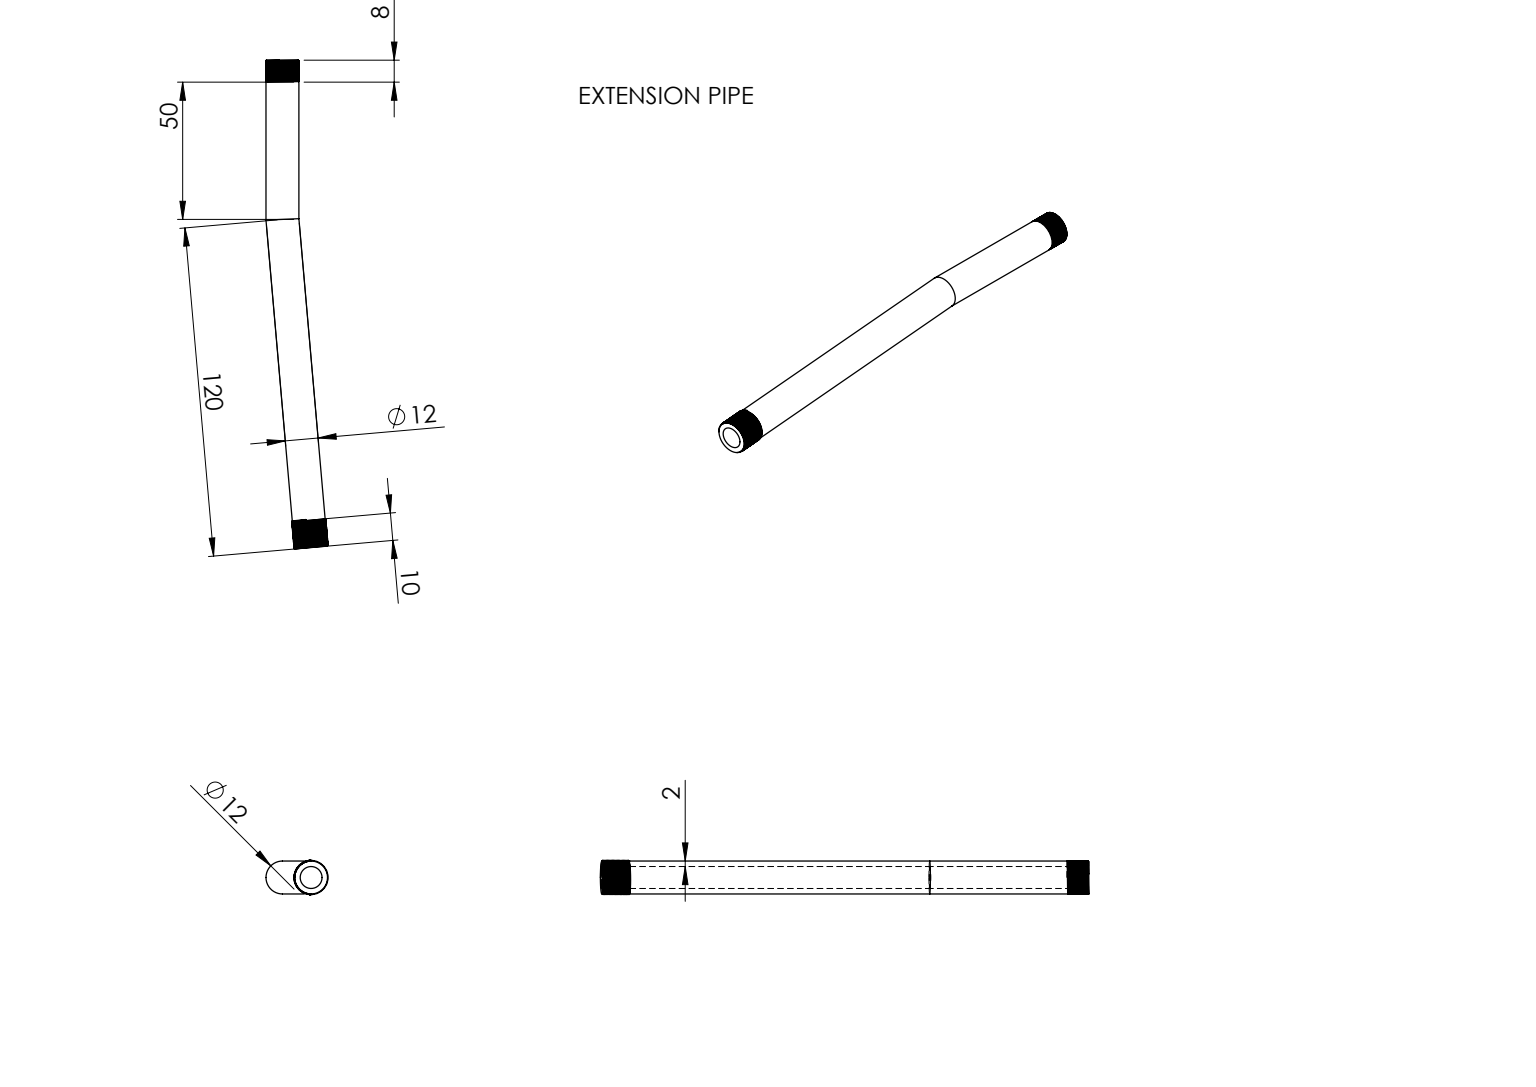
ISO-10303-21;
HEADER;
FILE_DESCRIPTION (('STEP AP214'),
    '1' );
FILE_NAME ('extension pipe.step',
    '2026-10-31T03:36:27',
    ( '' ),
    ( '' ),
    'SwSTEP 2.0',
    'SolidWorks 2026',
    '' );
FILE_SCHEMA (( 'AUTOMOTIVE_DESIGN' ));
ENDSEC;

DATA;
#1=CARTESIAN_POINT ( 'NONE',  ( 20.99999999999999645, 6.928203230275506996, -4.556249998770971033 ) ) ;
#4=CARTESIAN_POINT ( 'NONE',  ( 28.29077060037018043, 5.407089921784856479, 169.1523531505532674 ) ) ;
#11=CARTESIAN_POINT ( 'NONE',  ( 31.25278368747686741, 6.928203230275514990, 167.1898537967678351 ) ) ;
#19=CARTESIAN_POINT ( 'NONE',  ( 15.24356964375000167, -3.323476615752272600, -8.765624999385490668 ) ) ;
#24=CARTESIAN_POINT ( 'NONE',  ( 24.95044711734591658, -3.604726614523244610, 166.7907448923220954 ) ) ;
#32=CARTESIAN_POINT ( 'NONE',  ( 37.56819361912707222, 7.646167579472015790E-16, 167.7383919071516516 ) ) ;
#33=EDGE_LOOP ( 'NONE', ( #36990, #5292, #11130, #31770 ) ) ;
#35=CARTESIAN_POINT ( 'NONE',  ( 23.99999999999999645, 5.196152422706631135, -0.5437499987709648597 ) ) ;
#41=ORIENTED_EDGE ( 'NONE', *, *, #17124, .T. ) ;
#45=CARTESIAN_POINT ( 'NONE',  ( 31.45868912971818432, 0.000000000000000000, 169.5433637710095809 ) ) ;
#46=CARTESIAN_POINT ( 'NONE',  ( 37.19073179189800271, 7.347880794884117764E-16, 166.2186317273649934 ) ) ;
#58=CARTESIAN_POINT ( 'NONE',  ( 24.36378002397578868, 0.000000000000000000, 160.0851093307920223 ) ) ;
#59=CARTESIAN_POINT ( 'NONE',  ( 26.75643035624999655, 3.323476615752271712, -1.340624999385481075 ) ) ;
#64=ORIENTED_EDGE ( 'NONE', *, *, #31239, .F. ) ;
#66=CARTESIAN_POINT ( 'NONE',  ( 18.00000000000000355, -5.196152422706632912, -7.518749998770946519 ) ) ;
#67=CARTESIAN_POINT ( 'NONE',  ( 23.87821517812499650, 4.985214923628404904, -6.140624999385474680 ) ) ;
#75=CARTESIAN_POINT ( 'NONE',  ( 33.73804336749152810, 5.196152422706631135, 161.1753621882693892 ) ) ;
#80=CARTESIAN_POINT ( 'NONE',  ( 23.87821517812499650, 4.985214923628404904, -5.353124999385477700 ) ) ;
#88=EDGE_CURVE ( 'NONE', #32501, #27950, #21194, .T. ) ;
#91=CARTESIAN_POINT ( 'NONE',  ( 36.93903810116746911, 3.604726614523243278, 160.5471114303018680 ) ) ;
#103=ORIENTED_EDGE ( 'NONE', *, *, #10401, .F. ) ;
#104=CARTESIAN_POINT ( 'NONE',  ( 15.00000000000000000, 3.464101615137752166, -5.437500000000009770 ) ) ;
#106=DIRECTION ( 'NONE',  ( 0.9961946980917462113, 0.000000000000000000, -0.08715574274765118534 ) ) ;
#109=CARTESIAN_POINT ( 'NONE',  ( 31.18169728485186454, -7.209453229046475009, 166.3773324967488918 ) ) ;
#111=DIRECTION ( 'NONE',  ( 1.000000000000000000, 0.000000000000000000, 0.000000000000000000 ) ) ;
#114=ORIENTED_EDGE ( 'NONE', *, *, #15759, .T. ) ;
#119=CARTESIAN_POINT ( 'NONE',  ( 21.00000000000000000, 6.646953231504538984, -7.003124999385472726 ) ) ;
#122=CARTESIAN_POINT ( 'NONE',  ( 31.03707322417642800, -6.928203230275514990, 164.7242719189907803 ) ) ;
#123=CARTESIAN_POINT ( 'NONE',  ( 34.15965927292618431, 5.196152422706637353, 165.9944540390638679 ) ) ;
#126=CARTESIAN_POINT ( 'NONE',  ( 31.34102887711597774, 6.928203230275506996, 168.1985009298100522 ) ) ;
#131=DIRECTION ( 'NONE',  ( 0.9961946980917462113, 0.000000000000000000, -0.08715574274765118534 ) ) ;
#134=( BOUNDED_CURVE ( )  B_SPLINE_CURVE ( 2, ( #28363, #34243, #8285, #7031, #33171, #27292, #31580 ),
 .UNSPECIFIED., .F., .F. ) 
 B_SPLINE_CURVE_WITH_KNOTS ( ( 3, 2, 2, 3 ),
 ( 0.2826086956521732252, 0.2898550724637675158, 0.2971014492753617509, 0.3043478260869560414 ),
 .UNSPECIFIED. ) 
 CURVE ( )  GEOMETRIC_REPRESENTATION_ITEM ( )  RATIONAL_B_SPLINE_CURVE ( ( 1.000000000000012212, 0.8660254037844263841, 1.000000000000000000, 0.8660254037844387076, 1.000000000000000000, 0.8660254037844479225, 0.9999999999999907851 ) ) 
 REPRESENTATION_ITEM ( '' )  );
#139=CARTESIAN_POINT ( 'NONE',  ( 26.40304527788004663, 2.021082040740327379, -8.000000000000000000 ) ) ;
#140=CARTESIAN_POINT ( 'NONE',  ( 37.59924285248093412, -3.604726614523238837, 168.0932862683468443 ) ) ;
#141=CARTESIAN_POINT ( 'NONE',  ( 15.00000000000000178, -3.464101615137757051, -1.256249998770949228 ) ) ;
#150=CARTESIAN_POINT ( 'NONE',  ( 36.93740393099094632, -3.604726614523235284, 160.5284327797126025 ) ) ;
#151=CARTESIAN_POINT ( 'NONE',  ( 15.24356964374999990, 3.323476615752268604, -7.378124999385474503 ) ) ;
#153=CARTESIAN_POINT ( 'NONE',  ( 24.98313052087628350, 3.604726614523240613, 167.1643179041065252 ) ) ;
#154=CARTESIAN_POINT ( 'NONE',  ( 34.06814574304114984, -5.196152422706635576, 164.9484496060674985 ) ) ;
#161=EDGE_LOOP ( 'NONE', ( #20979, #30282, #30052, #34984, #7724, #7445, #15889, #35352 ) ) ;
#167=AXIS2_PLACEMENT_3D ( 'NONE', #4303, #33308, #24772 ) ;
#168=CARTESIAN_POINT ( 'NONE',  ( 26.75643035624999655, 3.323476615752271712, -3.140624999385464022 ) ) ;
#182=CARTESIAN_POINT ( 'NONE',  ( 21.00000000000016342, 4.000000000000002665, 50.00000000000000000 ) ) ;
#188=CARTESIAN_POINT ( 'NONE',  ( 30.87038786627866216, 6.928203230275506996, 162.8190495601146495 ) ) ;
#191=FACE_OUTER_BOUND ( 'NONE', #37346, .T. ) ;
#193=CARTESIAN_POINT ( 'NONE',  ( 15.24356964375000167, -3.323476615752272600, -1.453124999385472016 ) ) ;
#209=CARTESIAN_POINT ( 'NONE',  ( 19.00081571707366379, 5.492723647597353320, -10.23957781181608517 ) ) ;
#215=CARTESIAN_POINT ( 'NONE',  ( 25.06483902970220967, 0.000000000000000000, 168.0982504335675287 ) ) ;
#230=AXIS2_PLACEMENT_3D ( 'NONE', #7909, #4677, #5414 ) ;
#236=LINE ( 'NONE', #19612, #23826 ) ;
#242=CARTESIAN_POINT ( 'NONE',  ( 24.81477950914817754, 0.000000000000000000, 162.4454087870936121 ) ) ;
#243=ORIENTED_EDGE ( 'NONE', *, *, #7163, .F. ) ;
#249=CARTESIAN_POINT ( 'NONE',  ( 26.75643035624999655, 3.323476615752271712, -2.240624999385472549 ) ) ;
#252=ORIENTED_EDGE ( 'NONE', *, *, #5826, .F. ) ;
#255=CARTESIAN_POINT ( 'NONE',  ( 15.24356964374999990, 3.323476615752268604, -4.678124999385468108 ) ) ;
#260=EDGE_CURVE ( 'NONE', #23273, #19908, #35667, .T. ) ;
#264=CARTESIAN_POINT ( 'NONE',  ( 27.81970530529572372, -5.196152422706632912, 162.3707280659671994 ) ) ;
#268=CARTESIAN_POINT ( 'NONE',  ( 26.75643035624999655, 7.049594010296217766E-16, -4.978124999385491023 ) ) ;
#269=CARTESIAN_POINT ( 'NONE',  ( 24.00000000000000000, -5.196152422706629359, -1.650000000000012568 ) ) ;
#276=CARTESIAN_POINT ( 'NONE',  ( 33.95006120609467359, 5.407089921784862696, 162.2014130487530110 ) ) ;
#280=CARTESIAN_POINT ( 'NONE',  ( 24.71019261795870037, -3.464101615138094559, 161.2499751506078383 ) ) ;
#288=ORIENTED_EDGE ( 'NONE', *, *, #7515, .F. ) ;
#289=CARTESIAN_POINT ( 'NONE',  ( 15.00000000000000000, 3.464101615137752166, -3.637499999999994849 ) ) ;
#290=CARTESIAN_POINT ( 'NONE',  ( 34.18580599575048495, -5.196152422706635576, 166.2933124484913492 ) ) ;
#293=CARTESIAN_POINT ( 'NONE',  ( 34.37331128181295270, -5.407089921784855591, 167.0391835513610488 ) ) ;
#298=ORIENTED_EDGE ( 'NONE', *, *, #35567, .F. ) ;
#300=CARTESIAN_POINT ( 'NONE',  ( 24.61867908796596183, 0.000000000000000000, 160.2039707163872038 ) ) ;
#303=CARTESIAN_POINT ( 'NONE',  ( 15.24356964374999990, 3.323476615752268604, -6.028124999385455318 ) ) ;
#308=DIRECTION ( 'NONE',  ( 0.000000000000000000, 0.000000000000000000, 1.000000000000000000 ) ) ;
#309=CARTESIAN_POINT ( 'NONE',  ( 28.35571312319377313, 5.196152422706630247, 168.4973254592314618 ) ) ;
#314=( BOUNDED_CURVE ( )  B_SPLINE_CURVE ( 2, ( #13110, #21469, #7242, #4198, #30360, #25227, #30737 ),
 .UNSPECIFIED., .F., .F. ) 
 B_SPLINE_CURVE_WITH_KNOTS ( ( 3, 2, 2, 3 ),
 ( 0.5000000000000013323, 0.5072463768115947902, 0.5144927536231880261, 0.5217391304347814840 ),
 .UNSPECIFIED. ) 
 CURVE ( )  GEOMETRIC_REPRESENTATION_ITEM ( )  RATIONAL_B_SPLINE_CURVE ( ( 0.9999999999999753530, 0.8660254037844633546, 1.000000000000000000, 0.8660254037844387076, 1.000000000000000000, 0.8660254037844592467, 0.9999999999999794609 ) ) 
 REPRESENTATION_ITEM ( '' )  );
#323=CARTESIAN_POINT ( 'NONE',  ( 21.00000000000016342, -4.000000000000002665, 50.00000000000000000 ) ) ;
#324=CARTESIAN_POINT ( 'NONE',  ( 37.56655944895057075, 3.604726614523243278, 167.7197132565624713 ) ) ;
#325=CARTESIAN_POINT ( 'NONE',  ( 21.00000000000000000, 6.928203230275506996, -1.406249998770969123 ) ) ;
#330=FACE_OUTER_BOUND ( 'NONE', #17009, .T. ) ;
#335=EDGE_LOOP ( 'NONE', ( #19344, #12527, #16125, #26950 ) ) ;
#336=CARTESIAN_POINT ( 'NONE',  ( 24.36378002397578868, 0.000000000000000000, 160.0851093307920223 ) ) ;
#338=CARTESIAN_POINT ( 'NONE',  ( 26.75643035624999655, -3.323476615752267715, -8.053124999385453009 ) ) ;
#340=CARTESIAN_POINT ( 'NONE',  ( 37.21031035046954116, 7.646167579472024665E-16, 163.6477674281124450 ) ) ;
#341=CARTESIAN_POINT ( 'NONE',  ( 25.01414827068343172, -3.464101615137761048, 164.7242041589784947 ) ) ;
#348=ORIENTED_EDGE ( 'NONE', *, *, #4481, .T. ) ;
#352=EDGE_CURVE ( 'NONE', #13050, #23173, #13433, .T. ) ;
#354=CARTESIAN_POINT ( 'NONE',  ( 18.12178482187500350, -4.985214923628407568, -4.678124999385496530 ) ) ;
#377=ORIENTED_EDGE ( 'NONE', *, *, #18191, .T. ) ;
#378=CARTESIAN_POINT ( 'NONE',  ( 37.64336544724692146, -3.604726614523235284, 168.5976098342557918 ) ) ;
#380=CARTESIAN_POINT ( 'NONE',  ( 26.75643035624999655, 7.049594010296217766E-16, -1.265624999385456251 ) ) ;
#392=CARTESIAN_POINT ( 'NONE',  ( 18.12178482187499640, 4.985214923628404904, -8.428124999385472549 ) ) ;
#399=CARTESIAN_POINT ( 'NONE',  ( 28.05054758442196672, 5.407089921784862696, 166.4065915139379115 ) ) ;
#402=DIRECTION ( 'NONE',  ( 0.9961946980917462113, 0.000000000000000000, -0.08715574274765118534 ) ) ;
#407=VERTEX_POINT ( 'NONE', #11887 ) ;
#416=ORIENTED_EDGE ( 'NONE', *, *, #28626, .T. ) ;
#424=CARTESIAN_POINT ( 'NONE',  ( 25.44883753774445978, 3.464101615137752610, 169.6927252169354290 ) ) ;
#435=CARTESIAN_POINT ( 'NONE',  ( 30.67183618977810156, -7.209453229046475009, 160.5495935129122245 ) ) ;
#436=CARTESIAN_POINT ( 'NONE',  ( 26.75643035624999655, 7.049594010296217766E-16, -3.178124999385495641 ) ) ;
#441=CARTESIAN_POINT ( 'NONE',  ( 26.75643035624999655, -3.323476615752267271, -6.253124999385469174 ) ) ;
#448=CARTESIAN_POINT ( 'NONE',  ( 24.82458453031440726, 0.000000000000000000, 162.5574806918533000 ) ) ;
#452=CARTESIAN_POINT ( 'NONE',  ( 23.87821517812499650, 4.985214923628404904, -6.703124999385495997 ) ) ;
#460=CARTESIAN_POINT ( 'NONE',  ( 20.99999999999999645, 6.928203230275506996, -5.906249998770958243 ) ) ;
#461=CARTESIAN_POINT ( 'NONE',  ( 33.74088742350031822, -5.407089921784861808, 159.8105457733328478 ) ) ;
#470=CARTESIAN_POINT ( 'NONE',  ( 37.03711979530484655, 3.464101615138000856, 164.4628385719782955 ) ) ;
#474=CARTESIAN_POINT ( 'NONE',  ( 18.00000000000000000, 5.196152422706630247, -8.174999999999988276 ) ) ;
#476=CYLINDRICAL_SURFACE ( 'NONE', #30001, 5.999999999999994671 ) ;
#479=CARTESIAN_POINT ( 'NONE',  ( 28.14696362483655889, -5.407089921784859143, 167.5086318987019069 ) ) ;
#484=AXIS2_PLACEMENT_3D ( 'NONE', #11652, #17544, #9193 ) ;
#486=DIRECTION ( 'NONE',  ( 0.000000000000000000, 0.000000000000000000, 1.000000000000000000 ) ) ;
#487=CARTESIAN_POINT ( 'NONE',  ( 26.99999999999999645, 7.347880794884117764E-16, -3.318749998770964549 ) ) ;
#489=CARTESIAN_POINT ( 'NONE',  ( 23.87821517812500005, -4.985214923628404016, -6.290624999385458160 ) ) ;
#492=CARTESIAN_POINT ( 'NONE',  ( 36.99463137071579411, 7.347880794884117764E-16, 163.9771936566585566 ) ) ;
#496=CARTESIAN_POINT ( 'NONE',  ( 25.41615413421409642, -3.464101615137757051, 169.3191522051509992 ) ) ;
#508=CARTESIAN_POINT ( 'NONE',  ( 37.44889919624123564, 3.604726614523243278, 166.3748504141385922 ) ) ;
#509=CARTESIAN_POINT ( 'NONE',  ( 15.00000000000000000, 3.464101615137752166, -2.231249998770934884 ) ) ;
#517=CARTESIAN_POINT ( 'NONE',  ( 24.78536444607796341, 0.000000000000000000, 162.1091930777120069 ) ) ;
#518=ORIENTED_EDGE ( 'NONE', *, *, #17390, .F. ) ;
#519=CARTESIAN_POINT ( 'NONE',  ( 30.61300606342343755, 7.209453229046475009, 159.8771620917002565 ) ) ;
#520=CARTESIAN_POINT ( 'NONE',  ( 26.75643035624999655, 7.049594010296217766E-16, -9.815624999385457627 ) ) ;
#522=CARTESIAN_POINT ( 'NONE',  ( 37.33123894353190764, 3.604726614523243278, 165.0299875717147131 ) ) ;
#523=CARTESIAN_POINT ( 'NONE',  ( 30.89980292934887629, 6.928203230275514990, 163.1552652694962546 ) ) ;
#534=EDGE_CURVE ( 'NONE', #28874, #27232, #3235, .T. ) ;
#535=CARTESIAN_POINT ( 'NONE',  ( 18.12178482187499640, 4.985214923628404904, -4.828124999385480010 ) ) ;
#544=CARTESIAN_POINT ( 'NONE',  ( 31.20375858228842603, -6.928203230275506996, 166.6294942803155550 ) ) ;
#550=CARTESIAN_POINT ( 'NONE',  ( 30.88754665307854097, 7.209453229046475009, 163.0151753906892793 ) ) ;
#554=CARTESIAN_POINT ( 'NONE',  ( 15.00000000000000000, 0.000000000000000000, 0.000000000000000000 ) ) ;
#562=CARTESIAN_POINT ( 'NONE',  ( 37.52570519453759346, -3.604726614523235284, 167.2527469918319412 ) ) ;
#565=CARTESIAN_POINT ( 'NONE',  ( 26.99999999999999645, 7.347880794884117764E-16, -4.668749998770954868 ) ) ;
#574=CARTESIAN_POINT ( 'NONE',  ( 21.00000000000000000, 6.646953231504538984, -1.603124999385459937 ) ) ;
#582=CARTESIAN_POINT ( 'NONE',  ( 27.85444716323975101, 5.407089921784862696, 164.1651534432314747 ) ) ;
#585=CARTESIAN_POINT ( 'NONE',  ( 15.00000000000001954, 11.99999999999999822, 50.26196565745151190 ) ) ;
#588=CARTESIAN_POINT ( 'NONE',  ( 31.04687824534265417, -6.928203230275506996, 164.8363438237504113 ) ) ;
#589=CARTESIAN_POINT ( 'NONE',  ( 27.99008328789078703, -5.407089921784859143, 165.7154814421367348 ) ) ;
#590=VERTEX_POINT ( 'NONE', #13390 ) ;
#594=EDGE_CURVE ( 'NONE', #25471, #14391, #18768, .T. ) ;
#596=LINE ( 'NONE', #9710, #21812 ) ;
#608=CARTESIAN_POINT ( 'NONE',  ( 20.99999999999999645, 0.000000000000000000, -8.000000000000000000 ) ) ;
#611=CARTESIAN_POINT ( 'NONE',  ( 26.99999999999999645, 7.347880794884117764E-16, -4.668749998770954868 ) ) ;
#617=CARTESIAN_POINT ( 'NONE',  ( 29.49486714975617474, 6.148716665048038266, 159.5363409456820136 ) ) ;
#619=CARTESIAN_POINT ( 'NONE',  ( 26.75643035624999655, -3.323476615752267715, -2.315624999385466509 ) ) ;
#623=VECTOR ( 'NONE', #32641, 1000.000000000000000 ) ;
#624=ORIENTED_EDGE ( 'NONE', *, *, #36236, .T. ) ;
#625=CARTESIAN_POINT ( 'NONE',  ( 26.75643035624999655, -3.323476615752267271, -4.003124999385458516 ) ) ;
#626=CARTESIAN_POINT ( 'NONE',  ( 24.65463083184878101, 3.464101615137419543, 160.6149010293500510 ) ) ;
#629=EDGE_CURVE ( 'NONE', #9403, #23945, #16100, .T. ) ;
#633=CARTESIAN_POINT ( 'NONE',  ( 36.68087069682425039, 7.347880794884117764E-16, 160.3908927435282692 ) ) ;
#638=CARTESIAN_POINT ( 'NONE',  ( 15.24356964374999990, 0.000000000000000000, -6.553124999385484983 ) ) ;
#646=CARTESIAN_POINT ( 'NONE',  ( 36.81810950810510974, 7.646167579472024665E-16, 159.1648912866995715 ) ) ;
#658=CARTESIAN_POINT ( 'NONE',  ( 18.00000000000000355, -5.196152422706632912, -8.025000000000003908 ) ) ;
#662=CARTESIAN_POINT ( 'NONE',  ( 37.41458162253433528, 3.604726614523238837, 165.9825987517649253 ) ) ;
#664=EDGE_CURVE ( 'NONE', #25295, #10376, #15092, .T. ) ;
#671=CARTESIAN_POINT ( 'NONE',  ( 15.00000000000063771, -3.464101615138124757, -3.506249998770952558 ) ) ;
#673=CARTESIAN_POINT ( 'NONE',  ( 21.00000000000000000, 6.646953231504538984, -5.203124999385457805 ) ) ;
#678=CARTESIAN_POINT ( 'NONE',  ( 28.18902776508177510, 5.196152422706636465, 166.5921030979066586 ) ) ;
#681=FACE_OUTER_BOUND ( 'NONE', #22092, .T. ) ;
#682=CARTESIAN_POINT ( 'NONE',  ( 28.43415329166666083, 5.196152422706630247, 169.3939006875140194 ) ) ;
#687=CARTESIAN_POINT ( 'NONE',  ( 20.99999999999999645, -6.646953231504538984, -0.5906249993854775227 ) ) ;
#694=CARTESIAN_POINT ( 'NONE',  ( 37.06326651802246630, 7.347880794884125653E-16, 164.7616969801814548 ) ) ;
#695=CARTESIAN_POINT ( 'NONE',  ( 28.06362094583411704, -5.407089921784865361, 166.5560207186516664 ) ) ;
#703=CARTESIAN_POINT ( 'NONE',  ( 36.95867962683190910, 3.464101615138031054, 163.5662633436957663 ) ) ;
#706=CARTESIAN_POINT ( 'NONE',  ( 27.54558899987776144, 5.407089921784856479, 160.6348884818688418 ) ) ;
#708=CARTESIAN_POINT ( 'NONE',  ( 21.00000000000000000, 6.928203230275506996, -0.5624999999999866773 ) ) ;
#710=CARTESIAN_POINT ( 'NONE',  ( 30.98069435314010178, -7.209453229046482114, 164.0798584742748290 ) ) ;
#711=CARTESIAN_POINT ( 'NONE',  ( 31.03707322417642800, -6.928203230275514990, 164.7242719189907518 ) ) ;
#712=CARTESIAN_POINT ( 'NONE',  ( 25.17756528844239483, 0.000000000000000000, 166.5920692191248804 ) ) ;
#721=CARTESIAN_POINT ( 'NONE',  ( 26.75643035624999655, 7.049594010296217766E-16, -4.528124999385485516 ) ) ;
#733=( BOUNDED_CURVE ( )  B_SPLINE_CURVE ( 2, ( #32456, #15221, #12753, #23751, #29425, #29803, #21299 ),
 .UNSPECIFIED., .F., .F. ) 
 B_SPLINE_CURVE_WITH_KNOTS ( ( 3, 2, 2, 3 ),
 ( 0.6956521739130425708, 0.7028985507246365838, 0.7101449275362307079, 0.7173913043478246099 ),
 .UNSPECIFIED. ) 
 CURVE ( )  GEOMETRIC_REPRESENTATION_ITEM ( )  RATIONAL_B_SPLINE_CURVE ( ( 1.000000000000016431, 0.8660254037844222763, 1.000000000000000000, 0.8660254037844387076, 1.000000000000000000, 0.8660254037844653530, 0.9999999999999733546 ) ) 
 REPRESENTATION_ITEM ( '' )  );
#738=CARTESIAN_POINT ( 'NONE',  ( 30.90715669519676467, -7.209453229046475009, 163.2393191977598974 ) ) ;
#750=ORIENTED_EDGE ( 'NONE', *, *, #22577, .F. ) ;
#751=EDGE_CURVE ( 'NONE', #37490, #27706, #21564, .T. ) ;
#752=CARTESIAN_POINT ( 'NONE',  ( 28.14696362483655889, -5.407089921784859143, 167.5086318987019069 ) ) ;
#753=CARTESIAN_POINT ( 'NONE',  ( 21.00000000000000000, -6.646953231504538984, -3.628124999385489158 ) ) ;
#755=CARTESIAN_POINT ( 'NONE',  ( 15.02283181144952628, 7.347880794884122694E-16, 50.52293445648592751 ) ) ;
#757=CARTESIAN_POINT ( 'NONE',  ( 20.99999999999999645, -6.928203230275506996, -7.481249998770959309 ) ) ;
#766=CARTESIAN_POINT ( 'NONE',  ( 23.87821517812500005, -4.985214923628404016, -2.240624999385460114 ) ) ;
#768=CARTESIAN_POINT ( 'NONE',  ( 15.00000000000000178, -3.464101615137757051, -6.206249998770966059 ) ) ;
#769=DIRECTION ( 'NONE',  ( 0.000000000000000000, 0.000000000000000000, 1.000000000000000000 ) ) ;
#772=VECTOR ( 'NONE', #3527, 1000.000000000000000 ) ;
#773=ORIENTED_EDGE ( 'NONE', *, *, #629, .F. ) ;
#775=CARTESIAN_POINT ( 'NONE',  ( 24.70858993122118363, 3.604726614523240613, 164.0263046051175024 ) ) ;
#782=CARTESIAN_POINT ( 'NONE',  ( 25.03378979634835488, -3.604726614523240613, 167.7433560723723076 ) ) ;
#795=( BOUNDED_CURVE ( )  B_SPLINE_CURVE ( 2, ( #34956, #23784, #32113, #6149, #3492, #15063, #12212 ),
 .UNSPECIFIED., .F., .F. ) 
 B_SPLINE_CURVE_WITH_KNOTS ( ( 3, 2, 2, 3 ),
 ( 0.02173913043478289606, 0.02898550724637719705, 0.03623188405797149458, 0.04347826086956579211 ),
 .UNSPECIFIED. ) 
 CURVE ( )  GEOMETRIC_REPRESENTATION_ITEM ( )  RATIONAL_B_SPLINE_CURVE ( ( 0.9999999999999946709, 0.8660254037844440367, 1.000000000000000000, 0.8660254037844387076, 1.000000000000000000, 0.8660254037844280495, 1.000000000000010658 ) ) 
 REPRESENTATION_ITEM ( '' )  );
#802=CARTESIAN_POINT ( 'NONE',  ( 21.00000000000000355, 0.000000000000000000, 50.00000000000001421 ) ) ;
#804=CARTESIAN_POINT ( 'NONE',  ( 26.99999999999999289, 0.000000000000000000, 49.73803434254939759 ) ) ;
#805=VERTEX_POINT ( 'NONE', #21931 ) ;
#810=CARTESIAN_POINT ( 'NONE',  ( 21.00000000000000000, 6.646953231504538984, -5.765624999385476457 ) ) ;
#816=CARTESIAN_POINT ( 'NONE',  ( 18.12178482187500350, -4.985214923628407568, -5.915624999385471483 ) ) ;
#826=CARTESIAN_POINT ( 'NONE',  ( 30.69389748721465949, -6.928203230275506996, 160.8017552964788592 ) ) ;
#830=CARTESIAN_POINT ( 'NONE',  ( 26.75643035624999655, 3.323476615752271268, -6.290624999385498128 ) ) ;
#834=LINE ( 'NONE', #16009, #19275 ) ;
#838=CARTESIAN_POINT ( 'NONE',  ( 33.81932759197320593, -5.407089921784861808, 160.7071210016154055 ) ) ;
#845=CARTESIAN_POINT ( 'NONE',  ( 25.05990503573306682, 0.000000000000000000, 165.2472063767010013 ) ) ;
#849=ORIENTED_EDGE ( 'NONE', *, *, #1576, .T. ) ;
#850=CARTESIAN_POINT ( 'NONE',  ( 26.99999999999999645, 3.464101615137755275, -7.387499999999980638 ) ) ;
#855=CARTESIAN_POINT ( 'NONE',  ( 31.16208724273364084, 7.209453229046475009, 166.1531886896782737 ) ) ;
#860=ORIENTED_EDGE ( 'NONE', *, *, #32619, .T. ) ;
#865=CARTESIAN_POINT ( 'NONE',  ( 15.24356964374999990, 3.323476615752268604, -6.478124999385451055 ) ) ;
#870=( BOUNDED_CURVE ( )  B_SPLINE_CURVE ( 2, ( #20831, #29529, #6222, #18875, #33264, #1604, #17986 ),
 .UNSPECIFIED., .F., .F. ) 
 B_SPLINE_CURVE_WITH_KNOTS ( ( 3, 2, 2, 3 ),
 ( 0.6304347826086960094, 0.6376811594202902445, 0.6449275362318845906, 0.6521739130434789367 ),
 .UNSPECIFIED. ) 
 CURVE ( )  GEOMETRIC_REPRESENTATION_ITEM ( )  RATIONAL_B_SPLINE_CURVE ( ( 0.9999999999999938938, 0.8660254037844448138, 1.000000000000000000, 0.8660254037844387076, 1.000000000000000000, 0.8660254037844263841, 1.000000000000012212 ) ) 
 REPRESENTATION_ITEM ( '' )  );
#873=CARTESIAN_POINT ( 'NONE',  ( 31.36063891923419789, -6.928203230275506996, 168.4226447368806987 ) ) ;
#886=CARTESIAN_POINT ( 'NONE',  ( 28.14206111430700474, -5.407089921784865361, 167.4525959469342524 ) ) ;
#899=CARTESIAN_POINT ( 'NONE',  ( 33.71964321120555752, 5.407089921784857367, 159.5677233156729642 ) ) ;
#900=CARTESIAN_POINT ( 'NONE',  ( 26.99999999999999645, 3.464101615137755275, -0.6375000000000126121 ) ) ;
#902=CARTESIAN_POINT ( 'NONE',  ( 24.90795869275643426, 0.000000000000000000, 166.3050999770023850 ) ) ;
#903=UNCERTAINTY_MEASURE_WITH_UNIT (LENGTH_MEASURE( 1.000000000000000082E-05 ), #4566, 'distance_accuracy_value', 'NONE');
#904=CARTESIAN_POINT ( 'NONE',  ( 36.98482634954957859, 7.347880794884125653E-16, 163.8651217518988688 ) ) ;
#905=DIRECTION ( 'NONE',  ( 1.000000000000000000, 0.000000000000000000, 0.000000000000000000 ) ) ;
#908=EDGE_CURVE ( 'NONE', #17354, #5563, #28159, .T. ) ;
#911=ORIENTED_EDGE ( 'NONE', *, *, #11960, .F. ) ;
#917=CARTESIAN_POINT ( 'NONE',  ( 21.00000000000000000, 6.646953231504538984, -3.515624999385498217 ) ) ;
#927=FACE_BOUND ( 'NONE', #31912, .T. ) ;
#930=CARTESIAN_POINT ( 'NONE',  ( 37.29692136982500728, 3.604726614523238837, 164.6377359093410746 ) ) ;
#934=PLANE ( 'NONE',  #1221 ) ;
#941=VERTEX_POINT ( 'NONE', #5036 ) ;
#942=CARTESIAN_POINT ( 'NONE',  ( 31.22091736908830839, -7.209453229046475009, 166.8256201108902133 ) ) ;
#943=CARTESIAN_POINT ( 'NONE',  ( 23.87821517812500005, -4.985214923628404016, -2.690624999385465621 ) ) ;
#951=ORIENTED_EDGE ( 'NONE', *, *, #25354, .F. ) ;
#952=VERTEX_POINT ( 'NONE', #16800 ) ;
#955=CARTESIAN_POINT ( 'NONE',  ( 26.75643035624999655, 3.323476615752271712, -2.128124999385482052 ) ) ;
#957=CARTESIAN_POINT ( 'NONE',  ( 26.99999999999999645, 7.347880794884117764E-16, -7.818749998770941012 ) ) ;
#961=ORIENTED_EDGE ( 'NONE', *, *, #8896, .T. ) ;
#964=CARTESIAN_POINT ( 'NONE',  ( 24.75434669616370087, -3.604726614523244610, 164.5493068216156871 ) ) ;
#971=CARTESIAN_POINT ( 'NONE',  ( 31.20130732697009535, 7.209453229046475009, 166.6014763038195383 ) ) ;
#972=VERTEX_POINT ( 'NONE', #11471 ) ;
#977=DIRECTION ( 'NONE',  ( 0.000000000000000000, 0.000000000000000000, 1.000000000000000000 ) ) ;
#986=CARTESIAN_POINT ( 'NONE',  ( 23.99999999999999645, 5.196152422706631135, -1.500000000000001332 ) ) ;
#992=CARTESIAN_POINT ( 'NONE',  ( 25.05663669537974414, 3.464101615137583856, 165.2098490755226123 ) ) ;
#998=CARTESIAN_POINT ( 'NONE',  ( 15.24356964375000167, -3.323476615752272600, -4.715624999385497063 ) ) ;
#1002=CARTESIAN_POINT ( 'NONE',  ( 20.99999999999999645, -6.646953231504538984, -6.778124999385457983 ) ) ;
#1004=VECTOR ( 'NONE', #14540, 1000.000000000000000 ) ;
#1006=EDGE_CURVE ( 'NONE', #5916, #35535, #23839, .T. ) ;
#1009=CARTESIAN_POINT ( 'NONE',  ( 33.60730975337005333, -5.196152422706629359, 159.6810701411317552 ) ) ;
#1014=CARTESIAN_POINT ( 'NONE',  ( 20.99999999999999645, -6.646953231504538984, -7.340624999385477523 ) ) ;
#1015=CARTESIAN_POINT ( 'NONE',  ( 26.99999999999999645, 7.347880794884117764E-16, -2.475000000000004974 ) ) ;
#1019=CARTESIAN_POINT ( 'NONE',  ( 25.48152094116770883, 0.000000000000000000, 170.0662982274954800 ) ) ;
#1024=CARTESIAN_POINT ( 'NONE',  ( 36.85732959234155004, 7.646167579472024665E-16, 159.6131789008408646 ) ) ;
#1032=CARTESIAN_POINT ( 'NONE',  ( 24.99999999999999289, 0.000000000000000000, -8.000000000000000000 ) ) ;
#1038=CARTESIAN_POINT ( 'NONE',  ( 26.99999999999999645, 7.347880794884117764E-16, -6.074999999999997513 ) ) ;
#1042=CARTESIAN_POINT ( 'NONE',  ( 27.82012958953286130, 5.407089921784856479, 163.7729017808578362 ) ) ;
#1043=CARTESIAN_POINT ( 'NONE',  ( 28.42434827050043467, 5.196152422706636465, 169.2818287827543600 ) ) ;
#1051=CARTESIAN_POINT ( 'NONE',  ( 26.75643035624999655, -3.323476615752267715, -7.603124999385488358 ) ) ;
#1058=CARTESIAN_POINT ( 'NONE',  ( 31.24297866652486633, -6.928203230275506996, 167.0777818944568480 ) ) ;
#1070=EDGE_CURVE ( 'NONE', #30479, #30148, #16319, .T. ) ;
#1072=( BOUNDED_CURVE ( )  B_SPLINE_CURVE ( 2, ( #10156, #21731, #27592, #6752, #33281, #24192, #32900 ),
 .UNSPECIFIED., .F., .F. ) 
 B_SPLINE_CURVE_WITH_KNOTS ( ( 3, 2, 2, 3 ),
 ( 0.7173913043478248319, 0.7246376811594191780, 0.7318840579710134131, 0.7391304347826076482 ),
 .UNSPECIFIED. ) 
 CURVE ( )  GEOMETRIC_REPRESENTATION_ITEM ( )  RATIONAL_B_SPLINE_CURVE ( ( 1.000000000000022649, 0.8660254037844161701, 1.000000000000000000, 0.8660254037844387076, 1.000000000000000000, 0.8660254037844571373, 0.9999999999999815703 ) ) 
 REPRESENTATION_ITEM ( '' )  );
#1076=CARTESIAN_POINT ( 'NONE',  ( 37.44236251553515871, -3.604726614523238837, 166.3001358117817006 ) ) ;
#1085=CARTESIAN_POINT ( 'NONE',  ( 15.00000000000000355, 7.347880794884112834E-16, -8.000000000000000000 ) ) ;
#1089=CARTESIAN_POINT ( 'NONE',  ( 24.39973176785919051, 3.604726614523236616, 160.4960396437548695 ) ) ;
#1090=CARTESIAN_POINT ( 'NONE',  ( 21.00000000000000000, -6.646953231504538984, -9.478124999385466154 ) ) ;
#1091=CARTESIAN_POINT ( 'NONE',  ( 25.40961745350799461, 3.464101615137737067, 169.2444376027941360 ) ) ;
#1092=CARTESIAN_POINT ( 'NONE',  ( 24.79356678040014117, -3.604726614523244610, 164.9975944357569517 ) ) ;
#1093=CARTESIAN_POINT ( 'NONE',  ( 36.86389775648721212, -3.464101615137755275, 162.4829016082965438 ) ) ;
#1105=CARTESIAN_POINT ( 'NONE',  ( 15.24356964374999990, 0.000000000000000000, -6.553124999385484983 ) ) ;
#1116=LINE ( 'NONE', #12682, #17619 ) ;
#1120=CARTESIAN_POINT ( 'NONE',  ( 31.08364707426076023, 7.209453229046475009, 165.2566134613956876 ) ) ;
#1130=ORIENTED_EDGE ( 'NONE', *, *, #27910, .F. ) ;
#1131=CARTESIAN_POINT ( 'NONE',  ( 34.37331128181295270, -5.407089921784855591, 167.0391835513610488 ) ) ;
#1132=CARTESIAN_POINT ( 'NONE',  ( 26.75643035624999655, -3.323476615752267715, -3.103124999385467486 ) ) ;
#1133=CARTESIAN_POINT ( 'NONE',  ( 26.78555467025737258, 0.1019468494213565390, -8.000000000000003553 ) ) ;
#1143=CARTESIAN_POINT ( 'NONE',  ( 21.00000000000000000, -6.646953231504538984, -2.728124999385465266 ) ) ;
#1145=EDGE_CURVE ( 'NONE', #13208, #28137, #27709, .T. ) ;
#1146=CARTESIAN_POINT ( 'NONE',  ( 15.00000000000000178, -3.464101615137757051, -8.456249998770944742 ) ) ;
#1153=CARTESIAN_POINT ( 'NONE',  ( 24.74781001545762393, 3.604726614523240613, 164.4745922192587670 ) ) ;
#1158=DIRECTION ( 'NONE',  ( 0.000000000000000000, 0.000000000000000000, 1.000000000000000000 ) ) ;
#1161=CARTESIAN_POINT ( 'NONE',  ( 37.41131328218130392, 7.646167579472015790E-16, 165.9452414505865079 ) ) ;
#1163=CARTESIAN_POINT ( 'NONE',  ( 31.31161381383153142, -6.928203230275514990, 167.8622852179797462 ) ) ;
#1170=VERTEX_POINT ( 'NONE', #12026 ) ;
#1171=( LENGTH_UNIT ( ) NAMED_UNIT ( * ) SI_UNIT ( .MILLI., .METRE. ) );
#1175=CARTESIAN_POINT ( 'NONE',  ( 15.00000000000000000, 0.000000000000000000, -1.349999999999990097 ) ) ;
#1178=CARTESIAN_POINT ( 'NONE',  ( 15.60291623300155095, 2.331604889245508350, -7.999999999999992895 ) ) ;
#1186=CARTESIAN_POINT ( 'NONE',  ( 15.24356964375000167, -3.323476615752272600, -3.815624999385473615 ) ) ;
#1189=CARTESIAN_POINT ( 'NONE',  ( 36.99136303036318196, -3.464101615137506140, 163.9398363554800540 ) ) ;
#1196=CARTESIAN_POINT ( 'NONE',  ( 27.61053152270135058, 5.196152422706630247, 159.9798607905470362 ) ) ;
#1200=CARTESIAN_POINT ( 'NONE',  ( 23.87821517812500005, -4.985214923628404016, -5.953124999385495109 ) ) ;
#1214=CARTESIAN_POINT ( 'NONE',  ( 26.97716818855048260, 0.000000000000000000, 49.47706554351410801 ) ) ;
#1221=AXIS2_PLACEMENT_3D ( 'NONE', #29172, #18014, #26333 ) ;
#1223=CARTESIAN_POINT ( 'NONE',  ( 26.99999999999999289, 0.000000000000000000, -8.000000000000000000 ) ) ;
#1226=CARTESIAN_POINT ( 'NONE',  ( 31.04442699002431993, 7.209453229046475009, 164.8083258472544230 ) ) ;
#1229=VERTEX_POINT ( 'NONE', #1019 ) ;
#1234=DIRECTION ( 'NONE',  ( 0.000000000000000000, 0.000000000000000000, 1.000000000000000000 ) ) ;
#1236=CARTESIAN_POINT ( 'NONE',  ( 25.22171936664797798, 0.000000000000000000, 169.8914008901326724 ) ) ;
#1237=CARTESIAN_POINT ( 'NONE',  ( 21.00000000000000000, 6.646953231504538984, -9.253124999385450522 ) ) ;
#1238=VECTOR ( 'NONE', #13008, 1000.000000000000000 ) ;
#1246=CARTESIAN_POINT ( 'NONE',  ( 31.30180879287953388, 6.928203230275506996, 167.7502133156687876 ) ) ;
#1252=CARTESIAN_POINT ( 'NONE',  ( 15.24356964374999990, 0.000000000000000000, -0.2531249993854844949 ) ) ;
#1260=CARTESIAN_POINT ( 'NONE',  ( 28.02440086159767674, -5.407089921784865361, 166.1077331045103733 ) ) ;
#1269=CARTESIAN_POINT ( 'NONE',  ( 18.00000000000000355, -5.196152422706632912, -7.968749998770952025 ) ) ;
#1275=CARTESIAN_POINT ( 'NONE',  ( 21.00000000000000000, 6.928203230275506996, -0.1124999999999909128 ) ) ;
#1277=CARTESIAN_POINT ( 'NONE',  ( 30.88264414254899393, 7.209453229046482114, 162.9591394389215964 ) ) ;
#1278=CARTESIAN_POINT ( 'NONE',  ( 24.77882776526477571, -3.464101615137761048, 162.0344784741307933 ) ) ;
#1283=ORIENTED_EDGE ( 'NONE', *, *, #15614, .T. ) ;
#1285=ORIENTED_EDGE ( 'NONE', *, *, #5231, .T. ) ;
#1290=CARTESIAN_POINT ( 'NONE',  ( 15.24356964374999990, 0.000000000000000000, -5.653124999385472194 ) ) ;
#1304=EDGE_CURVE ( 'NONE', #17372, #23833, #795, .T. ) ;
#1306=CARTESIAN_POINT ( 'NONE',  ( 37.13677269252619340, 7.646167579472015790E-16, 162.8072281515975135 ) ) ;
#1309=CARTESIAN_POINT ( 'NONE',  ( 14.99999999999945111, -3.464101615137439083, -0.8625000000000012657 ) ) ;
#1311=CARTESIAN_POINT ( 'NONE',  ( 18.00000000000000355, -5.196152422706632912, -5.718749998770950249 ) ) ;
#1313=CARTESIAN_POINT ( 'NONE',  ( 18.00000000000000355, -5.196152422706632912, -4.368749998770960374 ) ) ;
#1319=CARTESIAN_POINT ( 'NONE',  ( 28.21233043189729273, 5.407089921784856479, 168.2557779222707097 ) ) ;
#1320=CARTESIAN_POINT ( 'NONE',  ( 18.12178482187500350, -4.985214923628407568, -3.665624999385469707 ) ) ;
#1324=CARTESIAN_POINT ( 'NONE',  ( 34.27731952563551232, 5.196152422706637353, 167.3393168814877185 ) ) ;
#1335=CARTESIAN_POINT ( 'NONE',  ( 18.12178482187499640, 4.985214923628404904, -0.6656249993854668201 ) ) ;
#1337=CARTESIAN_POINT ( 'NONE',  ( 26.75643035624999655, 7.049594010296217766E-16, -0.4781249993854874702 ) ) ;
#1343=CARTESIAN_POINT ( 'NONE',  ( 24.86547026816695904, 3.604726614523240613, 165.8194550616826461 ) ) ;
#1350=CARTESIAN_POINT ( 'NONE',  ( 25.02725311564228505, 3.604726614523236616, 167.6686414700154444 ) ) ;
#1355=( BOUNDED_CURVE ( )  B_SPLINE_CURVE ( 2, ( #10748, #29951, #25522, #19488, #18598, #33873, #4171 ),
 .UNSPECIFIED., .F., .F. ) 
 B_SPLINE_CURVE_WITH_KNOTS ( ( 3, 2, 2, 3 ),
 ( 0.4782608695652167397, 0.4855072463768107527, 0.4927536231884048767, 0.4999999999999988898 ),
 .UNSPECIFIED. ) 
 CURVE ( )  GEOMETRIC_REPRESENTATION_ITEM ( )  RATIONAL_B_SPLINE_CURVE ( ( 1.000000000000012212, 0.8660254037844263841, 1.000000000000000000, 0.8660254037844387076, 1.000000000000000000, 0.8660254037844592467, 0.9999999999999794609 ) ) 
 REPRESENTATION_ITEM ( '' )  );
#1357=EDGE_CURVE ( 'NONE', #13931, #17802, #834, .T. ) ;
#1359=ADVANCED_FACE ( 'NONE', ( #15816 ), #4428, .T. ) ;
#1368=CARTESIAN_POINT ( 'NONE',  ( 15.00000000000000000, 0.000000000000000000, -2.250000000000001776 ) ) ;
#1370=DIRECTION ( 'NONE',  ( 0.9961946980917462113, 0.000000000000000000, -0.08715574274765118534 ) ) ;
#1372=DIRECTION ( 'NONE',  ( 1.000000000000000000, 0.000000000000000000, 0.000000000000000000 ) ) ;
#1379=CARTESIAN_POINT ( 'NONE',  ( 26.75643035624999655, 3.323476615752271712, -5.390624999385475569 ) ) ;
#1381=ORIENTED_EDGE ( 'NONE', *, *, #20383, .F. ) ;
#1382=CARTESIAN_POINT ( 'NONE',  ( 20.99999999999999645, 6.646953231504538984, -7.003124999385472726 ) ) ;
#1407=CARTESIAN_POINT ( 'NONE',  ( 34.31653960987195973, 5.196152422706637353, 167.7876044956290116 ) ) ;
#1412=ORIENTED_EDGE ( 'NONE', *, *, #35882, .T. ) ;
#1416=CARTESIAN_POINT ( 'NONE',  ( 37.29365302947196881, 7.646167579472015790E-16, 164.6003786081626572 ) ) ;
#1417=CARTESIAN_POINT ( 'NONE',  ( 31.40966402442264283, 6.928203230275514990, 168.9830042533329504 ) ) ;
#1419=ORIENTED_EDGE ( 'NONE', *, *, #11897, .T. ) ;
#1423=CARTESIAN_POINT ( 'NONE',  ( 24.58599568454329543, 3.464101615138089674, 159.8303977058270959 ) ) ;
#1424=CARTESIAN_POINT ( 'NONE',  ( 26.99999999999999289, 0.000000000000000000, -8.000000000000000000 ) ) ;
#1427=CYLINDRICAL_SURFACE ( 'NONE', #12358, 5.999999999999994671 ) ;
#1428=CARTESIAN_POINT ( 'NONE',  ( 23.87821517812500005, -4.985214923628404016, -8.540624999385460825 ) ) ;
#1436=CARTESIAN_POINT ( 'NONE',  ( 25.21351703232580022, 3.464101615137752166, 167.0029995320877276 ) ) ;
#1449=CARTESIAN_POINT ( 'NONE',  ( 27.82830044041545747, -5.407089921784865361, 163.8662950338039650 ) ) ;
#1462=DIRECTION ( 'NONE',  ( 0.08715574274765150453, 0.000000000000000000, 0.9961946980917461003 ) ) ;
#1464=VERTEX_POINT ( 'NONE', #21326 ) ;
#1467=CARTESIAN_POINT ( 'NONE',  ( 21.00000000000000000, -6.928203230275506996, -2.137499999999987743 ) ) ;
#1469=CARTESIAN_POINT ( 'NONE',  ( 33.98928129033111389, 5.407089921784862696, 162.6497006628943041 ) ) ;
#1470=CARTESIAN_POINT ( 'NONE',  ( 36.82794601260381029, 7.347880794884125653E-16, 162.0719712953337250 ) ) ;
#1478=DIRECTION ( 'NONE',  ( 0.9961946980917462113, 0.000000000000000000, -0.08715574274765118534 ) ) ;
#1480=CARTESIAN_POINT ( 'NONE',  ( 23.87821517812499650, 4.985214923628404904, -7.153124999385473970 ) ) ;
#1493=CARTESIAN_POINT ( 'NONE',  ( 30.82871652672388052, -7.209453229046475009, 162.3427439694773398 ) ) ;
#1503=ORIENTED_EDGE ( 'NONE', *, *, #11731, .F. ) ;
#1504=CARTESIAN_POINT ( 'NONE',  ( 24.87690945940258302, -3.604726614523240613, 165.9502056158071355 ) ) ;
#1505=CARTESIAN_POINT ( 'NONE',  ( 18.12178482187500350, -4.985214923628407568, -4.565624999385481608 ) ) ;
#1506=EDGE_CURVE ( 'NONE', #23173, #20504, #20187, .T. ) ;
#1508=AXIS2_PLACEMENT_3D ( 'NONE', #13039, #30663, #33125 ) ;
#1514=ORIENTED_EDGE ( 'NONE', *, *, #4696, .F. ) ;
#1518=CARTESIAN_POINT ( 'NONE',  ( 21.00000000000000000, -6.646953231504538984, -3.628124999385489158 ) ) ;
#1521=CARTESIAN_POINT ( 'NONE',  ( 26.99999999999999645, 7.347880794884117764E-16, -9.168749998770959309 ) ) ;
#1528=CARTESIAN_POINT ( 'NONE',  ( 36.97172150469783958, -3.604726614523238837, 160.9206844420862694 ) ) ;
#1531=SURFACE_SIDE_STYLE ('',( #14174 ) ) ;
#1538=VECTOR ( 'NONE', #3418, 1000.000000000000000 ) ;
#1539=( BOUNDED_CURVE ( )  B_SPLINE_CURVE ( 2, ( #31113, #8365, #19564, #1, #19936, #11568, #23141 ),
 .UNSPECIFIED., .F., .F. ) 
 B_SPLINE_CURVE_WITH_KNOTS ( ( 3, 2, 2, 3 ),
 ( 0.3913043478260868069, 0.3985507246376810975, 0.4057971014492754436, 0.4130434782608697342 ),
 .UNSPECIFIED. ) 
 CURVE ( )  GEOMETRIC_REPRESENTATION_ITEM ( )  RATIONAL_B_SPLINE_CURVE ( ( 1.000000000000003109, 0.8660254037844357100, 1.000000000000000000, 0.8660254037844387076, 1.000000000000000000, 0.8660254037844355990, 1.000000000000003109 ) ) 
 REPRESENTATION_ITEM ( '' )  );
#1544=CARTESIAN_POINT ( 'NONE',  ( 27.00000000000003908, -3.464101615137728185, -2.456249998770948295 ) ) ;
#1555=LINE ( 'NONE', #16722, #15004 ) ;
#1556=FACE_OUTER_BOUND ( 'NONE', #35166, .T. ) ;
#1558=ORIENTED_EDGE ( 'NONE', *, *, #594, .T. ) ;
#1563=CARTESIAN_POINT ( 'NONE',  ( 18.12178482187499640, 4.985214923628404904, -5.278124999385486404 ) ) ;
#1566=EDGE_CURVE ( 'NONE', #3429, #35216, #33057, .T. ) ;
#1569=CARTESIAN_POINT ( 'NONE',  ( 23.87821517812499650, 4.985214923628404904, -7.040624999385459049 ) ) ;
#1573=( BOUNDED_CURVE ( )  B_SPLINE_CURVE ( 2, ( #20156, #25464, #8226, #17130, #28666, #34364, #31705 ),
 .UNSPECIFIED., .F., .F. ) 
 B_SPLINE_CURVE_WITH_KNOTS ( ( 3, 2, 2, 3 ),
 ( 0.6086956521739121939, 0.6159420289855062070, 0.6231884057971003310, 0.6304347826086944551 ),
 .UNSPECIFIED. ) 
 CURVE ( )  GEOMETRIC_REPRESENTATION_ITEM ( )  RATIONAL_B_SPLINE_CURVE ( ( 1.000000000000016431, 0.8660254037844222763, 1.000000000000000000, 0.8660254037844387076, 1.000000000000000000, 0.8660254037844612451, 0.9999999999999774625 ) ) 
 REPRESENTATION_ITEM ( '' )  );
#1574=AXIS2_PLACEMENT_3D ( 'NONE', #26100, #8857, #131 ) ;
#1576=EDGE_CURVE ( 'NONE', #14024, #22269, #24528, .T. ) ;
#1581=CARTESIAN_POINT ( 'NONE',  ( 27.81970530529572372, -5.196152422706632912, 162.3707280659671994 ) ) ;
#1584=CARTESIAN_POINT ( 'NONE',  ( 24.00000000000000000, -5.196152422706629359, -7.950000000000012612 ) ) ;
#1591=ORIENTED_EDGE ( 'NONE', *, *, #30400, .T. ) ;
#1602=EDGE_LOOP ( 'NONE', ( #5890, #19433, #27846, #21433 ) ) ;
#1603=DIRECTION ( 'NONE',  ( 0.000000000000000000, 0.000000000000000000, 1.000000000000000000 ) ) ;
#1604=CARTESIAN_POINT ( 'NONE',  ( 14.99999999999968203, -3.464101615137573198, -7.106249998770961973 ) ) ;
#1607=CARTESIAN_POINT ( 'NONE',  ( 24.75598086634022010, 0.000000000000000000, 164.5679854722048958 ) ) ;
#1610=VERTEX_POINT ( 'NONE', #12971 ) ;
#1612=ORIENTED_EDGE ( 'NONE', *, *, #18908, .T. ) ;
#1614=CARTESIAN_POINT ( 'NONE',  ( 21.00000000000000000, -6.928203230275506996, -5.231249998770948650 ) ) ;
#1615=CARTESIAN_POINT ( 'NONE',  ( 15.24356964374999990, 0.000000000000000000, -1.040624999385481031 ) ) ;
#1618=CARTESIAN_POINT ( 'NONE',  ( 26.75643035624999655, 3.323476615752271712, -9.328124999385446259 ) ) ;
#1626=CARTESIAN_POINT ( 'NONE',  ( 25.18083362879543685, -3.464101615137757051, 166.6294265203033262 ) ) ;
#1632=CARTESIAN_POINT ( 'NONE',  ( 20.99999999999999645, 6.646953231504538984, -1.715624999385482852 ) ) ;
#1636=AXIS2_PLACEMENT_3D ( 'NONE', #17636, #21747, #29554 ) ;
#1638=CARTESIAN_POINT ( 'NONE',  ( 28.25112623189659544, -5.196152422706632912, 167.3018918215213660 ) ) ;
#1642=CARTESIAN_POINT ( 'NONE',  ( 37.32470226282583781, -3.604726614523238837, 164.9552729693578215 ) ) ;
#1647=CARTESIAN_POINT ( 'NONE',  ( 15.00000000000034461, -3.464101615137956003, -3.562499999999996447 ) ) ;
#1651=CARTESIAN_POINT ( 'NONE',  ( 16.07192114941521766, -3.422577806627481234, -8.000000000000001776 ) ) ;
#1657=CARTESIAN_POINT ( 'NONE',  ( 18.00000000000000000, 5.196152422706630247, -3.225000000000005862 ) ) ;
#1658=CARTESIAN_POINT ( 'NONE',  ( 24.71512661192725702, -3.604726614523244610, 164.1010192074743941 ) ) ;
#1659=CARTESIAN_POINT ( 'NONE',  ( 33.68901826208886519, 5.196152422706637353, 160.6150026693684367 ) ) ;
#1670=CARTESIAN_POINT ( 'NONE',  ( 21.00000000000000000, 6.646953231504538984, -7.565624999385492266 ) ) ;
#1673=CARTESIAN_POINT ( 'NONE',  ( 31.44888410865908668, 6.928203230275514990, 169.4312918674742434 ) ) ;
#1681=DIRECTION ( 'NONE',  ( -0.000000000000000000, -0.000000000000000000, -1.000000000000000000 ) ) ;
#1682=CARTESIAN_POINT ( 'NONE',  ( 33.83730346391489263, 5.407089921784857367, 160.9125861580968149 ) ) ;
#1691=CARTESIAN_POINT ( 'NONE',  ( 34.15106413780644345, 5.407089921784857367, 164.4988870712271023 ) ) ;
#1693=CARTESIAN_POINT ( 'NONE',  ( 15.24356964374999990, 0.000000000000000000, -4.640624999385472904 ) ) ;
#1698=CARTESIAN_POINT ( 'NONE',  ( 15.00000000000000355, 7.347880794884112834E-16, -8.000000000000000000 ) ) ;
#1702=ORIENTED_EDGE ( 'NONE', *, *, #27762, .F. ) ;
#1706=CARTESIAN_POINT ( 'NONE',  ( 21.00000000000000000, 6.646953231504538984, -4.753124999385462068 ) ) ;
#1709=CARTESIAN_POINT ( 'NONE',  ( 21.00000000000000000, 6.928203230275506996, -9.506249998770956111 ) ) ;
#1713=ORIENTED_EDGE ( 'NONE', *, *, #10791, .T. ) ;
#1717=CARTESIAN_POINT ( 'NONE',  ( 30.82381401619432637, -7.209453229046482114, 162.2867080177096852 ) ) ;
#1718=ADVANCED_FACE ( 'NONE', ( #28616 ), #14601, .T. ) ;
#1728=DIRECTION ( 'NONE',  ( 0.08715574274765150453, 0.000000000000000000, 0.9961946980917461003 ) ) ;
#1736=CARTESIAN_POINT ( 'NONE',  ( 15.02283181144952628, 7.347880794884122694E-16, 50.52293445648592751 ) ) ;
#1747=CARTESIAN_POINT ( 'NONE',  ( 15.00000000000000178, -3.464101615137757051, -6.712500000000003020 ) ) ;
#1751=EDGE_CURVE ( 'NONE', #24079, #15328, #5891, .T. ) ;
#1754=CARTESIAN_POINT ( 'NONE',  ( 21.00000000000000000, 6.646953231504538984, -7.565624999385492266 ) ) ;
#1757=CARTESIAN_POINT ( 'NONE',  ( 23.87821517812499650, 4.985214923628404904, -7.490624999385464555 ) ) ;
#1760=CARTESIAN_POINT ( 'NONE',  ( 37.64499961742345135, 3.604726614523243278, 168.6162884848450005 ) ) ;
#1763=ADVANCED_FACE ( 'NONE', ( #26334 ), #19416, .T. ) ;
#1764=CARTESIAN_POINT ( 'NONE',  ( 27.00000000000052580, -3.464101615137444412, -7.462499999999999467 ) ) ;
#1768=CYLINDRICAL_SURFACE ( 'NONE', #5822, 5.999999999999994671 ) ;
#1777=CYLINDRICAL_SURFACE ( 'NONE', #7695, 5.999999999999994671 ) ;
#1778=ORIENTED_EDGE ( 'NONE', *, *, #29074, .T. ) ;
#1794=CARTESIAN_POINT ( 'NONE',  ( 34.05955060792140188, -5.407089921784855591, 163.4528826382307614 ) ) ;
#1795=DIRECTION ( 'NONE',  ( 0.000000000000000000, 0.000000000000000000, 1.000000000000000000 ) ) ;
#1799=ORIENTED_EDGE ( 'NONE', *, *, #664, .T. ) ;
#1800=ORIENTED_EDGE ( 'NONE', *, *, #8770, .F. ) ;
#1801=CARTESIAN_POINT ( 'NONE',  ( 26.99999999999999645, 7.347880794884117764E-16, -6.018749998770944742 ) ) ;
#1804=DIRECTION ( 'NONE',  ( 0.9961946980917462113, 0.000000000000000000, -0.08715574274765118534 ) ) ;
#1805=CARTESIAN_POINT ( 'NONE',  ( 15.24356964375000167, -3.323476615752272600, -9.103124999385496352 ) ) ;
#1812=CARTESIAN_POINT ( 'NONE',  ( 25.25600545691528254, 0.000000000000000000, 167.4886444474074381 ) ) ;
#1816=CARTESIAN_POINT ( 'NONE',  ( 26.75643035624999655, -3.323476615752267271, -0.9656249993854794100 ) ) ;
#1824=CARTESIAN_POINT ( 'NONE',  ( 34.09102412561951212, 5.196152422706631135, 165.2099507155409412 ) ) ;
#1825=CARTESIAN_POINT ( 'NONE',  ( 34.06772145880400160, 5.407089921784862696, 163.5462758911768617 ) ) ;
#1832=CARTESIAN_POINT ( 'NONE',  ( 37.07307153918868181, 7.347880794884117764E-16, 164.8737688849411143 ) ) ;
#1834=CARTESIAN_POINT ( 'NONE',  ( 30.72331255028488428, -6.928203230275514990, 161.1379710058604644 ) ) ;
#1836=CARTESIAN_POINT ( 'NONE',  ( 27.00000000000052580, -3.464101615137444412, -7.856249998770953979 ) ) ;
#1842=CARTESIAN_POINT ( 'NONE',  ( 18.00000000000000355, -5.196152422706632912, -2.175000000000010481 ) ) ;
#1843=CARTESIAN_POINT ( 'NONE',  ( 27.74986027194257332, -5.407089921784865361, 162.9697198055213789 ) ) ;
#1844=CARTESIAN_POINT ( 'NONE',  ( 30.84097280299421229, -6.928203230275514990, 162.4828338482843151 ) ) ;
#1855=CARTESIAN_POINT ( 'NONE',  ( 23.87821517812500005, -4.985214923628404016, -9.553124999385486760 ) ) ;
#1858=DIRECTION ( 'NONE',  ( 0.08715574274765150453, 0.000000000000000000, 0.9961946980917461003 ) ) ;
#1868=CARTESIAN_POINT ( 'NONE',  ( 33.87652354815133293, 5.407089921784857367, 161.3608737722381079 ) ) ;
#1869=CARTESIAN_POINT ( 'NONE',  ( 37.15151170766156952, 7.347880794884117764E-16, 165.7703441132237003 ) ) ;
#1871=CARTESIAN_POINT ( 'NONE',  ( 36.59262550718515428, 7.347880794884125653E-16, 159.3822456104860237 ) ) ;
#1876=CYLINDRICAL_SURFACE ( 'NONE', #25136, 5.999999999999994671 ) ;
#1878=AXIS2_PLACEMENT_3D ( 'NONE', #9654, #26702, #23684 ) ;
#1880=CARTESIAN_POINT ( 'NONE',  ( 37.17272443640960233, -3.604726614523235284, 163.2181584645603323 ) ) ;
#1881=CARTESIAN_POINT ( 'NONE',  ( 23.87821517812499650, 4.985214923628404904, -5.240624999385462779 ) ) ;
#1884=CARTESIAN_POINT ( 'NONE',  ( 37.33453876732453125, -3.464101615137755275, 167.8623529779920034 ) ) ;
#1887=CARTESIAN_POINT ( 'NONE',  ( 29.49323130461320730, 6.148716367659644355, 159.5176625013623095 ) ) ;
#1891=ORIENTED_EDGE ( 'NONE', *, *, #7343, .F. ) ;
#1894=CARTESIAN_POINT ( 'NONE',  ( 15.24356964374999990, 3.323476615752268604, -2.878124999385485161 ) ) ;
#1897=CARTESIAN_POINT ( 'NONE',  ( 24.00000000000000000, -5.196152422706629359, -10.14374999877096251 ) ) ;
#1898=EDGE_CURVE ( 'NONE', #29577, #4196, #33243, .T. ) ;
#1918=ORIENTED_EDGE ( 'NONE', *, *, #4718, .F. ) ;
#1929=CARTESIAN_POINT ( 'NONE',  ( 34.14658591151403755, -5.196152422706635576, 165.8450248343500562 ) ) ;
#1931=VECTOR ( 'NONE', #2756, 1000.000000000000000 ) ;
#1936=CARTESIAN_POINT ( 'NONE',  ( 26.75643035624999655, -3.323476615752267715, -7.715624999385478411 ) ) ;
#1941=CARTESIAN_POINT ( 'NONE',  ( 34.52528910822917396, -5.407089921784861808, 168.7762980561585380 ) ) ;
#1949=CARTESIAN_POINT ( 'NONE',  ( 20.99999999999999645, 6.928203230275506996, -6.862499999999990941 ) ) ;
#1950=CARTESIAN_POINT ( 'NONE',  ( 15.00000000000000000, 0.000000000000000000, -3.093749998770961795 ) ) ;
#1954=( BOUNDED_CURVE ( )  B_SPLINE_CURVE ( 2, ( #28163, #8083, #30649, #25506, #1824, #24944, #13393 ),
 .UNSPECIFIED., .F., .F. ) 
 B_SPLINE_CURVE_WITH_KNOTS ( ( 3, 2, 2, 3 ),
 ( 0.3478260869565212854, 0.3550724637681154094, 0.3623188405797094780, 0.3695652173913035465 ),
 .UNSPECIFIED. ) 
 CURVE ( )  GEOMETRIC_REPRESENTATION_ITEM ( )  RATIONAL_B_SPLINE_CURVE ( ( 1.000000000000008216, 0.8660254037844304920, 1.000000000000000000, 0.8660254037844387076, 1.000000000000000000, 0.8660254037844530295, 0.9999999999999856781 ) ) 
 REPRESENTATION_ITEM ( '' )  );
#1960=ORIENTED_EDGE ( 'NONE', *, *, #2267, .F. ) ;
#1967=CARTESIAN_POINT ( 'NONE',  ( 37.07307153918868181, 7.347880794884117764E-16, 164.8737688849411143 ) ) ;
#1977=CARTESIAN_POINT ( 'NONE',  ( 37.01584409946383403, -3.604726614523235284, 161.4250080079952170 ) ) ;
#1978=CARTESIAN_POINT ( 'NONE',  ( 24.93570810221097034, -3.464101615138005741, 163.8276289306958233 ) ) ;
#1983=ORIENTED_EDGE ( 'NONE', *, *, #32619, .F. ) ;
#1985=CARTESIAN_POINT ( 'NONE',  ( 23.99999999999999645, 5.196152422706631135, -4.143749998770957177 ) ) ;
#1988=CYLINDRICAL_SURFACE ( 'NONE', #26802, 6.000000000000001776 ) ;
#1996=CARTESIAN_POINT ( 'NONE',  ( 24.93897644267070035, 3.464101615137752166, 163.8649862330987048 ) ) ;
#2001=CARTESIAN_POINT ( 'NONE',  ( 20.99999999999999645, -6.646953231504538984, -2.840624999385488181 ) ) ;
#2010=CARTESIAN_POINT ( 'NONE',  ( 24.86547026816695904, 3.604726614523240613, 165.8194550616826461 ) ) ;
#2025=CARTESIAN_POINT ( 'NONE',  ( 15.00000000000000000, 3.464101615137752166, -2.287500000000007638 ) ) ;
#2028=CARTESIAN_POINT ( 'NONE',  ( 33.87162103762178589, 5.407089921784862696, 161.3048378204704534 ) ) ;
#2030=CARTESIAN_POINT ( 'NONE',  ( 33.83282523762249383, -5.196152422706635576, 162.2587239212197971 ) ) ;
#2038=CARTESIAN_POINT ( 'NONE',  ( 26.99999999999999645, 7.347880794884117764E-16, -1.124999999999987121 ) ) ;
#2040=CARTESIAN_POINT ( 'NONE',  ( 21.00000000000000000, 6.646953231504538984, -9.815624999385470062 ) ) ;
#2056=CARTESIAN_POINT ( 'NONE',  ( 24.55988044515800439, 0.000000000000000000, 162.3265474014984591 ) ) ;
#2059=CARTESIAN_POINT ( 'NONE',  ( 36.86389775648778055, -3.464101615137418211, 162.4829016082964870 ) ) ;
#2060=CARTESIAN_POINT ( 'NONE',  ( 27.72819177541068214, 5.196152422706630247, 161.3247236329709153 ) ) ;
#2062=DIRECTION ( 'NONE',  ( 0.9961946980917462113, 0.000000000000000000, -0.08715574274765118534 ) ) ;
#2068=CARTESIAN_POINT ( 'NONE',  ( 31.04442699002431993, 7.209453229046475009, 164.8083258472544230 ) ) ;
#2069=CARTESIAN_POINT ( 'NONE',  ( 15.24356964375000167, -3.323476615752272600, -4.603124999385474148 ) ) ;
#2071=CARTESIAN_POINT ( 'NONE',  ( 34.52528910822917396, -5.407089921784861808, 168.7762980561585380 ) ) ;
#2073=CARTESIAN_POINT ( 'NONE',  ( 28.43742163191258499, -5.196152422706638241, 169.4312579874681148 ) ) ;
#2079=VERTEX_POINT ( 'NONE', #21052 ) ;
#2080=ORIENTED_EDGE ( 'NONE', *, *, #22684, .F. ) ;
#2084=AXIS2_PLACEMENT_3D ( 'NONE', #26295, #17974, #2991 ) ;
#2085=CARTESIAN_POINT ( 'NONE',  ( 18.12178482187499640, 4.985214923628404904, -3.365624999385474769 ) ) ;
#2088=CARTESIAN_POINT ( 'NONE',  ( 26.75643035624999655, -3.323476615752267715, -1.865624999385470772 ) ) ;
#2093=( BOUNDED_CURVE ( )  B_SPLINE_CURVE ( 2, ( #2964, #14532, #17944, #15093, #20983, #26642, #12807 ),
 .UNSPECIFIED., .F., .F. ) 
 B_SPLINE_CURVE_WITH_KNOTS ( ( 3, 2, 2, 3 ),
 ( 0.7608695652173899093, 0.7681159420289841444, 0.7753623188405783795, 0.7826086956521727256 ),
 .UNSPECIFIED. ) 
 CURVE ( )  GEOMETRIC_REPRESENTATION_ITEM ( )  RATIONAL_B_SPLINE_CURVE ( ( 1.000000000000026645, 0.8660254037844120623, 1.000000000000000000, 0.8660254037844387076, 1.000000000000000000, 0.8660254037844612451, 0.9999999999999774625 ) ) 
 REPRESENTATION_ITEM ( '' )  );
#2101=CARTESIAN_POINT ( 'NONE',  ( 21.00000000000000355, 0.000000000000000000, 50.00000000000001421 ) ) ;
#2107=VERTEX_POINT ( 'NONE', #23887 ) ;
#2108=CYLINDRICAL_SURFACE ( 'NONE', #17316, 5.999999999999994671 ) ;
#2114=CARTESIAN_POINT ( 'NONE',  ( 26.99999999999999645, 7.347880794884117764E-16, -1.518749998770940746 ) ) ;
#2117=CARTESIAN_POINT ( 'NONE',  ( 24.00000000000000000, -5.196152422706629359, -8.399999999999991473 ) ) ;
#2123=CARTESIAN_POINT ( 'NONE',  ( 26.75643035624999655, 3.323476615752271712, -7.190624999385489602 ) ) ;
#2151=CARTESIAN_POINT ( 'NONE',  ( 24.99999999999999289, 0.000000000000000000, -8.000000000000000000 ) ) ;
#2162=CARTESIAN_POINT ( 'NONE',  ( 33.86345018673919327, -5.407089921784855591, 161.2114445675243530 ) ) ;
#2163=CARTESIAN_POINT ( 'NONE',  ( 21.00000000000000000, 6.646953231504538984, -0.8156249993854914893 ) ) ;
#2169=CARTESIAN_POINT ( 'NONE',  ( 21.00000000000000000, -6.928203230275506996, -5.681249998770944387 ) ) ;
#2170=CARTESIAN_POINT ( 'NONE',  ( 20.99999999999999645, 6.646953231504538984, -3.403124999385474858 ) ) ;
#2172=CARTESIAN_POINT ( 'NONE',  ( 15.00000000000021316, 3.464101615137874735, -4.537499999999988987 ) ) ;
#2179=CARTESIAN_POINT ( 'NONE',  ( 37.03385145495223441, 7.347880794884117764E-16, 164.4254812707998497 ) ) ;
#2184=CARTESIAN_POINT ( 'NONE',  ( 18.12178482187499640, 4.985214923628404904, -2.578124999385478233 ) ) ;
#2190=CARTESIAN_POINT ( 'NONE',  ( 26.99999999999983658, -3.464101615137843648, -6.562499999999986677 ) ) ;
#2193=CARTESIAN_POINT ( 'NONE',  ( 17.00000000000000000, 4.898587196589406912E-16, 50.17464377163448574 ) ) ;
#2194=CARTESIAN_POINT ( 'NONE',  ( 37.24953043470598146, 7.646167579472024665E-16, 164.0960550422537096 ) ) ;
#2196=VECTOR ( 'NONE', #32723, 1000.000000000000114 ) ;
#2210=CARTESIAN_POINT ( 'NONE',  ( 26.99999999999999645, 7.347880794884117764E-16, -3.374999999999989342 ) ) ;
#2211=CARTESIAN_POINT ( 'NONE',  ( 25.96202780814182631, -3.113882786269718483, -8.000000000000003553 ) ) ;
#2212=CARTESIAN_POINT ( 'NONE',  ( 36.97825818540390941, 3.604726614523243278, 160.9953990444431611 ) ) ;
#2214=CARTESIAN_POINT ( 'NONE',  ( 34.50404489593442747, 5.407089921784857367, 168.5334755984986828 ) ) ;
#2219=ORIENTED_EDGE ( 'NONE', *, *, #1145, .T. ) ;
#2224=CARTESIAN_POINT ( 'NONE',  ( 26.75643035624999655, 3.323476615752271712, -9.440624999385470062 ) ) ;
#2236=EDGE_CURVE ( 'NONE', #14024, #33229, #26477, .T. ) ;
#2240=CARTESIAN_POINT ( 'NONE',  ( 33.98111043944852128, -5.407089921784855591, 162.5563074099482037 ) ) ;
#2243=CYLINDRICAL_SURFACE ( 'NONE', #18562, 5.999999999999994671 ) ;
#2251=CARTESIAN_POINT ( 'NONE',  ( 34.11184405356999605, 5.407089921784857367, 164.0505994570858093 ) ) ;
#2252=CARTESIAN_POINT ( 'NONE',  ( 21.00000000000000000, 6.646953231504538984, -4.303124999385465443 ) ) ;
#2255=CARTESIAN_POINT ( 'NONE',  ( 28.20742792136773858, 5.407089921784862696, 168.1997419705030552 ) ) ;
#2256=CARTESIAN_POINT ( 'NONE',  ( 34.19887935716262461, 5.196152422706637353, 166.4427416532051609 ) ) ;
#2266=LINE ( 'NONE', #16314, #18341 ) ;
#2267=EDGE_CURVE ( 'NONE', #1610, #12755, #4683, .T. ) ;
#2268=CARTESIAN_POINT ( 'NONE',  ( 23.87821517812499650, 4.985214923628404904, -4.340624999385478411 ) ) ;
#2271=CARTESIAN_POINT ( 'NONE',  ( 18.12178482187500350, -4.985214923628407568, -0.6281249993854709501 ) ) ;
#2279=CARTESIAN_POINT ( 'NONE',  ( 26.97716818855048260, 0.000000000000000000, 49.47706554351410801 ) ) ;
#2289=( BOUNDED_CURVE ( )  B_SPLINE_CURVE ( 2, ( #27246, #1836, #16257, #30474, #1269, #21760, #1651 ),
 .UNSPECIFIED., .F., .F. ) 
 B_SPLINE_CURVE_WITH_KNOTS ( ( 3, 2, 2, 3 ),
 ( 0.7173913043478249429, 0.7246376811594196221, 0.7318840579710143013, 0.7349428514613199903 ),
 .UNSPECIFIED. ) 
 CURVE ( )  GEOMETRIC_REPRESENTATION_ITEM ( )  RATIONAL_B_SPLINE_CURVE ( ( 1.000000000000020428, 0.8660254037844181685, 1.000000000000000000, 0.8660254037844387076, 1.000000000000000000, 0.9434475140576754626, 0.9346381638529801528 ) ) 
 REPRESENTATION_ITEM ( '' )  );
#2299=CARTESIAN_POINT ( 'NONE',  ( 23.99999999999999645, 5.196152422706631135, -2.849999999999991651 ) ) ;
#2302=CARTESIAN_POINT ( 'NONE',  ( 25.01087993033039325, 0.000000000000000000, 164.6868468578000488 ) ) ;
#2305=CARTESIAN_POINT ( 'NONE',  ( 26.99999999999999645, 3.464101615137755275, -8.287500000000004974 ) ) ;
#2312=CARTESIAN_POINT ( 'NONE',  ( 21.00000000000000000, 6.646953231504538984, -7.115624999385463667 ) ) ;
#2316=ORIENTED_EDGE ( 'NONE', *, *, #22130, .T. ) ;
#2321=CARTESIAN_POINT ( 'NONE',  ( 28.20742792136773858, 5.407089921784862696, 168.1997419705030552 ) ) ;
#2323=CARTESIAN_POINT ( 'NONE',  ( 37.38683221308021842, 7.347880794884117764E-16, 168.4600697980714017 ) ) ;
#2343=CARTESIAN_POINT ( 'NONE',  ( 25.29522554115172639, 0.000000000000000000, 167.9369320615487311 ) ) ;
#2354=CARTESIAN_POINT ( 'NONE',  ( 37.01911243981686539, 7.646167579472015790E-16, 161.4623653091736628 ) ) ;
#2359=ORIENTED_EDGE ( 'NONE', *, *, #5005, .F. ) ;
#2360=CARTESIAN_POINT ( 'NONE',  ( 15.00000000000000000, 3.464101615137752166, -5.831249998770964282 ) ) ;
#2361=CARTESIAN_POINT ( 'NONE',  ( 26.75643035624999655, -3.323476615752267271, -3.103124999385467042 ) ) ;
#2370=CARTESIAN_POINT ( 'NONE',  ( 24.98473320761322114, -3.464101615137757051, 164.3879884495968611 ) ) ;
#2374=CARTESIAN_POINT ( 'NONE',  ( 26.75643035624999655, 3.323476615752271268, -1.340624999385481075 ) ) ;
#2381=EDGE_CURVE ( 'NONE', #34425, #11807, #4459, .T. ) ;
#2383=CARTESIAN_POINT ( 'NONE',  ( 25.44230085693126497, 0.000000000000000000, 169.6180106133541869 ) ) ;
#2384=CARTESIAN_POINT ( 'NONE',  ( 30.88264414254898682, 7.209453229046482114, 162.9591394389216532 ) ) ;
#2398=CARTESIAN_POINT ( 'NONE',  ( 15.00000000000000000, 0.000000000000000000, -4.049999999999998046 ) ) ;
#2399=CARTESIAN_POINT ( 'NONE',  ( 25.55176585154777769, -3.713212129012403828, -8.000000000000000000 ) ) ;
#2401=CARTESIAN_POINT ( 'NONE',  ( 33.61057809361597748, 5.196152422706637353, 159.7184274410858507 ) ) ;
#2404=ADVANCED_FACE ( 'NONE', ( #11971 ), #31579, .F. ) ;
#2411=CARTESIAN_POINT ( 'NONE',  ( 23.87821517812499650, 4.985214923628404904, -8.053124999385484983 ) ) ;
#2415=CARTESIAN_POINT ( 'NONE',  ( 28.46356835473687852, 5.196152422706636465, 169.7301163968956530 ) ) ;
#2416=CARTESIAN_POINT ( 'NONE',  ( 30.78459393195788607, -7.209453229046482114, 161.8384204035683922 ) ) ;
#2426=CARTESIAN_POINT ( 'NONE',  ( 37.56002276824448671, -3.604726614523238837, 167.6449986542055797 ) ) ;
#2429=CARTESIAN_POINT ( 'NONE',  ( 26.99999999999999645, 7.347880794884117764E-16, -6.468749998770951137 ) ) ;
#2437=CARTESIAN_POINT ( 'NONE',  ( 27.59788244552635206, -5.407089921784859143, 161.2326053007238897 ) ) ;
#2438=CARTESIAN_POINT ( 'NONE',  ( 15.24356964374999990, 3.323476615752268604, -8.728124999385462601 ) ) ;
#2441=CARTESIAN_POINT ( 'NONE',  ( 34.44684893975629336, -5.407089921784861808, 167.8797228278759803 ) ) ;
#2442=CARTESIAN_POINT ( 'NONE',  ( 37.10248660225891371, 7.347880794884125653E-16, 165.2099845943227479 ) ) ;
#2456=CARTESIAN_POINT ( 'NONE',  ( 15.24356964375000167, -3.323476615752272600, -1.115624999385467442 ) ) ;
#2470=VECTOR ( 'NONE', #10254, 1000.000000000000000 ) ;
#2474=ADVANCED_FACE ( 'NONE', ( #32117 ), #1777, .T. ) ;
#2480=CARTESIAN_POINT ( 'NONE',  ( 25.32464060422194052, 0.000000000000000000, 168.2731477709303363 ) ) ;
#2493=CARTESIAN_POINT ( 'NONE',  ( 23.87821517812499650, 4.985214923628404904, -8.053124999385484983 ) ) ;
#2499=CARTESIAN_POINT ( 'NONE',  ( 37.37045902776835504, 3.604726614523243278, 165.4782751858559777 ) ) ;
#2503=CARTESIAN_POINT ( 'NONE',  ( 15.00000000000000000, 0.000000000000000000, -7.649999999999989697 ) ) ;
#2506=( BOUNDED_SURFACE ( )  B_SPLINE_SURFACE ( 1, 2, ( 
 ( #13707, #36433, #4971, #33972, #19780, #1760, #25259, #19222, #1941, #13512, #36621, #10475, #30586, #11037, #30953, #4789, #10663, #33417, #22052, #4602, #16181, #22243, #33606, #7645, #28282, #36808, #27731, #16552, #24697, #16922, #10850, #8013, #10292, #19588, #31137, #36993, #5155, #16735, #2321, #31315, #13892, #25439, #28463, #13143, #36249, #29013, #11965, #34898, #215, #31867, #5522, #20327, #37357, #34707, #8940, #26178, #8754, #26364, #11410, #3057, #17106, #28832, #11780, #34343, #14627, #20516, #20697, #3246, #17480, #23346, #17292, #32054, #25623, #22979, #5900, #2867, #14820, #6084, #11590, #17669, #14440, #25995, #29205, #24, #34528, #6282, #399, #23536, #35081, #2499, #28646, #9131, #32242, #17857, #14073, #37180, #23166, #11221, #8388, #22793, #19957, #31499, #2684, #14259, #25809, #8568, #20135, #31681, #5711, #1343, #18046, #6850, #35458, #32622, #29778, #6660, #15194, #23726, #27313, #9695, #9508, #21084, #12149, #29588, #20889, #35264, #3808, #26741, #23917, #7051, #18425, #32430, #26934, #3433, #33191, #12343, #18234, #26553, #35837, #12724, #15764, #27128, #15384, #964, #12915, #1153, #582, #21271, #30161, #29969, #3998, #24478, #24293, #9879, #32809, #6475, #15572, #775, #24104, #21459, #32999, #35649, #36024, #12540, #18619, #3625, #4190, #10064, #9319, #21639, #7234, #29399, #15001, #34260, #19876, #33567, #5438, #4374, #27689, #37092, #8122, #20054, #31418, #28380, #22896, #19693, #5263, #13989, #31233, #1717, #23077, #17020, #28745, #28559, #18808, #33380, #2600, #2785, #14172, #25726, #25540, #2416, #37279, #24656, #11326, #16840, #11140, #7418, #17206, #34444, #30350, #1528, #5622, #22717, #8304, #21827, #34623, #16138, #24843, #8483, #14359, #25913, #13287, #31599, #37458, #11508, #15953, #36207, #36394, #27506, #13101, #10251, #10440, #18989, #30546, #4563, #22013, #32526, #6001, #35179, #11691, #34997, #17954, #2971, #20799, #15101, #26843, #9415, #23636, #9225, #23444, #32341, #31779, #17581, #26462, #9040, #20991, #6379, #17764, #12252, #20612, #32152, #3345, #6192, #29114, #12445, #29497, #18143, #3536 ),
 ( #26651, #14541, #682, #29305, #14913, #23264, #6569, #23822, #20236, #28936, #29685, #496, #12062, #34808, #24013, #3158, #14728, #35364, #3719, #15291, #26277, #873, #8667, #5814, #17396, #26096, #309, #126, #8853, #20427, #31971, #11875, #35742, #27404, #18899, #7510, #24197, #13012, #4099, #1246, #35930, #12816, #21365, #29875, #33468, #15859, #15670, #27221, #18330, #9788, #27035, #3908, #9972, #32904, #30064, #13198, #24566, #1058, #33099, #9603, #1812, #18526, #24385, #32716, #4469, #30451, #21918, #33286, #21552, #7142, #19084, #7324, #6756, #1436, #36299, #36120, #10160, #30635, #16048, #27595, #21735, #12632, #15480, #1626, #18716, #24750, #6958, #4652, #30255, #10346, #4282, #27785, #16234, #13380, #35559, #21177, #8256, #19276, #25307, #36859, #19829, #2738, #24933, #10904, #22478, #36487, #13761, #16606, #7696, #5026, #31368, #25493, #5391, #28148, #2179, #22107, #28701, #25681, #4840, #31551, #16971, #33656, #25122, #28333, #30816, #34025, #8070, #31006, #16419, #11279, #19646, #10717, #11093, #31188, #5211, #33844, #34211, #2556, #22291, #28513, #16788, #7883, #8436, #2370, #13944, #27966, #19457, #37045, #20005, #22667, #14125, #37231, #22849, #34398, #5575, #10531, #17161, #1996, #13569, #36679, #20188, #20562, #8619, #17531, #14491, #34765, #32293, #5765, #11462, #11827, #3295, #29065, #25863, #32476, #2922, #6333, #17715, #14867, #29449, #6523, #3484, #3109, #18097, #34946, #8992, #9368, #14676, #31737, #23775, #31921, #264, #17345, #448, #26226, #28888, #17905, #14310, #26603, #35313, #32104, #26048, #29637, #23216, #12202, #37412, #23031, #34578, #23398, #75, #6137, #9179, #11640, #8807, #29254, #26413, #20379, #12015, #5952, #23586, #35128, #20748, #15054, #633, #20943, #32853, #826, #7458, #4419, #21129, #10295, #21684, #12393, #3860, #7096, #35508, #4046, #15618, #9744, #23965, #27547, #6903, #26983, #27358, #35879, #18475, #12583, #12961, #18849, #1009, #33236, #9921, #24149, #24700, #27172, #1196, #6709, #35692, #24339, #36252, #21316, #30016, #21505, #7275, #30396, #24519, #3673, #21867, #19037, #33420 ) ),
 .UNSPECIFIED., .F., .F., .F. ) 
 B_SPLINE_SURFACE_WITH_KNOTS ( ( 2, 2 ),
 ( 3, 2, 2, 2, 2, 2, 2, 2, 2, 2, 2, 2, 2, 2, 2, 2, 2, 2, 2, 2, 2, 2, 2, 2, 2, 2, 2, 2, 2, 2, 2, 2, 2, 2, 2, 2, 2, 2, 2, 2, 2, 2, 2, 2, 2, 2, 2, 2, 2, 2, 2, 2, 2, 2, 2, 2, 2, 2, 2, 2, 2, 2, 2, 2, 2, 2, 2, 2, 2, 2, 2, 2, 2, 2, 2, 2, 2, 2, 2, 2, 2, 2, 2, 2, 2, 2, 2, 2, 2, 2, 2, 2, 2, 2, 2, 2, 2, 2, 2, 2, 2, 2, 2, 2, 2, 2, 2, 2, 2, 2, 2, 2, 2, 2, 2, 2, 2, 2, 2, 2, 2, 2, 2, 2, 2, 2, 2, 2, 2, 2, 2, 2, 2, 2, 3 ),
 ( 0.000000000000000000, 1.000000000000000000 ),
 ( 0.000000000000000000, 0.007246376811594202987, 0.01449275362318840597, 0.02173913043478260809, 0.02898550724637681195, 0.03623188405797101580, 0.04347826086956521618, 0.05072463768115942351, 0.05797101449275362389, 0.06521739130434782428, 0.07246376811594203160, 0.07971014492753622505, 0.08695652173913043237, 0.09420289855072463969, 0.1014492753623188470, 0.1086956521739130405, 0.1159420289855072478, 0.1231884057971014551, 0.1304347826086956486, 0.1376811594202898559, 0.1449275362318840632, 0.1521739130434782705, 0.1594202898550724501, 0.1666666666666666574, 0.1739130434782608647, 0.1811594202898550721, 0.1884057971014492794, 0.1956521739130434867, 0.2028985507246376940, 0.2101449275362318736, 0.2173913043478260809, 0.2246376811594202882, 0.2318840579710144956, 0.2391304347826087029, 0.2463768115942029102, 0.2536231884057971175, 0.2608695652173912971, 0.2681159420289855322, 0.2753623188405797118, 0.2826086956521738913, 0.2898550724637681264, 0.2971014492753623060, 0.3043478260869565410, 0.3115942028985507206, 0.3188405797101449002, 0.3260869565217391353, 0.3333333333333333148, 0.3405797101449275499, 0.3478260869565217295, 0.3550724637681159646, 0.3623188405797101441, 0.3695652173913043237, 0.3768115942028985588, 0.3840579710144927383, 0.3913043478260869734, 0.3985507246376811530, 0.4057971014492753881, 0.4130434782608695676, 0.4202898550724637472, 0.4275362318840579823, 0.4347826086956521618, 0.4420289855072463969, 0.4492753623188405765, 0.4565217391304347561, 0.4637681159420289911, 0.4710144927536231707, 0.4782608695652174058, 0.4855072463768115854, 0.4927536231884058204, 0.5000000000000000000, 0.5072463768115942351, 0.5144927536231883591, 0.5217391304347825942, 0.5289855072463768293, 0.5362318840579710644, 0.5434782608695651884, 0.5507246376811594235, 0.5579710144927536586, 0.5652173913043477826, 0.5724637681159420177, 0.5797101449275362528, 0.5869565217391304879, 0.5942028985507246119, 0.6014492753623188470, 0.6086956521739130821, 0.6159420289855072062, 0.6231884057971014412, 0.6304347826086956763, 0.6376811594202898004, 0.6449275362318840354, 0.6521739130434782705, 0.6594202898550725056, 0.6666666666666666297, 0.6739130434782608647, 0.6811594202898550998, 0.6884057971014492239, 0.6956521739130434590, 0.7028985507246376940, 0.7101449275362319291, 0.7173913043478260532, 0.7246376811594202882, 0.7318840579710145233, 0.7391304347826086474, 0.7463768115942028825, 0.7536231884057971175, 0.7608695652173913526, 0.7681159420289854767, 0.7753623188405797118, 0.7826086956521739468, 0.7898550724637680709, 0.7971014492753623060, 0.8043478260869565410, 0.8115942028985507761, 0.8188405797101449002, 0.8260869565217391353, 0.8333333333333333703, 0.8405797101449274944, 0.8478260869565217295, 0.8550724637681159646, 0.8623188405797101996, 0.8695652173913043237, 0.8768115942028985588, 0.8840579710144927938, 0.8913043478260869179, 0.8985507246376811530, 0.9057971014492753881, 0.9130434782608695121, 0.9202898550724637472, 0.9275362318840579823, 0.9347826086956522174, 0.9420289855072463414, 0.9492753623188405765, 0.9565217391304348116, 0.9637681159420289356, 0.9662082944262200268 ),
 .UNSPECIFIED. ) 
 GEOMETRIC_REPRESENTATION_ITEM ( )  RATIONAL_B_SPLINE_SURFACE ( (
 ( 1.000000000000000000, 0.8660254037844387076, 1.000000000000000000, 0.8660254037844387076, 1.000000000000000000, 0.8660254037844387076, 1.000000000000000000, 0.8660254037844387076, 1.000000000000000000, 0.8660254037844387076, 1.000000000000000000, 0.8660254037844387076, 1.000000000000000000, 0.8660254037844387076, 1.000000000000000000, 0.8660254037844387076, 1.000000000000000000, 0.8660254037844387076, 1.000000000000000000, 0.8660254037844387076, 1.000000000000000000, 0.8660254037844387076, 1.000000000000000000, 0.8660254037844387076, 1.000000000000000000, 0.8660254037844387076, 1.000000000000000000, 0.8660254037844387076, 1.000000000000000000, 0.8660254037844387076, 1.000000000000000000, 0.8660254037844387076, 1.000000000000000000, 0.8660254037844387076, 1.000000000000000000, 0.8660254037844387076, 1.000000000000000000, 0.8660254037844387076, 1.000000000000000000, 0.8660254037844387076, 1.000000000000000000, 0.8660254037844387076, 1.000000000000000000, 0.8660254037844387076, 1.000000000000000000, 0.8660254037844387076, 1.000000000000000000, 0.8660254037844387076, 1.000000000000000000, 0.8660254037844387076, 1.000000000000000000, 0.8660254037844387076, 1.000000000000000000, 0.8660254037844387076, 1.000000000000000000, 0.8660254037844387076, 1.000000000000000000, 0.8660254037844387076, 1.000000000000000000, 0.8660254037844387076, 1.000000000000000000, 0.8660254037844387076, 1.000000000000000000, 0.8660254037844387076, 1.000000000000000000, 0.8660254037844387076, 1.000000000000000000, 0.8660254037844387076, 1.000000000000000000, 0.8660254037844387076, 1.000000000000000000, 0.8660254037844387076, 1.000000000000000000, 0.8660254037844387076, 1.000000000000000000, 0.8660254037844387076, 1.000000000000000000, 0.8660254037844387076, 1.000000000000000000, 0.8660254037844387076, 1.000000000000000000, 0.8660254037844387076, 1.000000000000000000, 0.8660254037844387076, 1.000000000000000000, 0.8660254037844387076, 1.000000000000000000, 0.8660254037844387076, 1.000000000000000000, 0.8660254037844387076, 1.000000000000000000, 0.8660254037844387076, 1.000000000000000000, 0.8660254037844387076, 1.000000000000000000, 0.8660254037844387076, 1.000000000000000000, 0.8660254037844387076, 1.000000000000000000, 0.8660254037844387076, 1.000000000000000000, 0.8660254037844387076, 1.000000000000000000, 0.8660254037844387076, 1.000000000000000000, 0.8660254037844387076, 1.000000000000000000, 0.8660254037844387076, 1.000000000000000000, 0.8660254037844387076, 1.000000000000000000, 0.8660254037844387076, 1.000000000000000000, 0.8660254037844387076, 1.000000000000000000, 0.8660254037844387076, 1.000000000000000000, 0.8660254037844387076, 1.000000000000000000, 0.8660254037844387076, 1.000000000000000000, 0.8660254037844387076, 1.000000000000000000, 0.8660254037844387076, 1.000000000000000000, 0.8660254037844387076, 1.000000000000000000, 0.8660254037844387076, 1.000000000000000000, 0.8660254037844387076, 1.000000000000000000, 0.8660254037844387076, 1.000000000000000000, 0.8660254037844387076, 1.000000000000000000, 0.8660254037844387076, 1.000000000000000000, 0.8660254037844387076, 1.000000000000000000, 0.8660254037844387076, 1.000000000000000000, 0.8660254037844387076, 1.000000000000000000, 0.8660254037844387076, 1.000000000000000000, 0.8660254037844387076, 1.000000000000000000, 0.8660254037844387076, 1.000000000000000000, 0.8660254037844387076, 1.000000000000000000, 0.8660254037844387076, 1.000000000000000000, 0.8660254037844387076, 1.000000000000000000, 0.8660254037844387076, 1.000000000000000000, 0.8660254037844387076, 1.000000000000000000, 0.8660254037844387076, 1.000000000000000000, 0.8660254037844387076, 1.000000000000000000, 0.8660254037844387076, 1.000000000000000000, 0.8660254037844387076, 1.000000000000000000, 0.8660254037844387076, 1.000000000000000000, 0.8660254037844387076, 1.000000000000000000, 0.8660254037844387076, 1.000000000000000000, 0.8660254037844387076, 1.000000000000000000, 0.8660254037844387076, 1.000000000000000000, 0.8660254037844387076, 1.000000000000000000, 0.8660254037844387076, 1.000000000000000000, 0.8660254037844387076, 1.000000000000000000, 0.8660254037844387076, 1.000000000000000000, 0.8660254037844387076, 1.000000000000000000, 0.8660254037844387076, 1.000000000000000000, 0.8660254037844387076, 1.000000000000000000, 0.8660254037844387076, 1.000000000000000000, 0.8660254037844387076, 1.000000000000000000, 0.8660254037844387076, 1.000000000000000000, 0.8660254037844387076, 1.000000000000000000, 0.8660254037844387076, 1.000000000000000000, 0.8660254037844387076, 1.000000000000000000, 0.8660254037844387076, 1.000000000000000000, 0.8660254037844387076, 1.000000000000000000, 0.8660254037844387076, 1.000000000000000000, 0.8660254037844387076, 1.000000000000000000, 0.8660254037844387076, 1.000000000000000000, 0.8660254037844387076, 1.000000000000000000, 0.8660254037844387076, 1.000000000000000000, 0.8660254037844387076, 1.000000000000000000, 0.8660254037844387076, 1.000000000000000000, 0.8660254037844387076, 1.000000000000000000, 0.8660254037844387076, 1.000000000000000000, 0.8660254037844387076, 1.000000000000000000, 0.8660254037844387076, 1.000000000000000000, 0.8660254037844387076, 1.000000000000000000, 0.8660254037844387076, 1.000000000000000000, 0.8660254037844387076, 1.000000000000000000, 0.8660254037844387076, 1.000000000000000000, 0.8660254037844387076, 1.000000000000000000, 0.8660254037844387076, 1.000000000000000000, 0.8660254037844387076, 1.000000000000000000, 0.8660254037844387076, 1.000000000000000000, 0.8660254037844387076, 1.000000000000000000, 0.8660254037844387076, 1.000000000000000000, 0.8660254037844387076, 1.000000000000000000, 0.8660254037844387076, 1.000000000000000000, 0.8660254037844387076, 1.000000000000000000, 0.8660254037844387076, 1.000000000000000000, 0.8660254037844387076, 1.000000000000000000, 0.8660254037844387076, 1.000000000000000000, 0.8660254037844387076, 1.000000000000000000, 0.8660254037844387076, 1.000000000000000000, 0.8660254037844387076, 1.000000000000000000, 0.9548847740583508159, 0.9401541683247176540),
 ( 1.000000000000000000, 0.8660254037844387076, 1.000000000000000000, 0.8660254037844387076, 1.000000000000000000, 0.8660254037844387076, 1.000000000000000000, 0.8660254037844387076, 1.000000000000000000, 0.8660254037844387076, 1.000000000000000000, 0.8660254037844387076, 1.000000000000000000, 0.8660254037844387076, 1.000000000000000000, 0.8660254037844387076, 1.000000000000000000, 0.8660254037844387076, 1.000000000000000000, 0.8660254037844387076, 1.000000000000000000, 0.8660254037844387076, 1.000000000000000000, 0.8660254037844387076, 1.000000000000000000, 0.8660254037844387076, 1.000000000000000000, 0.8660254037844387076, 1.000000000000000000, 0.8660254037844387076, 1.000000000000000000, 0.8660254037844387076, 1.000000000000000000, 0.8660254037844387076, 1.000000000000000000, 0.8660254037844387076, 1.000000000000000000, 0.8660254037844387076, 1.000000000000000000, 0.8660254037844387076, 1.000000000000000000, 0.8660254037844387076, 1.000000000000000000, 0.8660254037844387076, 1.000000000000000000, 0.8660254037844387076, 1.000000000000000000, 0.8660254037844387076, 1.000000000000000000, 0.8660254037844387076, 1.000000000000000000, 0.8660254037844387076, 1.000000000000000000, 0.8660254037844387076, 1.000000000000000000, 0.8660254037844387076, 1.000000000000000000, 0.8660254037844387076, 1.000000000000000000, 0.8660254037844387076, 1.000000000000000000, 0.8660254037844387076, 1.000000000000000000, 0.8660254037844387076, 1.000000000000000000, 0.8660254037844387076, 1.000000000000000000, 0.8660254037844387076, 1.000000000000000000, 0.8660254037844387076, 1.000000000000000000, 0.8660254037844387076, 1.000000000000000000, 0.8660254037844387076, 1.000000000000000000, 0.8660254037844387076, 1.000000000000000000, 0.8660254037844387076, 1.000000000000000000, 0.8660254037844387076, 1.000000000000000000, 0.8660254037844387076, 1.000000000000000000, 0.8660254037844387076, 1.000000000000000000, 0.8660254037844387076, 1.000000000000000000, 0.8660254037844387076, 1.000000000000000000, 0.8660254037844387076, 1.000000000000000000, 0.8660254037844387076, 1.000000000000000000, 0.8660254037844387076, 1.000000000000000000, 0.8660254037844387076, 1.000000000000000000, 0.8660254037844387076, 1.000000000000000000, 0.8660254037844387076, 1.000000000000000000, 0.8660254037844387076, 1.000000000000000000, 0.8660254037844387076, 1.000000000000000000, 0.8660254037844387076, 1.000000000000000000, 0.8660254037844387076, 1.000000000000000000, 0.8660254037844387076, 1.000000000000000000, 0.8660254037844387076, 1.000000000000000000, 0.8660254037844387076, 1.000000000000000000, 0.8660254037844387076, 1.000000000000000000, 0.8660254037844387076, 1.000000000000000000, 0.8660254037844387076, 1.000000000000000000, 0.8660254037844387076, 1.000000000000000000, 0.8660254037844387076, 1.000000000000000000, 0.8660254037844387076, 1.000000000000000000, 0.8660254037844387076, 1.000000000000000000, 0.8660254037844387076, 1.000000000000000000, 0.8660254037844387076, 1.000000000000000000, 0.8660254037844387076, 1.000000000000000000, 0.8660254037844387076, 1.000000000000000000, 0.8660254037844387076, 1.000000000000000000, 0.8660254037844387076, 1.000000000000000000, 0.8660254037844387076, 1.000000000000000000, 0.8660254037844387076, 1.000000000000000000, 0.8660254037844387076, 1.000000000000000000, 0.8660254037844387076, 1.000000000000000000, 0.8660254037844387076, 1.000000000000000000, 0.8660254037844387076, 1.000000000000000000, 0.8660254037844387076, 1.000000000000000000, 0.8660254037844387076, 1.000000000000000000, 0.8660254037844387076, 1.000000000000000000, 0.8660254037844387076, 1.000000000000000000, 0.8660254037844387076, 1.000000000000000000, 0.8660254037844387076, 1.000000000000000000, 0.8660254037844387076, 1.000000000000000000, 0.8660254037844387076, 1.000000000000000000, 0.8660254037844387076, 1.000000000000000000, 0.8660254037844387076, 1.000000000000000000, 0.8660254037844387076, 1.000000000000000000, 0.8660254037844387076, 1.000000000000000000, 0.8660254037844387076, 1.000000000000000000, 0.8660254037844387076, 1.000000000000000000, 0.8660254037844387076, 1.000000000000000000, 0.8660254037844387076, 1.000000000000000000, 0.8660254037844387076, 1.000000000000000000, 0.8660254037844387076, 1.000000000000000000, 0.8660254037844387076, 1.000000000000000000, 0.8660254037844387076, 1.000000000000000000, 0.8660254037844387076, 1.000000000000000000, 0.8660254037844387076, 1.000000000000000000, 0.8660254037844387076, 1.000000000000000000, 0.8660254037844387076, 1.000000000000000000, 0.8660254037844387076, 1.000000000000000000, 0.8660254037844387076, 1.000000000000000000, 0.8660254037844387076, 1.000000000000000000, 0.8660254037844387076, 1.000000000000000000, 0.8660254037844387076, 1.000000000000000000, 0.8660254037844387076, 1.000000000000000000, 0.8660254037844387076, 1.000000000000000000, 0.8660254037844387076, 1.000000000000000000, 0.8660254037844387076, 1.000000000000000000, 0.8660254037844387076, 1.000000000000000000, 0.8660254037844387076, 1.000000000000000000, 0.8660254037844387076, 1.000000000000000000, 0.8660254037844387076, 1.000000000000000000, 0.8660254037844387076, 1.000000000000000000, 0.8660254037844387076, 1.000000000000000000, 0.8660254037844387076, 1.000000000000000000, 0.8660254037844387076, 1.000000000000000000, 0.8660254037844387076, 1.000000000000000000, 0.8660254037844387076, 1.000000000000000000, 0.8660254037844387076, 1.000000000000000000, 0.8660254037844387076, 1.000000000000000000, 0.8660254037844387076, 1.000000000000000000, 0.8660254037844387076, 1.000000000000000000, 0.8660254037844387076, 1.000000000000000000, 0.8660254037844387076, 1.000000000000000000, 0.8660254037844387076, 1.000000000000000000, 0.8660254037844387076, 1.000000000000000000, 0.8660254037844387076, 1.000000000000000000, 0.8660254037844387076, 1.000000000000000000, 0.8660254037844387076, 1.000000000000000000, 0.8660254037844387076, 1.000000000000000000, 0.8660254037844387076, 1.000000000000000000, 0.8660254037844387076, 1.000000000000000000, 0.9548847740583508159, 0.9401541683247176540) ) ) 
 REPRESENTATION_ITEM ( '' )  SURFACE ( )  );
#2512=CARTESIAN_POINT ( 'NONE',  ( 20.99999999999999645, 0.000000000000000000, -8.000000000000000000 ) ) ;
#2519=ADVANCED_FACE ( 'NONE', ( #4986 ), #21698, .T. ) ;
#2527=DIRECTION ( 'NONE',  ( 0.000000000000000000, 0.000000000000000000, 1.000000000000000000 ) ) ;
#2528=CARTESIAN_POINT ( 'NONE',  ( 24.65789917220240213, 0.000000000000000000, 160.6522583305284968 ) ) ;
#2541=CARTESIAN_POINT ( 'NONE',  ( 30.75027635825099281, -7.209453229046475009, 161.4461687411947821 ) ) ;
#2547=CARTESIAN_POINT ( 'NONE',  ( 24.00000000000000000, -5.196152422706629359, -7.443749998770954335 ) ) ;
#2548=CARTESIAN_POINT ( 'NONE',  ( 20.99999999999999645, -6.646953231504538984, -2.728124999385465266 ) ) ;
#2556=CARTESIAN_POINT ( 'NONE',  ( 36.95867962683237806, 3.464101615137755275, 163.5662633436956810 ) ) ;
#2560=CARTESIAN_POINT ( 'NONE',  ( 26.75643035624999655, 3.323476615752271268, -3.590624999385492178 ) ) ;
#2565=CARTESIAN_POINT ( 'NONE',  ( 36.91619120224290640, 7.347880794884117764E-16, 163.0806184283759706 ) ) ;
#2569=CARTESIAN_POINT ( 'NONE',  ( 33.91084112185822619, 5.407089921784862696, 161.7531254346117464 ) ) ;
#2583=CARTESIAN_POINT ( 'NONE',  ( 15.00000000000000000, 0.000000000000000000, -5.399999999999987921 ) ) ;
#2585=CARTESIAN_POINT ( 'NONE',  ( 27.47531968228746990, -5.407089921784865361, 159.8317065065323845 ) ) ;
#2587=CARTESIAN_POINT ( 'NONE',  ( 37.64990212795299840, 3.604726614523238837, 168.6723244366126551 ) ) ;
#2594=CARTESIAN_POINT ( 'NONE',  ( 18.00000000000000000, 5.196152422706630247, -4.968749998770949361 ) ) ;
#2596=CARTESIAN_POINT ( 'NONE',  ( 18.12178482187499640, 4.985214923628404904, -7.978124999385494576 ) ) ;
#2600=CARTESIAN_POINT ( 'NONE',  ( 33.91084112185822619, 5.407089921784862696, 161.7531254346117464 ) ) ;
#2608=CARTESIAN_POINT ( 'NONE',  ( 25.33444562538816669, 0.000000000000000000, 168.3852196756899957 ) ) ;
#2610=CARTESIAN_POINT ( 'NONE',  ( 34.48606902399273366, -5.407089921784861808, 168.3280104420172449 ) ) ;
#2620=CARTESIAN_POINT ( 'NONE',  ( 27.74168942105997360, 5.407089921784856479, 162.8763265525752786 ) ) ;
#2621=CARTESIAN_POINT ( 'NONE',  ( 26.75643035624999655, 7.049594010296217766E-16, -6.665624999385472371 ) ) ;
#2623=CARTESIAN_POINT ( 'NONE',  ( 25.02561894546576582, 0.000000000000000000, 167.6499628194262357 ) ) ;
#2624=CARTESIAN_POINT ( 'NONE',  ( 31.19395356112219986, -6.928203230275514990, 166.5174223755558955 ) ) ;
#2636=EDGE_CURVE ( 'NONE', #407, #26185, #30970, .T. ) ;
#2637=CARTESIAN_POINT ( 'NONE',  ( 21.00000000000000000, -6.646953231504538984, -2.840624999385488181 ) ) ;
#2644=CARTESIAN_POINT ( 'NONE',  ( 26.99999999999999645, 7.347880794884117764E-16, -2.925000000000010925 ) ) ;
#2649=CARTESIAN_POINT ( 'NONE',  ( 20.99999999999999645, 0.000000000000000000, -8.000000000000000000 ) ) ;
#2655=CARTESIAN_POINT ( 'NONE',  ( 14.99999999999989697, -3.464101615137695767, -2.606249998770969523 ) ) ;
#2658=CARTESIAN_POINT ( 'NONE',  ( 25.01527935017339033, 0.000000000000000000, 50.00000000000000000 ) ) ;
#2660=CARTESIAN_POINT ( 'NONE',  ( 37.60414536301047406, -3.604726614523235284, 168.1493222201144988 ) ) ;
#2678=CARTESIAN_POINT ( 'NONE',  ( 26.75643035624999655, -3.323476615752267715, -9.515624999385494220 ) ) ;
#2680=VERTEX_POINT ( 'NONE', #35055 ) ;
#2684=CARTESIAN_POINT ( 'NONE',  ( 37.32797060317886917, 7.646167579472024665E-16, 164.9926302705362957 ) ) ;
#2691=CARTESIAN_POINT ( 'NONE',  ( 25.22335353682449721, 3.604726614523236616, 169.9100795407218811 ) ) ;
#2692=ORIENTED_EDGE ( 'NONE', *, *, #1304, .T. ) ;
#2694=CARTESIAN_POINT ( 'NONE',  ( 25.32464060422194052, 0.000000000000000000, 168.2731477709303363 ) ) ;
#2718=CARTESIAN_POINT ( 'NONE',  ( 24.48470861703815515, -3.604726614523240613, 161.4673294743943188 ) ) ;
#2720=CARTESIAN_POINT ( 'NONE',  ( 15.24356964375000167, -3.323476615752272600, -1.115624999385467442 ) ) ;
#2725=ORIENTED_EDGE ( 'NONE', *, *, #34443, .F. ) ;
#2726=ORIENTED_EDGE ( 'NONE', *, *, #14588, .T. ) ;
#2727=CARTESIAN_POINT ( 'NONE',  ( 26.99999999999999645, -3.464101615137751278, -6.506249998770941900 ) ) ;
#2728=CARTESIAN_POINT ( 'NONE',  ( 15.24356964374999990, 3.323476615752268604, -2.428124999385457006 ) ) ;
#2730=CARTESIAN_POINT ( 'NONE',  ( 19.00081571707366379, 5.492723647597353320, -10.12707781181608979 ) ) ;
#2733=( BOUNDED_CURVE ( )  B_SPLINE_CURVE ( 3, ( #31686, #26557, #585, #12155 ),
 .UNSPECIFIED., .F., .F. ) 
 B_SPLINE_CURVE_WITH_KNOTS ( ( 4, 4 ),
 ( 3.141592653589793116, 6.283185307179586232 ),
 .UNSPECIFIED. ) 
 CURVE ( )  GEOMETRIC_REPRESENTATION_ITEM ( )  RATIONAL_B_SPLINE_CURVE ( ( 1.000000000000000000, 0.3333333333333333703, 0.3333333333333333703, 1.000000000000000000 ) ) 
 REPRESENTATION_ITEM ( '' )  );
#2736=ADVANCED_FACE ( 'NONE', ( #14977 ), #32026, .F. ) ;
#2738=CARTESIAN_POINT ( 'NONE',  ( 37.07633987954171317, 3.464101615137755275, 164.9111261861195601 ) ) ;
#2742=CARTESIAN_POINT ( 'NONE',  ( 23.87821517812500005, -4.985214923628404016, -3.703124999385493332 ) ) ;
#2753=CARTESIAN_POINT ( 'NONE',  ( 37.09591843811324452, 3.604726614523243278, 162.3402618868670118 ) ) ;
#2756=DIRECTION ( 'NONE',  ( 0.000000000000000000, 0.000000000000000000, 1.000000000000000000 ) ) ;
#2765=CARTESIAN_POINT ( 'NONE',  ( 26.99999999999999645, 7.347880794884117764E-16, -4.275000000000001243 ) ) ;
#2766=DIRECTION ( 'NONE',  ( 0.000000000000000000, 0.000000000000000000, 1.000000000000000000 ) ) ;
#2767=CARTESIAN_POINT ( 'NONE',  ( 36.89654967657799745, 7.646167579472024665E-16, 160.0614665149821576 ) ) ;
#2769=CARTESIAN_POINT ( 'NONE',  ( 24.61867908796596183, 0.000000000000000000, 160.2039707163872038 ) ) ;
#2772=FACE_OUTER_BOUND ( 'NONE', #7674, .T. ) ;
#2774=ORIENTED_EDGE ( 'NONE', *, *, #260, .F. ) ;
#2776=CARTESIAN_POINT ( 'NONE',  ( 30.95863305570354029, -6.928203230275514990, 163.8276966907082226 ) ) ;
#2778=CARTESIAN_POINT ( 'NONE',  ( 27.00000000000036593, 3.464101615137540779, -5.081249998770964282 ) ) ;
#2785=CARTESIAN_POINT ( 'NONE',  ( 37.01747826964035681, 3.604726614523243278, 161.4436866585844541 ) ) ;
#2793=VECTOR ( 'NONE', #22023, 1000.000000000000000 ) ;
#2798=CARTESIAN_POINT ( 'NONE',  ( 36.82301201863464968, 7.646167579472015790E-16, 159.2209272384671976 ) ) ;
#2799=CARTESIAN_POINT ( 'NONE',  ( 24.00000000000000000, -5.196152422706629359, -2.043749998770966414 ) ) ;
#2801=CARTESIAN_POINT ( 'NONE',  ( 24.62194742831963623, -3.464101615138128754, 160.2413280175655643 ) ) ;
#2806=LINE ( 'NONE', #8687, #33009 ) ;
#2809=CARTESIAN_POINT ( 'NONE',  ( 36.98316069593345645, 3.604726614523238837, 161.0514349962108156 ) ) ;
#2810=CARTESIAN_POINT ( 'NONE',  ( 18.12178482187499640, 4.985214923628404904, -6.965624999385466865 ) ) ;
#2812=CARTESIAN_POINT ( 'NONE',  ( 25.02235060511272735, 3.604726614523240613, 167.6126055182477614 ) ) ;
#2813=CARTESIAN_POINT ( 'NONE',  ( 28.14980768084533125, 5.196152422706636465, 166.1438154837653656 ) ) ;
#2823=CARTESIAN_POINT ( 'NONE',  ( 15.00000000000000000, 0.000000000000000000, -2.700000000000008171 ) ) ;
#2825=CARTESIAN_POINT ( 'NONE',  ( 26.75643035624999655, 3.323476615752271712, -1.790624999385476812 ) ) ;
#2839=AXIS2_PLACEMENT_3D ( 'NONE', #27460, #15532, #7009 ) ;
#2841=CARTESIAN_POINT ( 'NONE',  ( 24.00000000000000000, -5.196152422706629359, -0.2999999999999947153 ) ) ;
#2846=CARTESIAN_POINT ( 'NONE',  ( 34.46482481169798717, 5.407089921784857367, 168.0851879843573897 ) ) ;
#2848=CARTESIAN_POINT ( 'NONE',  ( 26.75643035624999655, 3.323476615752271712, -1.228124999385458160 ) ) ;
#2850=CARTESIAN_POINT ( 'NONE',  ( 20.99999999999999645, 0.000000000000000000, -8.000000000000000000 ) ) ;
#2852=CARTESIAN_POINT ( 'NONE',  ( 15.00000000000039613, 3.464101615137982204, -3.131249998770963217 ) ) ;
#2853=CARTESIAN_POINT ( 'NONE',  ( 25.28215217963232675, 3.464101615137679779, 167.7875028556106258 ) ) ;
#2855=CARTESIAN_POINT ( 'NONE',  ( 25.16776026727616511, 0.000000000000000000, 166.4799973143651926 ) ) ;
#2861=CARTESIAN_POINT ( 'NONE',  ( 26.75643035624999655, 7.049594010296217766E-16, -9.478124999385496352 ) ) ;
#2864=ORIENTED_EDGE ( 'NONE', *, *, #24228, .T. ) ;
#2867=CARTESIAN_POINT ( 'NONE',  ( 31.19640481644053409, 7.209453229046482114, 166.5454403520519122 ) ) ;
#2874=CARTESIAN_POINT ( 'NONE',  ( 31.43662783238875136, 7.209453229046475009, 169.2912019886672681 ) ) ;
#2877=CARTESIAN_POINT ( 'NONE',  ( 15.00000000000000000, 0.000000000000000000, -0.3937499987709536242 ) ) ;
#2887=ADVANCED_FACE ( 'NONE', ( #13726 ), #36826, .T. ) ;
#2889=DIRECTION ( 'NONE',  ( 1.000000000000000000, 0.000000000000000000, 0.000000000000000000 ) ) ;
#2896=VECTOR ( 'NONE', #4173, 1000.000000000000000 ) ;
#2899=CARTESIAN_POINT ( 'NONE',  ( 37.11555996377781952, 3.464101615137954671, 165.3594138002608531 ) ) ;
#2901=EDGE_LOOP ( 'NONE', ( #23388, #29483, #13738, #17865, #4823, #28867 ) ) ;
#2905=CARTESIAN_POINT ( 'NONE',  ( 27.55866236128991176, -5.407089921784859143, 160.7843176865825967 ) ) ;
#2906=CARTESIAN_POINT ( 'NONE',  ( 26.75643035624999655, -3.323476615752267715, -3.215624999385490401 ) ) ;
#2912=CARTESIAN_POINT ( 'NONE',  ( 26.99999999999999645, 3.464101615137755275, -7.331249998770939413 ) ) ;
#2913=CARTESIAN_POINT ( 'NONE',  ( 23.87821517812499650, 4.985214923628404904, -3.440624999385466509 ) ) ;
#2914=CARTESIAN_POINT ( 'NONE',  ( 27.00000000000015632, 3.464101615137663348, -6.487500000000022915 ) ) ;
#2922=CARTESIAN_POINT ( 'NONE',  ( 36.83775103377001869, 7.347880794884117764E-16, 162.1840432000934129 ) ) ;
#2927=CARTESIAN_POINT ( 'NONE',  ( 18.12178482187499640, 4.985214923628404904, -5.278124999385486404 ) ) ;
#2928=CARTESIAN_POINT ( 'NONE',  ( 15.00000000000027711, 3.464101615137910706, -0.4874999999999961586 ) ) ;
#2936=CARTESIAN_POINT ( 'NONE',  ( 27.61912665782109499, 5.407089921784862696, 161.4754277583837734 ) ) ;
#2939=EDGE_CURVE ( 'NONE', #15590, #31540, #34457, .T. ) ;
#2941=CARTESIAN_POINT ( 'NONE',  ( 26.99999999999999645, 7.347880794884117764E-16, -4.275000000000001243 ) ) ;
#2943=CARTESIAN_POINT ( 'NONE',  ( 25.40308077269482112, 0.000000000000000000, 169.1697229992128939 ) ) ;
#2950=CARTESIAN_POINT ( 'NONE',  ( 15.00000000000000178, -3.464101615137757051, -4.462499999999992362 ) ) ;
#2952=CARTESIAN_POINT ( 'NONE',  ( 33.89492370443730351, 5.196152422706631135, 162.9685126448345329 ) ) ;
#2954=CARTESIAN_POINT ( 'NONE',  ( 34.53019161875872101, -5.407089921784855591, 168.8323340079261925 ) ) ;
#2964=CARTESIAN_POINT ( 'NONE',  ( 36.74950584413092258, 7.347880794884125653E-16, 161.1753960670511674 ) ) ;
#2965=CARTESIAN_POINT ( 'NONE',  ( 15.24356964374999990, 0.000000000000000000, -6.440624999385469174 ) ) ;
#2968=CARTESIAN_POINT ( 'NONE',  ( 25.20698035151260896, 0.000000000000000000, 166.9282849285064856 ) ) ;
#2970=LINE ( 'NONE', #28558, #1004 ) ;
#2971=CARTESIAN_POINT ( 'NONE',  ( 30.64732363713033081, 7.209453229046482114, 160.2694137540738950 ) ) ;
#2979=EDGE_CURVE ( 'NONE', #31631, #35079, #36888, .T. ) ;
#2984=CARTESIAN_POINT ( 'NONE',  ( 26.60793733450167053, 1.299049382686714882, -8.000000000000000000 ) ) ;
#2985=CARTESIAN_POINT ( 'NONE',  ( 27.51944227705346790, -5.407089921784859143, 160.3360300724413321 ) ) ;
#2986=CARTESIAN_POINT ( 'NONE',  ( 26.99999999999999645, 7.347880794884117764E-16, -1.968749998770946696 ) ) ;
#2991=DIRECTION ( 'NONE',  ( 1.000000000000000000, 0.000000000000000000, 0.000000000000000000 ) ) ;
#2994=CARTESIAN_POINT ( 'NONE',  ( 30.66448242393021673, 6.928203230275514990, 160.4655395846485533 ) ) ;
#2995=ORIENTED_EDGE ( 'NONE', *, *, #23969, .F. ) ;
#2996=CARTESIAN_POINT ( 'NONE',  ( 30.73066631613276556, 7.209453229046475009, 161.2220249341241356 ) ) ;
#2997=CARTESIAN_POINT ( 'NONE',  ( 15.24356964374999990, 0.000000000000000000, -7.790624999385459049 ) ) ;
#2999=CARTESIAN_POINT ( 'NONE',  ( 34.42070221693199272, 5.407089921784862696, 167.5808644184484706 ) ) ;
#3000=CARTESIAN_POINT ( 'NONE',  ( 31.25278368747686741, 6.928203230275514990, 167.1898537967678351 ) ) ;
#3001=CARTESIAN_POINT ( 'NONE',  ( 26.97716818855048260, 0.000000000000000000, 49.47706554351410801 ) ) ;
#3012=CARTESIAN_POINT ( 'NONE',  ( 15.24356964374999990, 0.000000000000000000, -4.303124999385482319 ) ) ;
#3014=VECTOR ( 'NONE', #30318, 1000.000000000000000 ) ;
#3020=CARTESIAN_POINT ( 'NONE',  ( 36.98482634954957859, 7.347880794884125653E-16, 163.8651217518988688 ) ) ;
#3032=CARTESIAN_POINT ( 'NONE',  ( 36.84101937412247452, 3.464101615138092782, 162.2214005012719156 ) ) ;
#3038=CARTESIAN_POINT ( 'NONE',  ( 18.12178482187499640, 4.985214923628404904, -1.115624999385472771 ) ) ;
#3042=CARTESIAN_POINT ( 'NONE',  ( 30.96843807686977001, -6.928203230275506996, 163.9397685954678536 ) ) ;
#3043=LINE ( 'NONE', #5509, #7882 ) ;
#3052=CARTESIAN_POINT ( 'NONE',  ( 21.00000000000000000, -6.646953231504538984, -10.04062499938548392 ) ) ;
#3057=CARTESIAN_POINT ( 'NONE',  ( 25.02888728581879718, -3.604726614523244610, 167.6873201206046815 ) ) ;
#3065=CARTESIAN_POINT ( 'NONE',  ( 34.41253136604939300, -5.407089921784855591, 167.4874711655023418 ) ) ;
#3068=CARTESIAN_POINT ( 'NONE',  ( 15.00000000000000000, 0.000000000000000000, -1.293749998770965526 ) ) ;
#3085=CARTESIAN_POINT ( 'NONE',  ( 36.78545758801501364, -3.464101615137356927, 161.5863263800139293 ) ) ;
#3087=ORIENTED_EDGE ( 'NONE', *, *, #21957, .T. ) ;
#3094=CARTESIAN_POINT ( 'NONE',  ( 23.87821517812500005, -4.985214923628404016, -1.903124999385497063 ) ) ;
#3098=ORIENTED_EDGE ( 'NONE', *, *, #260, .T. ) ;
#3100=CARTESIAN_POINT ( 'NONE',  ( 23.87821517812500005, -4.985214923628404016, -4.490624999385461891 ) ) ;
#3109=CARTESIAN_POINT ( 'NONE',  ( 24.86053627419781265, 3.464101615137752166, 162.9684110048161187 ) ) ;
#3114=CARTESIAN_POINT ( 'NONE',  ( 20.99999999999999645, 6.646953231504538984, -4.415624999385457272 ) ) ;
#3122=CYLINDRICAL_SURFACE ( 'NONE', #484, 5.999999999999994671 ) ;
#3123=CARTESIAN_POINT ( 'NONE',  ( 24.63668644345436931, -3.604726614523244610, 163.2044439791918080 ) ) ;
#3137=CARTESIAN_POINT ( 'NONE',  ( 15.00000000000000178, -3.464101615137757051, -5.812500000000012434 ) ) ;
#3139=DIRECTION ( 'NONE',  ( 0.08715574274765150453, 0.000000000000000000, 0.9961946980917461003 ) ) ;
#3142=CARTESIAN_POINT ( 'NONE',  ( 37.49302179100721588, 3.604726614523238837, 166.8791739800475113 ) ) ;
#3146=VERTEX_POINT ( 'NONE', #36552 ) ;
#3148=LINE ( 'NONE', #28737, #19432 ) ;
#3150=CARTESIAN_POINT ( 'NONE',  ( 24.78536444607796341, 0.000000000000000000, 162.1091930777120069 ) ) ;
#3151=CARTESIAN_POINT ( 'NONE',  ( 21.00000000000000000, -6.646953231504538984, -5.878124999385467397 ) ) ;
#3155=CARTESIAN_POINT ( 'NONE',  ( 31.17434351900397971, 6.928203230275514990, 166.2932785684852490 ) ) ;
#3158=CARTESIAN_POINT ( 'NONE',  ( 31.38024896135242159, 6.928203230275506996, 168.6467885439513452 ) ) ;
#3169=CARTESIAN_POINT ( 'NONE',  ( 34.53836246964132073, 5.407089921784862696, 168.9257272608723213 ) ) ;
#3170=CARTESIAN_POINT ( 'NONE',  ( 15.00000000000000000, 3.464101615137752166, -2.681249998770962151 ) ) ;
#3175=FACE_OUTER_BOUND ( 'NONE', #34338, .T. ) ;
#3178=CYLINDRICAL_SURFACE ( 'NONE', #35316, 5.999999999999994671 ) ;
#3180=CARTESIAN_POINT ( 'NONE',  ( 24.59910052939444824, 0.000000000000000000, 162.7748350156397521 ) ) ;
#3181=CARTESIAN_POINT ( 'NONE',  ( 26.75643035624999655, -3.323476615752267715, -8.503124999385478944 ) ) ;
#3183=CARTESIAN_POINT ( 'NONE',  ( 31.00030439525832193, 7.209453229046482114, 164.3040022813454755 ) ) ;
#3184=CARTESIAN_POINT ( 'NONE',  ( 37.02404643378602600, 7.347880794884125653E-16, 164.3134093660401618 ) ) ;
#3196=CARTESIAN_POINT ( 'NONE',  ( 23.87821517812499650, 4.985214923628404904, -5.353124999385477700 ) ) ;
#3207=DIRECTION ( 'NONE',  ( 0.000000000000000000, 0.000000000000000000, 1.000000000000000000 ) ) ;
#3214=CARTESIAN_POINT ( 'NONE',  ( 25.41288579386105440, 0.000000000000000000, 169.2817949039725818 ) ) ;
#3226=CARTESIAN_POINT ( 'NONE',  ( 18.12178482187500350, -4.985214923628407568, -0.9656249993854615354 ) ) ;
#3230=CARTESIAN_POINT ( 'NONE',  ( 24.98473320761364036, -3.464101615138001744, 164.3879884495968042 ) ) ;
#3235=( BOUNDED_CURVE ( )  B_SPLINE_CURVE ( 2, ( #35009, #3357, #21004, #24208, #27048, #9052, #24025 ),
 .UNSPECIFIED., .F., .F. ) 
 B_SPLINE_CURVE_WITH_KNOTS ( ( 3, 2, 2, 3 ),
 ( 0.5869565217391301548, 0.5942028985507243899, 0.6014492753623187360, 0.6086956521739130821 ),
 .UNSPECIFIED. ) 
 CURVE ( )  GEOMETRIC_REPRESENTATION_ITEM ( )  RATIONAL_B_SPLINE_CURVE ( ( 1.000000000000006217, 0.8660254037844326014, 1.000000000000000000, 0.8660254037844387076, 1.000000000000000000, 0.8660254037844387076, 1.000000000000000000 ) ) 
 REPRESENTATION_ITEM ( '' )  );
#3239=CARTESIAN_POINT ( 'NONE',  ( 15.24356964375000167, -3.323476615752272600, -8.315624999385494931 ) ) ;
#3246=CARTESIAN_POINT ( 'NONE',  ( 37.44236251553515871, -3.604726614523238837, 166.3001358117817006 ) ) ;
#3252=CARTESIAN_POINT ( 'NONE',  ( 37.03385145495223441, 7.347880794884117764E-16, 164.4254812707998497 ) ) ;
#3253=CARTESIAN_POINT ( 'NONE',  ( 34.53019161875872101, -5.407089921784855591, 168.8323340079261925 ) ) ;
#3270=CARTESIAN_POINT ( 'NONE',  ( 26.99999999999981171, 3.464101615137862300, -4.181249998770934617 ) ) ;
#3274=CARTESIAN_POINT ( 'NONE',  ( 15.02283181144952628, 7.347880794884122694E-16, 50.52293445648592751 ) ) ;
#3282=CARTESIAN_POINT ( 'NONE',  ( 23.87821517812499650, 4.985214923628404904, -1.303124999385479876 ) ) ;
#3287=CARTESIAN_POINT ( 'NONE',  ( 23.87821517812500005, -4.985214923628404016, -4.040624999385455496 ) ) ;
#3295=CARTESIAN_POINT ( 'NONE',  ( 27.88507211235645400, 5.196152422706630247, 163.1178740895360306 ) ) ;
#3300=CARTESIAN_POINT ( 'NONE',  ( 18.12178482187499640, 4.985214923628404904, -3.478124999385490135 ) ) ;
#3308=CARTESIAN_POINT ( 'NONE',  ( 14.99999999999946709, 3.464101615137446188, -5.831249998770957177 ) ) ;
#3313=CARTESIAN_POINT ( 'NONE',  ( 15.00000000000000000, 0.000000000000000000, -1.293749998770965526 ) ) ;
#3323=CARTESIAN_POINT ( 'NONE',  ( 18.00000000000000355, -5.196152422706632912, -6.674999999999986500 ) ) ;
#3324=FACE_OUTER_BOUND ( 'NONE', #20908, .T. ) ;
#3325=DIRECTION ( 'NONE',  ( 1.000000000000000000, 0.000000000000000000, 0.000000000000000000 ) ) ;
#3327=CARTESIAN_POINT ( 'NONE',  ( 28.01623001071507701, 5.407089921784856479, 166.0143398515642730 ) ) ;
#3332=ORIENTED_EDGE ( 'NONE', *, *, #6641, .T. ) ;
#3333=CARTESIAN_POINT ( 'NONE',  ( 29.54925929127992745, 5.908847637349538218, 159.6727443940304738 ) ) ;
#3336=CARTESIAN_POINT ( 'NONE',  ( 18.12178482187499640, 4.985214923628404904, -6.515624999385460470 ) ) ;
#3345=CARTESIAN_POINT ( 'NONE',  ( 27.47531968228746990, -5.407089921784865361, 159.8317065065323845 ) ) ;
#3357=CARTESIAN_POINT ( 'NONE',  ( 27.00000000000015632, -3.464101615137659351, -6.112499999999985612 ) ) ;
#3359=CARTESIAN_POINT ( 'NONE',  ( 25.02561894546576582, 0.000000000000000000, 167.6499628194262357 ) ) ;
#3360=CARTESIAN_POINT ( 'NONE',  ( 15.00000000000000000, 3.464101615137752166, -3.131249998770958332 ) ) ;
#3367=CARTESIAN_POINT ( 'NONE',  ( 26.97716818855048260, 0.000000000000000000, 49.47706554351410801 ) ) ;
#3368=ORIENTED_EDGE ( 'NONE', *, *, #25804, .F. ) ;
#3371=CARTESIAN_POINT ( 'NONE',  ( 18.00000000000000355, -5.196152422706632912, -0.3749999999999864553 ) ) ;
#3374=CARTESIAN_POINT ( 'NONE',  ( 37.32797060317886917, 7.646167579472024665E-16, 164.9926302705362957 ) ) ;
#3375=CARTESIAN_POINT ( 'NONE',  ( 25.05336835491987557, -3.464101615137761048, 165.1724917731197593 ) ) ;
#3382=ORIENTED_EDGE ( 'NONE', *, *, #2381, .T. ) ;
#3385=CARTESIAN_POINT ( 'NONE',  ( 30.94882803475154986, 6.928203230275506996, 163.7156247883972071 ) ) ;
#3388=CARTESIAN_POINT ( 'NONE',  ( 26.75643035624999655, -3.323476615752267715, -4.565624999385477167 ) ) ;
#3402=FACE_OUTER_BOUND ( 'NONE', #33356, .T. ) ;
#3403=CARTESIAN_POINT ( 'NONE',  ( 24.73633934067528983, 0.000000000000000000, 161.5488335588110544 ) ) ;
#3413=CARTESIAN_POINT ( 'NONE',  ( 24.91612954363902688, -3.604726614523240613, 166.3984932299484569 ) ) ;
#3414=CARTESIAN_POINT ( 'NONE',  ( 26.75643035624999655, 3.323476615752271712, -1.678124999385453897 ) ) ;
#3415=ADVANCED_FACE ( 'NONE', ( #7387 ), #7759, .T. ) ;
#3416=CARTESIAN_POINT ( 'NONE',  ( 20.99999999999999645, 0.000000000000000000, -8.000000000000000000 ) ) ;
#3418=DIRECTION ( 'NONE',  ( 0.08715574274765150453, 0.000000000000000000, 0.9961946980917461003 ) ) ;
#3426=CARTESIAN_POINT ( 'NONE',  ( 15.24356964374999990, 0.000000000000000000, -1.040624999385481031 ) ) ;
#3429=VERTEX_POINT ( 'NONE', #25189 ) ;
#3433=CARTESIAN_POINT ( 'NONE',  ( 24.78703009969406779, 3.604726614523240613, 164.9228798334000601 ) ) ;
#3440=CARTESIAN_POINT ( 'NONE',  ( 34.21643094486717729, -5.407089921784855591, 165.2460330947959051 ) ) ;
#3463=DIRECTION ( 'NONE',  ( 0.08715574274765150453, 0.000000000000000000, 0.9961946980917461003 ) ) ;
#3471=CARTESIAN_POINT ( 'NONE',  ( 24.40626844856526745, -3.604726614523240613, 160.5707542461117612 ) ) ;
#3472=CARTESIAN_POINT ( 'NONE',  ( 21.00000000000000000, 6.646953231504538984, -1.265624999385487115 ) ) ;
#3475=ORIENTED_EDGE ( 'NONE', *, *, #28590, .T. ) ;
#3477=CARTESIAN_POINT ( 'NONE',  ( 23.87821517812499650, 4.985214923628404904, -4.340624999385478411 ) ) ;
#3478=CARTESIAN_POINT ( 'NONE',  ( 27.63994658577156827, 5.196152422706636465, 160.3160764999286698 ) ) ;
#3482=FACE_OUTER_BOUND ( 'NONE', #24373, .T. ) ;
#3484=CARTESIAN_POINT ( 'NONE',  ( 24.86380461455084756, 0.000000000000000000, 163.0057683059945930 ) ) ;
#3488=CARTESIAN_POINT ( 'NONE',  ( 18.12178482187499640, 4.985214923628404904, -5.728124999385491911 ) ) ;
#3492=CARTESIAN_POINT ( 'NONE',  ( 18.00000000000000355, -5.196152422706632912, -0.7687499987709400795 ) ) ;
#3497=CARTESIAN_POINT ( 'NONE',  ( 33.75396078491245078, 5.407089921784862696, 159.9599749780466027 ) ) ;
#3503=CARTESIAN_POINT ( 'NONE',  ( 24.00000000000000000, -5.196152422706629359, -2.043749998770966414 ) ) ;
#3507=CARTESIAN_POINT ( 'NONE',  ( 37.03385145495223441, 7.347880794884117764E-16, 164.4254812707998497 ) ) ;
#3511=CARTESIAN_POINT ( 'NONE',  ( 15.00000000000000000, 3.464101615137752166, -7.687499999999988454 ) ) ;
#3513=CARTESIAN_POINT ( 'NONE',  ( 26.99999999999999645, 7.347880794884117764E-16, -3.374999999999989342 ) ) ;
#3516=CARTESIAN_POINT ( 'NONE',  ( 25.06647319987872535, 3.604726614523236616, 168.1169290841567090 ) ) ;
#3519=ADVANCED_FACE ( 'NONE', ( #8684 ), #14560, .T. ) ;
#3524=DIRECTION ( 'NONE',  ( 0.000000000000000000, 0.000000000000000000, 1.000000000000000000 ) ) ;
#3526=CARTESIAN_POINT ( 'NONE',  ( 24.00000000000000000, -5.196152422706629359, -3.393749998770956289 ) ) ;
#3527=DIRECTION ( 'NONE',  ( 0.08715574274765150453, 0.000000000000000000, 0.9961946980917461003 ) ) ;
#3528=CARTESIAN_POINT ( 'NONE',  ( 26.75643035624999655, 7.049594010296217766E-16, -6.665624999385472371 ) ) ;
#3533=AXIS2_PLACEMENT_3D ( 'NONE', #32188, #12284, #905 ) ;
#3535=CARTESIAN_POINT ( 'NONE',  ( 26.97716818855048260, 0.000000000000000000, 49.47706554351410801 ) ) ;
#3536=CARTESIAN_POINT ( 'NONE',  ( 29.48996426250578295, 6.148716598298411107, 159.4803050314378368 ) ) ;
#3539=ADVANCED_FACE ( 'NONE', ( #330 ), #8320, .T. ) ;
#3542=CARTESIAN_POINT ( 'NONE',  ( 24.81151116879471630, 3.464101615137512358, 162.4080514859152231 ) ) ;
#3550=CARTESIAN_POINT ( 'NONE',  ( 26.09447537722126498, 2.706287405489508746, -7.999999999999998224 ) ) ;
#3552=CARTESIAN_POINT ( 'NONE',  ( 25.06483902970220967, 0.000000000000000000, 168.0982504335675287 ) ) ;
#3561=CARTESIAN_POINT ( 'NONE',  ( 33.97336387291019122, 5.196152422706631135, 163.8650878731170906 ) ) ;
#3563=ORIENTED_EDGE ( 'NONE', *, *, #11960, .T. ) ;
#3564=CARTESIAN_POINT ( 'NONE',  ( 26.99999999999999645, 3.464101615137755275, -0.1875000000000169031 ) ) ;
#3566=CARTESIAN_POINT ( 'NONE',  ( 34.18538171151332961, 5.407089921784862696, 164.8911387336007408 ) ) ;
#3568=CARTESIAN_POINT ( 'NONE',  ( 24.97492818644699142, -3.464101615137761048, 164.2759165448372016 ) ) ;
#3579=CARTESIAN_POINT ( 'NONE',  ( 15.24356964374999990, 0.000000000000000000, -4.753124999385488714 ) ) ;
#3589=CARTESIAN_POINT ( 'NONE',  ( 26.99999999999999645, 7.347880794884117764E-16, -0.6187499987709565996 ) ) ;
#3594=CARTESIAN_POINT ( 'NONE',  ( 27.82012958953286130, 5.407089921784856479, 163.7729017808578362 ) ) ;
#3600=CARTESIAN_POINT ( 'NONE',  ( 15.00000000000000000, 0.000000000000000000, -4.443749998770951670 ) ) ;
#3604=ORIENTED_EDGE ( 'NONE', *, *, #6147, .F. ) ;
#3605=CARTESIAN_POINT ( 'NONE',  ( 34.30794447475221176, 5.407089921784857367, 166.2920375277922460 ) ) ;
#3606=CARTESIAN_POINT ( 'NONE',  ( 15.24356964374999990, 3.323476615752268604, -3.328124999385480898 ) ) ;
#3609=CARTESIAN_POINT ( 'NONE',  ( 20.99999999999999645, 6.928203230275506996, -3.712500000000020339 ) ) ;
#3611=CARTESIAN_POINT ( 'NONE',  ( 24.00000000000000000, -5.196152422706629359, -7.443749998770954335 ) ) ;
#3619=CARTESIAN_POINT ( 'NONE',  ( 26.75643035624999655, -3.323476615752267715, -2.203124999385475569 ) ) ;
#3621=CARTESIAN_POINT ( 'NONE',  ( 23.99999999999999645, 5.196152422706631135, -7.743749998770948828 ) ) ;
#3625=CARTESIAN_POINT ( 'NONE',  ( 30.90225418466721408, -7.209453229046482114, 163.1832832459922713 ) ) ;
#3633=CARTESIAN_POINT ( 'NONE',  ( 24.95208128752243226, 0.000000000000000000, 166.8094235429113041 ) ) ;
#3658=CARTESIAN_POINT ( 'NONE',  ( 24.39973176785919406, 3.604726614523236616, 160.4960396437548411 ) ) ;
#3659=CARTESIAN_POINT ( 'NONE',  ( 15.24356964374999990, 3.323476615752268604, -5.690624999385482496 ) ) ;
#3663=AXIS2_PLACEMENT_3D ( 'NONE', #29610, #21659, #33212 ) ;
#3665=CARTESIAN_POINT ( 'NONE',  ( 26.75643035624999655, -3.323476615752267271, -5.803124999385441463 ) ) ;
#3666=CARTESIAN_POINT ( 'NONE',  ( 36.59589384753738273, 3.464101615138219348, 159.4196029116645548 ) ) ;
#3673=CARTESIAN_POINT ( 'NONE',  ( 24.58599568454271278, 3.464101615137752166, 159.8303977058271244 ) ) ;
#3679=CARTESIAN_POINT ( 'NONE',  ( 18.12178482187499640, 4.985214923628404904, -6.628124999385476279 ) ) ;
#3699=CARTESIAN_POINT ( 'NONE',  ( 23.99999999999999645, 5.196152422706631135, -6.899999999999989697 ) ) ;
#3703=CARTESIAN_POINT ( 'NONE',  ( 24.95208128752243226, 0.000000000000000000, 166.8094235429113041 ) ) ;
#3704=PLANE ( 'NONE',  #32296 ) ;
#3706=EDGE_LOOP ( 'NONE', ( #7520, #19620, #27501, #25106 ) ) ;
#3712=CARTESIAN_POINT ( 'NONE',  ( 18.12178482187499640, 4.985214923628404904, -7.415624999385473259 ) ) ;
#3715=LINE ( 'NONE', #27030, #1238 ) ;
#3719=CARTESIAN_POINT ( 'NONE',  ( 37.34761212884377812, 7.347880794884117764E-16, 168.0117821839301087 ) ) ;
#3723=CARTESIAN_POINT ( 'NONE',  ( 23.87821517812499650, 4.985214923628404904, -0.4031249993854957303 ) ) ;
#3727=ORIENTED_EDGE ( 'NONE', *, *, #35816, .T. ) ;
#3730=CARTESIAN_POINT ( 'NONE',  ( 15.00000000000000000, 0.000000000000000000, -7.649999999999989697 ) ) ;
#3731=CARTESIAN_POINT ( 'NONE',  ( 31.42927406654086298, -6.928203230275514990, 169.2071480604035685 ) ) ;
#3732=CARTESIAN_POINT ( 'NONE',  ( 25.02888728581879718, -3.604726614523244610, 167.6873201206046815 ) ) ;
#3740=CARTESIAN_POINT ( 'NONE',  ( 30.98804811898798661, 6.928203230275506996, 164.1639124025385001 ) ) ;
#3744=CARTESIAN_POINT ( 'NONE',  ( 15.24356964374999990, 3.323476615752268604, -9.628124999385486049 ) ) ;
#3746=CARTESIAN_POINT ( 'NONE',  ( 37.28875051894242887, 7.646167579472024665E-16, 164.5443426563950027 ) ) ;
#3747=CARTESIAN_POINT ( 'NONE',  ( 27.96678062107526941, -5.196152422706638241, 164.0518066177726553 ) ) ;
#3748=CARTESIAN_POINT ( 'NONE',  ( 31.13512343476753585, 6.928203230275514990, 165.8449909543439560 ) ) ;
#3755=ORIENTED_EDGE ( 'NONE', *, *, #23969, .T. ) ;
#3759=CARTESIAN_POINT ( 'NONE',  ( 15.24356964374999990, 0.000000000000000000, -3.403124999385470417 ) ) ;
#3773=CYLINDRICAL_SURFACE ( 'NONE', #31872, 6.000000000000001776 ) ;
#3774=CARTESIAN_POINT ( 'NONE',  ( 37.21848120135211957, 3.604726614523238837, 163.7411606810585170 ) ) ;
#3780=CARTESIAN_POINT ( 'NONE',  ( 27.00000000000018474, -3.464101615137644696, -4.256249998770928578 ) ) ;
#3785=CARTESIAN_POINT ( 'NONE',  ( 25.06974154023176382, 0.000000000000000000, 168.1542863853351548 ) ) ;
#3786=CARTESIAN_POINT ( 'NONE',  ( 15.24356964374999990, 0.000000000000000000, -1.940624999385465177 ) ) ;
#3791=DIRECTION ( 'NONE',  ( 0.08715574274765150453, 0.000000000000000000, 0.9961946980917461003 ) ) ;
#3798=CARTESIAN_POINT ( 'NONE',  ( 23.87821517812499650, 4.985214923628404904, -2.090624999385476634 ) ) ;
#3800=CARTESIAN_POINT ( 'NONE',  ( 23.99999999999999645, 5.196152422706631135, -8.193749998770954335 ) ) ;
#3808=CARTESIAN_POINT ( 'NONE',  ( 37.24953043470598146, 7.646167579472024665E-16, 164.0960550422537096 ) ) ;
#3813=DIRECTION ( 'NONE',  ( 0.08715574274765150453, 0.000000000000000000, 0.9961946980917461003 ) ) ;
#3815=LINE ( 'NONE', #32062, #11502 ) ;
#3816=CARTESIAN_POINT ( 'NONE',  ( 31.22091736908830839, -7.209453229046475009, 166.8256201108902133 ) ) ;
#3817=VERTEX_POINT ( 'NONE', #32924 ) ;
#3835=DIRECTION ( 'NONE',  ( 0.000000000000000000, 0.000000000000000000, 1.000000000000000000 ) ) ;
#3836=CARTESIAN_POINT ( 'NONE',  ( 15.70715912503073142, 2.547338863122542651, -8.000000000000005329 ) ) ;
#3846=CARTESIAN_POINT ( 'NONE',  ( 23.87821517812499650, 4.985214923628404904, -4.003124999385487826 ) ) ;
#3849=AXIS2_PLACEMENT_3D ( 'NONE', #13163, #4809, #19425 ) ;
#3851=CARTESIAN_POINT ( 'NONE',  ( 26.75643035624999655, -3.323476615752267271, -7.153124999385460647 ) ) ;
#3854=EDGE_CURVE ( 'NONE', #31979, #9957, #26863, .T. ) ;
#3860=CARTESIAN_POINT ( 'NONE',  ( 33.65960319901864040, 5.196152422706631135, 160.2787869599868316 ) ) ;
#3865=CARTESIAN_POINT ( 'NONE',  ( 20.99999999999999645, -6.646953231504538984, -6.440624999385486937 ) ) ;
#3866=DIRECTION ( 'NONE',  ( 1.000000000000000000, 0.000000000000000000, 0.000000000000000000 ) ) ;
#3873=CARTESIAN_POINT ( 'NONE',  ( 36.89654967657799745, 7.646167579472024665E-16, 160.0614665149821576 ) ) ;
#3885=CARTESIAN_POINT ( 'NONE',  ( 15.00000000000000178, -3.464101615137757051, -7.162499999999998757 ) ) ;
#3892=CARTESIAN_POINT ( 'NONE',  ( 37.17599277676264080, 7.646167579472015790E-16, 163.2555157657388065 ) ) ;
#3901=CARTESIAN_POINT ( 'NONE',  ( 18.12178482187499640, 4.985214923628404904, -9.215624999385468641 ) ) ;
#3905=CARTESIAN_POINT ( 'NONE',  ( 24.86380461455084756, 0.000000000000000000, 163.0057683059945930 ) ) ;
#3908=CARTESIAN_POINT ( 'NONE',  ( 31.26258870864309003, 6.928203230275506996, 167.3019257015274945 ) ) ;
#3920=LINE ( 'NONE', #36312, #31394 ) ;
#3921=CARTESIAN_POINT ( 'NONE',  ( 34.38148213269554532, 5.407089921784862696, 167.1325768043071776 ) ) ;
#3934=CARTESIAN_POINT ( 'NONE',  ( 33.79808337967844523, 5.407089921784857367, 160.4642985439555218 ) ) ;
#3935=CARTESIAN_POINT ( 'NONE',  ( 21.00000000000000000, -6.646953231504538984, -9.028124999385470417 ) ) ;
#3937=CARTESIAN_POINT ( 'NONE',  ( 28.05054758442196672, 5.407089921784862696, 166.4065915139379115 ) ) ;
#3938=CARTESIAN_POINT ( 'NONE',  ( 24.92917142150447063, 3.464101615137757051, 163.7529143283390169 ) ) ;
#3949=CARTESIAN_POINT ( 'NONE',  ( 18.12178482187499640, 4.985214923628404904, -7.078124999385481786 ) ) ;
#3956=( BOUNDED_CURVE ( )  B_SPLINE_CURVE ( 2, ( #12177, #35290, #9346, #20917, #22226, #10278, #25242 ),
 .UNSPECIFIED., .F., .F. ) 
 B_SPLINE_CURVE_WITH_KNOTS ( ( 3, 2, 2, 3 ),
 ( 0.8478260869565228397, 0.8550724637681171858, 0.8623188405797115319, 0.8695652173913057670 ),
 .UNSPECIFIED. ) 
 CURVE ( )  GEOMETRIC_REPRESENTATION_ITEM ( )  RATIONAL_B_SPLINE_CURVE ( ( 0.9999999999999794609, 0.8660254037844592467, 1.000000000000000000, 0.8660254037844387076, 1.000000000000000000, 0.8660254037844120623, 1.000000000000026645 ) ) 
 REPRESENTATION_ITEM ( '' )  );
#3958=CYLINDRICAL_SURFACE ( 'NONE', #2839, 6.000000000000001776 ) ;
#3960=CARTESIAN_POINT ( 'NONE',  ( 15.00000000000063771, -3.464101615138124757, -3.112499999999997158 ) ) ;
#3964=CARTESIAN_POINT ( 'NONE',  ( 27.91164311941789933, -5.407089921784859143, 164.8189062138541772 ) ) ;
#3976=CARTESIAN_POINT ( 'NONE',  ( 25.10569328411516921, 3.604726614523236616, 168.5652166982980305 ) ) ;
#3977=CARTESIAN_POINT ( 'NONE',  ( 26.75643035624999655, 3.323476615752271712, -3.028124999385441107 ) ) ;
#3980=CARTESIAN_POINT ( 'NONE',  ( 26.99999999999999645, 7.347880794884117764E-16, -2.475000000000004974 ) ) ;
#3981=CARTESIAN_POINT ( 'NONE',  ( 18.00000000000000000, 5.196152422706630247, -3.168749998770953091 ) ) ;
#3986=ORIENTED_EDGE ( 'NONE', *, *, #19589, .F. ) ;
#3989=CARTESIAN_POINT ( 'NONE',  ( 26.75643035624999655, -3.323476615752267715, -2.653124999385471305 ) ) ;
#3991=CARTESIAN_POINT ( 'NONE',  ( 18.00000000000000355, -5.196152422706632912, -10.21874999877095469 ) ) ;
#3998=CARTESIAN_POINT ( 'NONE',  ( 37.17109026623309376, 7.646167579472024665E-16, 163.1994798139711520 ) ) ;
#4006=CARTESIAN_POINT ( 'NONE',  ( 28.18618370907300275, -5.407089921784859143, 167.9569195128432000 ) ) ;
#4011=( BOUNDED_CURVE ( )  B_SPLINE_CURVE ( 2, ( #22876, #17188, #290, #5603, #11856, #34977, #8835 ),
 .UNSPECIFIED., .F., .F. ) 
 B_SPLINE_CURVE_WITH_KNOTS ( ( 3, 2, 2, 3 ),
 ( 0.2826086956521731142, 0.2898550724637674603, 0.2971014492753617509, 0.3043478260869560970 ),
 .UNSPECIFIED. ) 
 CURVE ( )  GEOMETRIC_REPRESENTATION_ITEM ( )  RATIONAL_B_SPLINE_CURVE ( ( 1.000000000000014433, 0.8660254037844243857, 1.000000000000000000, 0.8660254037844387076, 1.000000000000000000, 0.8660254037844469233, 0.9999999999999917843 ) ) 
 REPRESENTATION_ITEM ( '' )  );
#4018=ORIENTED_EDGE ( 'NONE', *, *, #22396, .T. ) ;
#4028=DIRECTION ( 'NONE',  ( 0.08715574274765150453, 0.000000000000000000, 0.9961946980917461003 ) ) ;
#4035=CARTESIAN_POINT ( 'NONE',  ( 21.00000000000000000, -6.646953231504538984, -5.090624999385466865 ) ) ;
#4037=EDGE_CURVE ( 'NONE', #22329, #4445, #17973, .T. ) ;
#4039=CARTESIAN_POINT ( 'NONE',  ( 18.12178482187500350, -4.985214923628407568, -7.715624999385467753 ) ) ;
#4046=CARTESIAN_POINT ( 'NONE',  ( 36.63838227223477872, -3.464101615137751278, 159.9052478282085303 ) ) ;
#4050=CARTESIAN_POINT ( 'NONE',  ( 26.75643035624999655, 3.323476615752271268, -5.840624999385470417 ) ) ;
#4060=CARTESIAN_POINT ( 'NONE',  ( 38.16802127826974100, 7.686353184319911769, 158.6159210646234783 ) ) ;
#4061=ORIENTED_EDGE ( 'NONE', *, *, #8048, .T. ) ;
#4069=CARTESIAN_POINT ( 'NONE',  ( 23.34314575050770202, 3.999999999999897859, 49.79500130984166617 ) ) ;
#4075=CARTESIAN_POINT ( 'NONE',  ( 15.00000000000000000, 0.000000000000000000, -7.649999999999989697 ) ) ;
#4080=CARTESIAN_POINT ( 'NONE',  ( 27.95086320365434318, -5.407089921784859143, 165.2671938279954702 ) ) ;
#4089=CARTESIAN_POINT ( 'NONE',  ( 18.00000000000000355, -5.196152422706632912, -1.274999999999998357 ) ) ;
#4091=CARTESIAN_POINT ( 'NONE',  ( 18.12178482187500350, -4.985214923628407568, -9.065624999385457627 ) ) ;
#4098=DIRECTION ( 'NONE',  ( 0.08715574274765150453, 0.000000000000000000, 0.9961946980917461003 ) ) ;
#4099=CARTESIAN_POINT ( 'NONE',  ( 28.31649303895732928, 5.196152422706630247, 168.0490378450901687 ) ) ;
#4105=AXIS2_PLACEMENT_3D ( 'NONE', #32264, #25832, #37379 ) ;
#4113=CARTESIAN_POINT ( 'NONE',  ( 31.25523494279520165, -7.209453229046482114, 167.2178717732638233 ) ) ;
#4125=ORIENTED_EDGE ( 'NONE', *, *, #17246, .T. ) ;
#4126=CARTESIAN_POINT ( 'NONE',  ( 18.00000000000000355, -5.196152422706632912, -6.168749998770955756 ) ) ;
#4127=EDGE_LOOP ( 'NONE', ( #7309, #1381, #30410, #24410 ) ) ;
#4129=CARTESIAN_POINT ( 'NONE',  ( 24.00000000000000000, -5.196152422706629359, -0.7500000000000006661 ) ) ;
#4130=CARTESIAN_POINT ( 'NONE',  ( 37.18419511108445619, 3.464101615137973766, 166.1439171237837513 ) ) ;
#4131=CARTESIAN_POINT ( 'NONE',  ( 37.13513852234969193, 3.604726614523243278, 162.7885495010082764 ) ) ;
#4132=CARTESIAN_POINT ( 'NONE',  ( 27.83604700695378398, 5.196152422706636465, 162.5575145706350781 ) ) ;
#4142=CARTESIAN_POINT ( 'NONE',  ( 18.12178482187500350, -4.985214923628407568, -6.928124999385470772 ) ) ;
#4157=CARTESIAN_POINT ( 'NONE',  ( 24.68080903822037087, -3.604726614523240613, 163.7087675451007271 ) ) ;
#4168=CARTESIAN_POINT ( 'NONE',  ( 34.25565102910361759, -5.407089921784855591, 165.6943207089371981 ) ) ;
#4169=CARTESIAN_POINT ( 'NONE',  ( 26.75643035624999655, -3.323476615752267715, -3.553124999385494753 ) ) ;
#4171=CARTESIAN_POINT ( 'NONE',  ( 36.98482634954957859, 7.347880794884125653E-16, 163.8651217518988688 ) ) ;
#4172=CARTESIAN_POINT ( 'NONE',  ( 34.38190641693269356, -5.196152422706635576, 168.5347505191977859 ) ) ;
#4173=DIRECTION ( 'NONE',  ( 0.08715574274765150453, 0.000000000000000000, 0.9961946980917461003 ) ) ;
#4178=VERTEX_POINT ( 'NONE', #1832 ) ;
#4181=CARTESIAN_POINT ( 'NONE',  ( 15.24356964374999990, 3.323476615752268604, -1.528124999385498173 ) ) ;
#4184=CARTESIAN_POINT ( 'NONE',  ( 23.87821517812499650, 4.985214923628404904, -0.4031249993854957303 ) ) ;
#4190=CARTESIAN_POINT ( 'NONE',  ( 27.78908035617901717, -5.407089921784865361, 163.4180074196626720 ) ) ;
#4195=CARTESIAN_POINT ( 'NONE',  ( 37.37536153829788077, 3.604726614523238837, 165.5343111376236607 ) ) ;
#4196=VERTEX_POINT ( 'NONE', #4671 ) ;
#4198=CARTESIAN_POINT ( 'NONE',  ( 20.99999999999999645, -6.928203230275506996, -5.287499999999990763 ) ) ;
#4205=EDGE_LOOP ( 'NONE', ( #21903, #16404, #32468, #17665, #13665 ) ) ;
#4214=DIRECTION ( 'NONE',  ( 0.000000000000000000, 0.000000000000000000, 1.000000000000000000 ) ) ;
#4221=CARTESIAN_POINT ( 'NONE',  ( 18.12178482187499640, 4.985214923628404904, -3.478124999385490135 ) ) ;
#4224=ORIENTED_EDGE ( 'NONE', *, *, #14456, .F. ) ;
#4231=( BOUNDED_CURVE ( )  B_SPLINE_CURVE ( 2, ( #32123, #5784, #34231, #14145, #25882, #5409, #2941 ),
 .UNSPECIFIED., .F., .F. ) 
 B_SPLINE_CURVE_WITH_KNOTS ( ( 3, 2, 2, 3 ),
 ( 0.3913043478260868069, 0.3985507246376810975, 0.4057971014492754436, 0.4130434782608697342 ),
 .UNSPECIFIED. ) 
 CURVE ( )  GEOMETRIC_REPRESENTATION_ITEM ( )  RATIONAL_B_SPLINE_CURVE ( ( 1.000000000000003109, 0.8660254037844357100, 1.000000000000000000, 0.8660254037844387076, 1.000000000000000000, 0.8660254037844355990, 1.000000000000003109 ) ) 
 REPRESENTATION_ITEM ( '' )  );
#4236=DIRECTION ( 'NONE',  ( 1.000000000000000000, 0.000000000000000000, 0.000000000000000000 ) ) ;
#4237=DIRECTION ( 'NONE',  ( 0.9961946980917462113, 0.000000000000000000, -0.08715574274765118534 ) ) ;
#4247=VERTEX_POINT ( 'NONE', #16254 ) ;
#4251=CARTESIAN_POINT ( 'NONE',  ( 36.82467767225140420, -3.464101615137388013, 162.0346139941552508 ) ) ;
#4263=CARTESIAN_POINT ( 'NONE',  ( 34.21643094486717729, -5.407089921784855591, 165.2460330947959051 ) ) ;
#4266=EDGE_CURVE ( 'NONE', #32003, #30542, #13215, .T. ) ;
#4269=ORIENTED_EDGE ( 'NONE', *, *, #629, .T. ) ;
#4274=CARTESIAN_POINT ( 'NONE',  ( 23.99999999999999645, 5.196152422706631135, -6.000000000000005329 ) ) ;
#4275=CARTESIAN_POINT ( 'NONE',  ( 23.87821517812499650, 4.985214923628404904, -9.740624999385467220 ) ) ;
#4282=CARTESIAN_POINT ( 'NONE',  ( 37.11229162342512211, 7.347880794884117764E-16, 165.3220564990824073 ) ) ;
#4292=ADVANCED_FACE ( 'NONE', ( #4491 ), #4860, .T. ) ;
#4293=EDGE_LOOP ( 'NONE', ( #6512, #33594, #114, #10757 ) ) ;
#4296=CARTESIAN_POINT ( 'NONE',  ( 24.75107835581066240, 0.000000000000000000, 164.5119495204372413 ) ) ;
#4303=CARTESIAN_POINT ( 'NONE',  ( 21.00000000000000355, 0.000000000000000000, 50.00000000000001421 ) ) ;
#4311=CARTESIAN_POINT ( 'NONE',  ( 15.00000000000000000, 0.000000000000000000, -1.799999999999996048 ) ) ;
#4313=CARTESIAN_POINT ( 'NONE',  ( 24.75107835581066240, 0.000000000000000000, 164.5119495204372413 ) ) ;
#4314=CARTESIAN_POINT ( 'NONE',  ( 33.79360515338605353, -5.196152422706635576, 161.8104363070785041 ) ) ;
#4321=ORIENTED_EDGE ( 'NONE', *, *, #23832, .F. ) ;
#4323=FACE_OUTER_BOUND ( 'NONE', #36129, .T. ) ;
#4325=CARTESIAN_POINT ( 'NONE',  ( 21.00000000000000000, -6.646953231504538984, -6.440624999385486049 ) ) ;
#4338=CARTESIAN_POINT ( 'NONE',  ( 24.83768937516614272, -3.604726614523240613, 165.5019180016658993 ) ) ;
#4341=CARTESIAN_POINT ( 'NONE',  ( 18.00000000000000355, -5.196152422706632912, -3.918749998770953979 ) ) ;
#4342=CARTESIAN_POINT ( 'NONE',  ( 29.51299565928205482, 6.068759932216711839, 159.5818089612911024 ) ) ;
#4350=CARTESIAN_POINT ( 'NONE',  ( 37.25770128558855987, 3.604726614523238837, 164.1894482951998100 ) ) ;
#4351=CARTESIAN_POINT ( 'NONE',  ( 26.75643035624999655, -3.323476615752267715, -4.003124999385458516 ) ) ;
#4353=CARTESIAN_POINT ( 'NONE',  ( 25.36712902881142284, -3.464101615137761048, 168.7587926862500467 ) ) ;
#4359=VERTEX_POINT ( 'NONE', #10923 ) ;
#4364=EDGE_CURVE ( 'NONE', #22619, #29003, #35223, .T. ) ;
#4365=CARTESIAN_POINT ( 'NONE',  ( 18.12178482187499640, 4.985214923628404904, -2.915624999385468819 ) ) ;
#4368=CARTESIAN_POINT ( 'NONE',  ( 15.00000000000000000, 0.000000000000000000, -9.843749998770940479 ) ) ;
#4374=CARTESIAN_POINT ( 'NONE',  ( 30.86303410043077022, -7.209453229046482114, 162.7349956318509783 ) ) ;
#4375=EDGE_CURVE ( 'NONE', #7924, #6128, #11760, .T. ) ;
#4384=CYLINDRICAL_SURFACE ( 'NONE', #12489, 6.000000000000001776 ) ;
#4399=FACE_OUTER_BOUND ( 'NONE', #4127, .T. ) ;
#4400=DIRECTION ( 'NONE',  ( 0.000000000000000000, 0.000000000000000000, 1.000000000000000000 ) ) ;
#4402=ORIENTED_EDGE ( 'NONE', *, *, #2381, .F. ) ;
#4407=CARTESIAN_POINT ( 'NONE',  ( 23.87821517812499650, 4.985214923628404904, -5.353124999385477700 ) ) ;
#4411=CARTESIAN_POINT ( 'NONE',  ( 26.60793733450167053, 1.299049382686714882, -8.000000000000000000 ) ) ;
#4419=CARTESIAN_POINT ( 'NONE',  ( 24.71019261795811772, -3.464101615137757051, 161.2499751506078667 ) ) ;
#4428=CYLINDRICAL_SURFACE ( 'NONE', #11372, 6.000000000000001776 ) ;
#4445=VERTEX_POINT ( 'NONE', #28905 ) ;
#4449=CARTESIAN_POINT ( 'NONE',  ( 37.13350435217316203, -3.604726614523235284, 162.7698708504190677 ) ) ;
#4457=LINE ( 'NONE', #1424, #25577 ) ;
#4459=( BOUNDED_CURVE ( )  B_SPLINE_CURVE ( 2, ( #28654, #34716, #22985, #6092, #5528, #26372, #28840 ),
 .UNSPECIFIED., .F., .F. ) 
 B_SPLINE_CURVE_WITH_KNOTS ( ( 3, 2, 2, 3 ),
 ( 0.08695652173913032135, 0.09420289855072443153, 0.1014492753623185417, 0.1086956521739126380 ),
 .UNSPECIFIED. ) 
 CURVE ( )  GEOMETRIC_REPRESENTATION_ITEM ( )  RATIONAL_B_SPLINE_CURVE ( ( 1.000000000000001998, 0.8660254037844367092, 1.000000000000000000, 0.8660254037844387076, 1.000000000000000000, 0.8660254037844461461, 0.9999999999999925615 ) ) 
 REPRESENTATION_ITEM ( '' )  );
#4461=CARTESIAN_POINT ( 'NONE',  ( 15.00000000000000000, 0.000000000000000000, -4.500000000000003553 ) ) ;
#4462=CARTESIAN_POINT ( 'NONE',  ( 26.75643035624999655, -3.323476615752267715, -8.503124999385478944 ) ) ;
#4466=CARTESIAN_POINT ( 'NONE',  ( 27.84585202812001015, 5.196152422706630247, 162.6695864753947660 ) ) ;
#4468=CARTESIAN_POINT ( 'NONE',  ( 15.00000000000001954, -11.99999999999999822, 50.26196565745151190 ) ) ;
#4469=CARTESIAN_POINT ( 'NONE',  ( 34.20868437832884013, 5.196152422706631135, 166.5548135579648488 ) ) ;
#4474=CARTESIAN_POINT ( 'NONE',  ( 15.24356964374999990, 0.000000000000000000, -1.153124999385496396 ) ) ;
#4479=CARTESIAN_POINT ( 'NONE',  ( 31.24297866652485922, -6.928203230275506996, 167.0777818944568480 ) ) ;
#4480=CARTESIAN_POINT ( 'NONE',  ( 21.00000000000000355, 0.000000000000000000, 50.00000000000001421 ) ) ;
#4481=EDGE_CURVE ( 'NONE', #19092, #11864, #4231, .T. ) ;
#4484=CARTESIAN_POINT ( 'NONE',  ( 31.00030439525832193, 7.209453229046482114, 164.3040022813455039 ) ) ;
#4491=FACE_OUTER_BOUND ( 'NONE', #25254, .T. ) ;
#4499=CYLINDRICAL_SURFACE ( 'NONE', #1508, 5.999999999999994671 ) ;
#4500=ORIENTED_EDGE ( 'NONE', *, *, #22553, .F. ) ;
#4501=CARTESIAN_POINT ( 'NONE',  ( 18.00000000000000355, -5.196152422706632912, -3.074999999999994404 ) ) ;
#4502=CARTESIAN_POINT ( 'NONE',  ( 37.17109026623309376, 7.646167579472024665E-16, 163.1994798139711520 ) ) ;
#4503=CARTESIAN_POINT ( 'NONE',  ( 36.71028575989448228, 7.347880794884125653E-16, 160.7271084529098744 ) ) ;
#4515=CARTESIAN_POINT ( 'NONE',  ( 23.87821517812499650, 4.985214923628404904, -6.253124999385489602 ) ) ;
#4519=CARTESIAN_POINT ( 'NONE',  ( 37.41951561650326852, 3.464101615137893386, 168.8336428086315095 ) ) ;
#4529=CARTESIAN_POINT ( 'NONE',  ( 37.06160086440634416, 3.604726614523238837, 161.9480102244933732 ) ) ;
#4539=CARTESIAN_POINT ( 'NONE',  ( 31.06403703214253653, -7.209453229046475009, 165.0324696543250411 ) ) ;
#4540=CARTESIAN_POINT ( 'NONE',  ( 26.75643035624999655, 3.323476615752271712, -4.378124999385460292 ) ) ;
#4542=ADVANCED_FACE ( 'NONE', ( #8274 ), #11657, .T. ) ;
#4543=CARTESIAN_POINT ( 'NONE',  ( 37.41297893579741896, -3.464101615137755275, 168.7589282062745610 ) ) ;
#4547=AXIS2_PLACEMENT_3D ( 'NONE', #25714, #19863, #111 ) ;
#4551=VERTEX_POINT ( 'NONE', #16991 ) ;
#4555=CARTESIAN_POINT ( 'NONE',  ( 26.75643035624999655, -3.323476615752267715, -4.453124999385455141 ) ) ;
#4557=CARTESIAN_POINT ( 'NONE',  ( 15.00000000000000000, 3.464101615137752166, -8.981249998770968190 ) ) ;
#4563=CARTESIAN_POINT ( 'NONE',  ( 36.89328133622495898, -3.604726614523238837, 160.0241092138036834 ) ) ;
#4566=( LENGTH_UNIT ( ) NAMED_UNIT ( * ) SI_UNIT ( .MILLI., .METRE. ) );
#4572=AXIS2_PLACEMENT_3D ( 'NONE', #26454, #29864, #27025 ) ;
#4581=ORIENTED_EDGE ( 'NONE', *, *, #28607, .F. ) ;
#4587=CARTESIAN_POINT ( 'NONE',  ( 26.99999999999999645, 7.347880794884117764E-16, -6.525000000000003020 ) ) ;
#4589=CARTESIAN_POINT ( 'NONE',  ( 33.98970557456826214, -5.196152422706635576, 164.0518743777849409 ) ) ;
#4592=ORIENTED_EDGE ( 'NONE', *, *, #7163, .T. ) ;
#4597=CARTESIAN_POINT ( 'NONE',  ( 26.75643035624999655, -3.323476615752267715, -8.165624999385475036 ) ) ;
#4600=CARTESIAN_POINT ( 'NONE',  ( 23.87821517812499650, 4.985214923628404904, -6.590624999385480187 ) ) ;
#4602=CARTESIAN_POINT ( 'NONE',  ( 37.59924285248093412, -3.604726614523238837, 168.0932862683468443 ) ) ;
#4612=( BOUNDED_CURVE ( )  B_SPLINE_CURVE ( 2, ( #7079, #32835, #6879, #15792, #27156, #29997, #9727 ),
 .UNSPECIFIED., .F., .F. ) 
 B_SPLINE_CURVE_WITH_KNOTS ( ( 3, 2, 2, 3 ),
 ( 0.7826086956521727256, 0.7898550724637667386, 0.7971014492753607517, 0.8043478260869548757 ),
 .UNSPECIFIED. ) 
 CURVE ( )  GEOMETRIC_REPRESENTATION_ITEM ( )  RATIONAL_B_SPLINE_CURVE ( ( 1.000000000000022649, 0.8660254037844161701, 1.000000000000000000, 0.8660254037844387076, 1.000000000000000000, 0.8660254037844694608, 0.9999999999999692468 ) ) 
 REPRESENTATION_ITEM ( '' )  );
#4624=CARTESIAN_POINT ( 'NONE',  ( 31.11551339264930860, -6.928203230275514990, 165.6208471472733095 ) ) ;
#4635=CARTESIAN_POINT ( 'NONE',  ( 31.06403703214253653, -7.209453229046475009, 165.0324696543250411 ) ) ;
#4642=CARTESIAN_POINT ( 'NONE',  ( 18.00000000000000000, 5.196152422706630247, -5.418749998770955756 ) ) ;
#4644=CARTESIAN_POINT ( 'NONE',  ( 27.00000000000036593, 3.464101615137540779, -4.687500000000010658 ) ) ;
#4645=CARTESIAN_POINT ( 'NONE',  ( 15.24356964374999990, 3.323476615752268604, -8.728124999385462601 ) ) ;
#4651=DIRECTION ( 'NONE',  ( 0.000000000000000000, 0.000000000000000000, 1.000000000000000000 ) ) ;
#4652=CARTESIAN_POINT ( 'NONE',  ( 31.14492845593375847, 6.928203230275506996, 165.9570628591036439 ) ) ;
#4656=CARTESIAN_POINT ( 'NONE',  ( 15.24356964374999990, 0.000000000000000000, -2.953124999385492444 ) ) ;
#4666=CARTESIAN_POINT ( 'NONE',  ( 34.10694154304044901, 5.407089921784862696, 163.9945635053181547 ) ) ;
#4671=CARTESIAN_POINT ( 'NONE',  ( 36.90638618107669799, 7.347880794884125653E-16, 162.9685465236163111 ) ) ;
#4677=DIRECTION ( 'NONE',  ( 0.08715574274765150453, 0.000000000000000000, 0.9961946980917461003 ) ) ;
#4682=CARTESIAN_POINT ( 'NONE',  ( 21.00000000000000000, 6.928203230275506996, -1.912500000000006084 ) ) ;
#4683=( BOUNDED_CURVE ( )  B_SPLINE_CURVE ( 2, ( #30317, #36175, #10221, #21795, #4341, #15921, #33348 ),
 .UNSPECIFIED., .F., .F. ) 
 B_SPLINE_CURVE_WITH_KNOTS ( ( 3, 2, 2, 3 ),
 ( 0.3260869565217381361, 0.3333333333333324267, 0.3405797101449267172, 0.3478260869565210078 ),
 .UNSPECIFIED. ) 
 CURVE ( )  GEOMETRIC_REPRESENTATION_ITEM ( )  RATIONAL_B_SPLINE_CURVE ( ( 1.000000000000018430, 0.8660254037844202779, 1.000000000000000000, 0.8660254037844387076, 1.000000000000000000, 0.8660254037844520303, 0.9999999999999866773 ) ) 
 REPRESENTATION_ITEM ( '' )  );
#4684=CARTESIAN_POINT ( 'NONE',  ( 27.71064018770612947, -5.407089921784865361, 162.5214321913800859 ) ) ;
#4685=CARTESIAN_POINT ( 'NONE',  ( 24.85399959338462139, 0.000000000000000000, 162.8936964012349051 ) ) ;
#4693=CARTESIAN_POINT ( 'NONE',  ( 27.00000000000018474, -3.464101615137644696, -3.862499999999974953 ) ) ;
#4694=AXIS2_PLACEMENT_3D ( 'NONE', #5646, #19525, #28580 ) ;
#4696=EDGE_CURVE ( 'NONE', #27232, #16220, #28719, .T. ) ;
#4697=CARTESIAN_POINT ( 'NONE',  ( 26.75643035624999655, 7.049594010296217766E-16, -7.678124999385471661 ) ) ;
#4710=CARTESIAN_POINT ( 'NONE',  ( 24.48470861703815515, -3.604726614523240613, 161.4673294743943188 ) ) ;
#4711=CARTESIAN_POINT ( 'NONE',  ( 18.00000000000000000, 5.196152422706630247, -0.9187499987709513150 ) ) ;
#4713=CARTESIAN_POINT ( 'NONE',  ( 27.88834045260238526, -5.196152422706638241, 163.1552313894900976 ) ) ;
#4718=EDGE_CURVE ( 'NONE', #32501, #13274, #11111, .T. ) ;
#4723=CARTESIAN_POINT ( 'NONE',  ( 24.75924920669325502, -3.604726614523240613, 164.6053427733833416 ) ) ;
#4725=CARTESIAN_POINT ( 'NONE',  ( 26.75643035624999655, 7.049594010296217766E-16, -4.415624999385469707 ) ) ;
#4727=CARTESIAN_POINT ( 'NONE',  ( 15.08123753375185849, -0.4834061343151928591, -8.000000000000001776 ) ) ;
#4729=CARTESIAN_POINT ( 'NONE',  ( 25.39981243234178976, 3.464101615137757051, 169.1323656980344765 ) ) ;
#4730=CARTESIAN_POINT ( 'NONE',  ( 24.70038759679241736, -3.464101615138067469, 161.1379032458481788 ) ) ;
#4732=CARTESIAN_POINT ( 'NONE',  ( 36.99463137071579411, 7.347880794884117764E-16, 163.9771936566585566 ) ) ;
#4739=CARTESIAN_POINT ( 'NONE',  ( 23.87821517812499650, 4.985214923628404904, -4.790624999385456384 ) ) ;
#4743=CARTESIAN_POINT ( 'NONE',  ( 21.00000000000000000, 6.928203230275506996, -9.956249998770953624 ) ) ;
#4745=AXIS2_PLACEMENT_3D ( 'NONE', #5039, #19291, #16984 ) ;
#4767=CARTESIAN_POINT ( 'NONE',  ( 15.24356964374999990, 0.000000000000000000, -0.1968749993854768121 ) ) ;
#4772=DIRECTION ( 'NONE',  ( 0.08715574274765150453, 0.000000000000000000, 0.9961946980917461003 ) ) ;
#4783=CARTESIAN_POINT ( 'NONE',  ( 15.24356964374999990, 0.000000000000000000, -6.103124999385478588 ) ) ;
#4789=CARTESIAN_POINT ( 'NONE',  ( 31.39250523762275691, 7.209453229046482114, 168.7868784227583205 ) ) ;
#4795=CARTESIAN_POINT ( 'NONE',  ( 15.00000000000031797, 3.464101615137936019, -6.787500000000000533 ) ) ;
#4800=CARTESIAN_POINT ( 'NONE',  ( 26.99999999999999645, 7.347880794884117764E-16, -7.874999999999992895 ) ) ;
#4805=ORIENTED_EDGE ( 'NONE', *, *, #9600, .T. ) ;
#4807=LINE ( 'NONE', #25277, #10293 ) ;
#4809=DIRECTION ( 'NONE',  ( 0.000000000000000000, 0.000000000000000000, 1.000000000000000000 ) ) ;
#4816=VERTEX_POINT ( 'NONE', #18493 ) ;
#4820=CARTESIAN_POINT ( 'NONE',  ( 24.55661210480496948, 3.604726614523236616, 162.2891901003200132 ) ) ;
#4821=CARTESIAN_POINT ( 'NONE',  ( 18.12178482187500350, -4.985214923628407568, -0.6281249993854709501 ) ) ;
#4823=ORIENTED_EDGE ( 'NONE', *, *, #34019, .F. ) ;
#4827=CARTESIAN_POINT ( 'NONE',  ( 15.00000000000000000, 0.000000000000000000, -4.893749998770957177 ) ) ;
#4828=CARTESIAN_POINT ( 'NONE',  ( 26.75643035624999655, 7.049594010296217766E-16, -0.8156249993854780556 ) ) ;
#4829=CARTESIAN_POINT ( 'NONE',  ( 20.99999999999999645, -6.928203230275506996, -1.237499999999996270 ) ) ;
#4830=CARTESIAN_POINT ( 'NONE',  ( 26.99999999999999645, 7.347880794884117764E-16, -6.074999999999997513 ) ) ;
#4835=EDGE_CURVE ( 'NONE', #9824, #31631, #31140, .T. ) ;
#4840=CARTESIAN_POINT ( 'NONE',  ( 28.05502581071438328, -5.196152422706632912, 165.0604537508149008 ) ) ;
#4845=CARTESIAN_POINT ( 'NONE',  ( 20.99999999999999645, 6.646953231504538984, -2.615624999385474325 ) ) ;
#4849=ORIENTED_EDGE ( 'NONE', *, *, #5730, .F. ) ;
#4853=LINE ( 'NONE', #31384, #28330 ) ;
#4854=CARTESIAN_POINT ( 'NONE',  ( 24.75434669616370087, -3.604726614523244610, 164.5493068216156871 ) ) ;
#4855=AXIS2_PLACEMENT_3D ( 'NONE', #18448, #29798, #30182 ) ;
#4860=CYLINDRICAL_SURFACE ( 'NONE', #5541, 6.000000000000001776 ) ;
#4869=VERTEX_POINT ( 'NONE', #15639 ) ;
#4870=CARTESIAN_POINT ( 'NONE',  ( 15.00000000000000000, 0.000000000000000000, -2.250000000000001776 ) ) ;
#4873=CARTESIAN_POINT ( 'NONE',  ( 37.17435860658612512, 3.604726614523243278, 163.2368371151495694 ) ) ;
#4874=CARTESIAN_POINT ( 'NONE',  ( 24.73633934067528983, 0.000000000000000000, 161.5488335588110544 ) ) ;
#4882=CARTESIAN_POINT ( 'NONE',  ( 23.99999999999999645, 5.196152422706631135, -1.049999999999995381 ) ) ;
#4884=CARTESIAN_POINT ( 'NONE',  ( 21.00000000000000000, -6.646953231504538984, -8.240624999385500971 ) ) ;
#4896=CARTESIAN_POINT ( 'NONE',  ( 24.47817193633207822, 3.604726614523236616, 161.3926148720374556 ) ) ;
#4904=CYLINDRICAL_SURFACE ( 'NONE', #4694, 3.999999999999996447 ) ;
#4906=ORIENTED_EDGE ( 'NONE', *, *, #11723, .T. ) ;
#4907=CARTESIAN_POINT ( 'NONE',  ( 37.33614145406145468, 3.604726614523238837, 165.0860235234823392 ) ) ;
#4908=CARTESIAN_POINT ( 'NONE',  ( 26.75643035624999655, 7.049594010296217766E-16, -6.215624999385465976 ) ) ;
#4911=CARTESIAN_POINT ( 'NONE',  ( 25.32464060422194052, 0.000000000000000000, 168.2731477709303363 ) ) ;
#4921=CARTESIAN_POINT ( 'NONE',  ( 15.24356964374999990, 0.000000000000000000, -4.190624999385467397 ) ) ;
#4924=CARTESIAN_POINT ( 'NONE',  ( 15.24356964375000167, -3.323476615752272600, -0.6656249993855035685 ) ) ;
#4944=ORIENTED_EDGE ( 'NONE', *, *, #22429, .F. ) ;
#4953=FACE_BOUND ( 'NONE', #35834, .T. ) ;
#4963=CARTESIAN_POINT ( 'NONE',  ( 21.00000000000000000, 6.646953231504538984, -6.665624999385467930 ) ) ;
#4966=( BOUNDED_CURVE ( )  B_SPLINE_CURVE ( 2, ( #30976, #5180, #7668, #7853, #10874, #28305, #2528 ),
 .UNSPECIFIED., .F., .F. ) 
 B_SPLINE_CURVE_WITH_KNOTS ( ( 3, 2, 2, 3 ),
 ( 0.8913043478260852526, 0.8985507246376795987, 0.9057971014492740558, 0.9130434782608682909 ),
 .UNSPECIFIED. ) 
 CURVE ( )  GEOMETRIC_REPRESENTATION_ITEM ( )  RATIONAL_B_SPLINE_CURVE ( ( 1.000000000000030864, 0.8660254037844079544, 1.000000000000000000, 0.8660254037844387076, 1.000000000000000000, 0.8660254037844612451, 0.9999999999999774625 ) ) 
 REPRESENTATION_ITEM ( '' )  );
#4971=CARTESIAN_POINT ( 'NONE',  ( 28.32508817407707014, 5.407089921784862696, 169.5446048129269059 ) ) ;
#4986=FACE_OUTER_BOUND ( 'NONE', #33375, .T. ) ;
#4987=ORIENTED_EDGE ( 'NONE', *, *, #28651, .F. ) ;
#4990=EDGE_CURVE ( 'NONE', #13050, #3146, #7113, .T. ) ;
#4992=CARTESIAN_POINT ( 'NONE',  ( 24.85399959338462139, 0.000000000000000000, 162.8936964012349051 ) ) ;
#5002=CARTESIAN_POINT ( 'NONE',  ( 26.99999999999999289, 0.000000000000000000, -8.000000000000000000 ) ) ;
#5005=EDGE_CURVE ( 'NONE', #21861, #11570, #10548, .T. ) ;
#5007=CARTESIAN_POINT ( 'NONE',  ( 24.59583218904140978, 3.604726614523236616, 162.7374777144612779 ) ) ;
#5015=CARTESIAN_POINT ( 'NONE',  ( 26.99999999999999645, 7.347880794884117764E-16, -5.568749998770966769 ) ) ;
#5016=CARTESIAN_POINT ( 'NONE',  ( 18.12178482187500350, -4.985214923628407568, -2.315624999385479388 ) ) ;
#5018=CARTESIAN_POINT ( 'NONE',  ( 24.82458453031440726, 0.000000000000000000, 162.5574806918533000 ) ) ;
#5020=EDGE_CURVE ( 'NONE', #14391, #30675, #18090, .T. ) ;
#5026=CARTESIAN_POINT ( 'NONE',  ( 25.09585677961646866, 3.464101615137752166, 165.6581366896638485 ) ) ;
#5031=CARTESIAN_POINT ( 'NONE',  ( 23.87821517812499650, 4.985214923628404904, -1.303124999385479876 ) ) ;
#5036=CARTESIAN_POINT ( 'NONE',  ( 15.00000000000000000, 0.000000000000000000, -1.743749998770943721 ) ) ;
#5039=CARTESIAN_POINT ( 'NONE',  ( 20.99999999999999645, 0.000000000000000000, 50.00000000000000000 ) ) ;
#5040=CARTESIAN_POINT ( 'NONE',  ( 27.98518077736123288, -5.407089921784865361, 165.6594454903691087 ) ) ;
#5054=EDGE_LOOP ( 'NONE', ( #36895, #16077, #18935, #1891 ) ) ;
#5055=CARTESIAN_POINT ( 'NONE',  ( 15.00000000000000000, 0.000000000000000000, -3.149999999999986144 ) ) ;
#5057=CARTESIAN_POINT ( 'NONE',  ( 26.66784417439646404, 1.063661697287894059, -7.999999999999996447 ) ) ;
#5058=CARTESIAN_POINT ( 'NONE',  ( 30.70615376348499836, -7.209453229046482114, 160.9418451752858346 ) ) ;
#5060=CARTESIAN_POINT ( 'NONE',  ( 25.18413345258806046, 3.604726614523236616, 169.4617919265805881 ) ) ;
#5062=CARTESIAN_POINT ( 'NONE',  ( 29.50988163713361701, 5.988803496771938129, 159.3844543775923341 ) ) ;
#5068=CARTESIAN_POINT ( 'NONE',  ( 18.00000000000000000, 5.196152422706630247, -0.9750000000000036415 ) ) ;
#5070=CARTESIAN_POINT ( 'NONE',  ( 15.24356964375000167, -3.323476615752272600, -10.11562499938547788 ) ) ;
#5074=CARTESIAN_POINT ( 'NONE',  ( 20.99999999999999645, 6.928203230275506996, -6.356249998770953979 ) ) ;
#5079=VECTOR ( 'NONE', #10139, 1000.000000000000000 ) ;
#5081=B_SPLINE_CURVE_WITH_KNOTS ( 'NONE', 3,
 ( #24628, #4342, #7572, #18957 ),
 .UNSPECIFIED., .F., .F.,
 ( 4, 4 ),
 ( 0.000000000000000000, 1.000000000000000000 ),
 .UNSPECIFIED. ) ;
#5086=CARTESIAN_POINT ( 'NONE',  ( 27.55866236128991176, -5.407089921784859143, 160.7843176865825967 ) ) ;
#5096=EDGE_LOOP ( 'NONE', ( #9638, #19365, #12138, #8583, #25132 ) ) ;
#5097=CARTESIAN_POINT ( 'NONE',  ( 37.29038468911893034, -3.604726614523235284, 164.5630213069841830 ) ) ;
#5098=CARTESIAN_POINT ( 'NONE',  ( 23.87821517812500005, -4.985214923628404016, -4.490624999385461891 ) ) ;
#5100=CARTESIAN_POINT ( 'NONE',  ( 31.29445502703164550, -7.209453229046482114, 167.6661593874051164 ) ) ;
#5101=CARTESIAN_POINT ( 'NONE',  ( 25.24293209539601435, 3.464101615137757051, 167.3392152414693328 ) ) ;
#5112=CARTESIAN_POINT ( 'NONE',  ( 15.24356964374999990, 0.000000000000000000, -3.740624999385461003 ) ) ;
#5115=CARTESIAN_POINT ( 'NONE',  ( 26.75643035624999655, 7.049594010296217766E-16, -0.9281249993854934210 ) ) ;
#5127=DIRECTION ( 'NONE',  ( 1.000000000000000000, 0.000000000000000000, 0.000000000000000000 ) ) ;
#5128=PLANE ( 'NONE',  #7526 ) ;
#5130=CYLINDRICAL_SURFACE ( 'NONE', #13327, 6.000000000000001776 ) ;
#5142=CARTESIAN_POINT ( 'NONE',  ( 20.99999999999999645, 0.000000000000000000, -8.000000000000000000 ) ) ;
#5144=CARTESIAN_POINT ( 'NONE',  ( 18.00000000000000355, -5.196152422706632912, -9.825000000000001066 ) ) ;
#5145=ORIENTED_EDGE ( 'NONE', *, *, #32855, .F. ) ;
#5149=CARTESIAN_POINT ( 'NONE',  ( 18.12178482187500350, -4.985214923628407568, -6.478124999385492799 ) ) ;
#5154=EDGE_CURVE ( 'NONE', #27666, #4551, #35006, .T. ) ;
#5155=CARTESIAN_POINT ( 'NONE',  ( 25.10405911393864642, 0.000000000000000000, 168.5465380477087933 ) ) ;
#5158=CARTESIAN_POINT ( 'NONE',  ( 33.65960319901864040, 5.196152422706631135, 160.2787869599868316 ) ) ;
#5160=FACE_OUTER_BOUND ( 'NONE', #36474, .T. ) ;
#5180=CARTESIAN_POINT ( 'NONE',  ( 36.62857725106935192, -3.464101615137295642, 159.7931759234488140 ) ) ;
#5191=CARTESIAN_POINT ( 'NONE',  ( 26.99999999999999289, 0.000000000000000000, -8.000000000000000000 ) ) ;
#5195=CARTESIAN_POINT ( 'NONE',  ( 24.67754069786733240, 0.000000000000000000, 163.6714102439223097 ) ) ;
#5196=CARTESIAN_POINT ( 'NONE',  ( 20.99999999999999645, 0.000000000000000000, -8.000000000000000000 ) ) ;
#5198=EDGE_LOOP ( 'NONE', ( #1983, #252, #12977, #1612 ) ) ;
#5201=CARTESIAN_POINT ( 'NONE',  ( 18.00000000000000355, -5.196152422706632912, -3.918749998770953979 ) ) ;
#5202=CARTESIAN_POINT ( 'NONE',  ( 23.87821517812499650, 4.985214923628404904, -2.990624999385460558 ) ) ;
#5205=DIRECTION ( 'NONE',  ( 0.000000000000000000, 0.000000000000000000, 1.000000000000000000 ) ) ;
#5211=CARTESIAN_POINT ( 'NONE',  ( 28.00273236506578201, 5.196152422706630247, 164.4627369319599097 ) ) ;
#5217=CARTESIAN_POINT ( 'NONE',  ( 20.99999999999999645, 6.646953231504538984, -3.065624999385470062 ) ) ;
#5223=CARTESIAN_POINT ( 'NONE',  ( 27.93736555800505172, -5.196152422706632912, 163.7155909083910501 ) ) ;
#5226=CARTESIAN_POINT ( 'NONE',  ( 15.02283181144952628, 7.347880794884122694E-16, 50.52293445648592751 ) ) ;
#5227=CARTESIAN_POINT ( 'NONE',  ( 33.97620792891898134, -5.407089921784861808, 162.5002714581805492 ) ) ;
#5229=( BOUNDED_CURVE ( )  B_SPLINE_CURVE ( 2, ( #5794, #12230, #35721, #18122, #6933, #35908, #3513 ),
 .UNSPECIFIED., .F., .F. ) 
 B_SPLINE_CURVE_WITH_KNOTS ( ( 3, 2, 2, 3 ),
 ( 0.3043478260869552088, 0.3115942028985494994, 0.3188405797101437900, 0.3260869565217381361 ),
 .UNSPECIFIED. ) 
 CURVE ( )  GEOMETRIC_REPRESENTATION_ITEM ( )  RATIONAL_B_SPLINE_CURVE ( ( 1.000000000000024647, 0.8660254037844140607, 1.000000000000000000, 0.8660254037844387076, 1.000000000000000000, 0.8660254037844571373, 0.9999999999999815703 ) ) 
 REPRESENTATION_ITEM ( '' )  );
#5231=EDGE_CURVE ( 'NONE', #8744, #16385, #16578, .T. ) ;
#5234=CARTESIAN_POINT ( 'NONE',  ( 30.69389748721466304, -6.928203230275506996, 160.8017552964788592 ) ) ;
#5243=CARTESIAN_POINT ( 'NONE',  ( 26.99999999999999645, -3.464101615137751278, -4.762500000000000178 ) ) ;
#5244=CARTESIAN_POINT ( 'NONE',  ( 20.00000000000024869, -5.916079783099657874, -7.999999999999998224 ) ) ;
#5245=CARTESIAN_POINT ( 'NONE',  ( 30.62771359501211066, -7.209453229046482114, 160.0452699470032485 ) ) ;
#5247=CARTESIAN_POINT ( 'NONE',  ( 25.14818170870464797, 0.000000000000000000, 169.0508616136177409 ) ) ;
#5249=CARTESIAN_POINT ( 'NONE',  ( 18.00000000000000000, 5.196152422706630247, -0.9187499987709513150 ) ) ;
#5253=ORIENTED_EDGE ( 'NONE', *, *, #34950, .F. ) ;
#5257=CARTESIAN_POINT ( 'NONE',  ( 18.12178482187500350, -4.985214923628407568, -7.828124999385482674 ) ) ;
#5260=AXIS2_PLACEMENT_3D ( 'NONE', #22579, #31108, #36961 ) ;
#5263=CARTESIAN_POINT ( 'NONE',  ( 37.05343001352376575, 7.646167579472024665E-16, 161.8546169715473013 ) ) ;
#5272=CARTESIAN_POINT ( 'NONE',  ( 30.78949644248743311, -7.209453229046475009, 161.8944563553360467 ) ) ;
#5273=CARTESIAN_POINT ( 'NONE',  ( 25.21678537267883868, 0.000000000000000000, 167.0403568332661450 ) ) ;
#5278=CARTESIAN_POINT ( 'NONE',  ( 21.00000000000000355, 0.000000000000000000, 50.00000000000001421 ) ) ;
#5282=CARTESIAN_POINT ( 'NONE',  ( 33.94189035521207387, -5.407089921784855591, 162.1080197958069107 ) ) ;
#5283=CARTESIAN_POINT ( 'NONE',  ( 26.75643035624999655, -3.323476615752267715, -4.453124999385455141 ) ) ;
#5285=CARTESIAN_POINT ( 'NONE',  ( 25.02888728581879718, -3.604726614523244610, 167.6873201206046247 ) ) ;
#5286=CARTESIAN_POINT ( 'NONE',  ( 31.21356360324042356, 6.928203230275514990, 166.7415661826265421 ) ) ;
#5287=CARTESIAN_POINT ( 'NONE',  ( 20.99999999999999645, 6.928203230275506996, -0.1124999999999909128 ) ) ;
#5292=ORIENTED_EDGE ( 'NONE', *, *, #29381, .T. ) ;
#5295=CARTESIAN_POINT ( 'NONE',  ( 15.00000000000000355, 7.347880794884112834E-16, -8.000000000000000000 ) ) ;
#5299=CARTESIAN_POINT ( 'NONE',  ( 15.00000000000000000, 0.000000000000000000, -3.093749998770961795 ) ) ;
#5300=CARTESIAN_POINT ( 'NONE',  ( 23.87821517812499650, 4.985214923628404904, -2.203124999385491556 ) ) ;
#5304=EDGE_CURVE ( 'NONE', #28188, #17354, #1573, .T. ) ;
#5322=CARTESIAN_POINT ( 'NONE',  ( 24.81477950914817754, 0.000000000000000000, 162.4454087870936121 ) ) ;
#5323=EDGE_LOOP ( 'NONE', ( #14755, #30529, #11955, #14828 ) ) ;
#5324=CARTESIAN_POINT ( 'NONE',  ( 28.32999068460662428, 5.407089921784856479, 169.6006407646945604 ) ) ;
#5332=CARTESIAN_POINT ( 'NONE',  ( 24.00000000000000000, -5.196152422706629359, -9.300000000000002487 ) ) ;
#5333=AXIS2_PLACEMENT_3D ( 'NONE', #14690, #14323, #32305 ) ;
#5338=CARTESIAN_POINT ( 'NONE',  ( 26.75643035624999655, 7.049594010296217766E-16, -5.878124999385475391 ) ) ;
#5340=EDGE_LOOP ( 'NONE', ( #9591, #12794, #30107, #31044 ) ) ;
#5341=AXIS2_PLACEMENT_3D ( 'NONE', #11867, #26088, #19687 ) ;
#5360=ORIENTED_EDGE ( 'NONE', *, *, #26558, .T. ) ;
#5364=CYLINDRICAL_SURFACE ( 'NONE', #36533, 5.999999999999994671 ) ;
#5370=ORIENTED_EDGE ( 'NONE', *, *, #5769, .F. ) ;
#5376=CARTESIAN_POINT ( 'NONE',  ( 27.66324925258708589, 5.407089921784856479, 161.9797513242927209 ) ) ;
#5378=ORIENTED_EDGE ( 'NONE', *, *, #33334, .F. ) ;
#5381=CARTESIAN_POINT ( 'NONE',  ( 26.99999999999999645, 7.347880794884117764E-16, -4.668749998770954868 ) ) ;
#5382=CARTESIAN_POINT ( 'NONE',  ( 18.12178482187500350, -4.985214923628407568, -3.665624999385469707 ) ) ;
#5383=CARTESIAN_POINT ( 'NONE',  ( 15.00000000000000000, 3.464101615137752610, -6.337500000000001243 ) ) ;
#5384=CARTESIAN_POINT ( 'NONE',  ( 15.00000000000000355, 7.347880794884112834E-16, 50.26196565745150480 ) ) ;
#5387=( BOUNDED_CURVE ( )  B_SPLINE_CURVE ( 2, ( #5809, #11504, #14724, #122, #20422, #29493, #6187 ),
 .UNSPECIFIED., .F., .F. ) 
 B_SPLINE_CURVE_WITH_KNOTS ( ( 3, 2, 2, 3 ),
 ( 0.4565217391304337569, 0.4637681159420281030, 0.4710144927536223936, 0.4782608695652167397 ),
 .UNSPECIFIED. ) 
 CURVE ( )  GEOMETRIC_REPRESENTATION_ITEM ( )  RATIONAL_B_SPLINE_CURVE ( ( 1.000000000000018430, 0.8660254037844202779, 1.000000000000000000, 0.8660254037844387076, 1.000000000000000000, 0.8660254037844510311, 0.9999999999999876765 ) ) 
 REPRESENTATION_ITEM ( '' )  );
#5391=CARTESIAN_POINT ( 'NONE',  ( 34.05180404138307182, 5.196152422706631135, 164.7616631013996766 ) ) ;
#5395=CARTESIAN_POINT ( 'NONE',  ( 20.99999999999999645, -6.646953231504538984, -4.640624999385471128 ) ) ;
#5396=CARTESIAN_POINT ( 'NONE',  ( 15.00000000000017408, -3.464101615137856083, -1.762499999999983968 ) ) ;
#5399=ORIENTED_EDGE ( 'NONE', *, *, #16506, .T. ) ;
#5405=CARTESIAN_POINT ( 'NONE',  ( 24.63014976274829593, 3.604726614523240613, 163.1297293768349164 ) ) ;
#5409=CARTESIAN_POINT ( 'NONE',  ( 27.00000000000007816, 3.464101615137709533, -4.237500000000011369 ) ) ;
#5414=DIRECTION ( 'NONE',  ( 0.9961946980917462113, 0.000000000000000000, -0.08715574274765118534 ) ) ;
#5419=CARTESIAN_POINT ( 'NONE',  ( 15.00000000000000178, -3.464101615137757051, -4.012499999999996625 ) ) ;
#5421=CARTESIAN_POINT ( 'NONE',  ( 24.39809759768267128, 0.000000000000000000, 160.4773609931656608 ) ) ;
#5423=CARTESIAN_POINT ( 'NONE',  ( 34.45175145028584041, -5.407089921784855591, 167.9357587796436064 ) ) ;
#5425=CARTESIAN_POINT ( 'NONE',  ( 26.99999999999999645, 7.347880794884117764E-16, -7.874999999999992895 ) ) ;
#5429=ORIENTED_EDGE ( 'NONE', *, *, #4835, .T. ) ;
#5431=LINE ( 'NONE', #31592, #26520 ) ;
#5433=CARTESIAN_POINT ( 'NONE',  ( 21.00000000000000000, 6.646953231504538984, -8.915624999385478588 ) ) ;
#5438=CARTESIAN_POINT ( 'NONE',  ( 33.97620792891898134, -5.407089921784861808, 162.5002714581805492 ) ) ;
#5450=CARTESIAN_POINT ( 'NONE',  ( 24.36051168362275021, 3.604726614523236616, 160.0477520296136049 ) ) ;
#5451=CARTESIAN_POINT ( 'NONE',  ( 24.00000000000000000, -5.196152422706629359, -0.6937499987709483396 ) ) ;
#5460=ORIENTED_EDGE ( 'NONE', *, *, #30351, .F. ) ;
#5461=CARTESIAN_POINT ( 'NONE',  ( 24.51739202056852207, 3.604726614523236616, 161.8409024861787202 ) ) ;
#5462=CARTESIAN_POINT ( 'NONE',  ( 23.87821517812499650, 4.985214923628404904, -8.840624999385482852 ) ) ;
#5464=EDGE_CURVE ( 'NONE', #1229, #34407, #29880, .T. ) ;
#5465=CARTESIAN_POINT ( 'NONE',  ( 34.40762885551985306, -5.407089921784861808, 167.4314352137346873 ) ) ;
#5466=CARTESIAN_POINT ( 'NONE',  ( 28.18902776508177510, 5.196152422706636465, 166.5921030979066586 ) ) ;
#5467=CARTESIAN_POINT ( 'NONE',  ( 20.99999999999999645, 0.000000000000000000, -8.000000000000000000 ) ) ;
#5472=VECTOR ( 'NONE', #9119, 1000.000000000000000 ) ;
#5479=CARTESIAN_POINT ( 'NONE',  ( 26.75643035624999655, -3.323476615752267715, -0.9656249993854794100 ) ) ;
#5488=ADVANCED_FACE ( 'NONE', ( #28855 ), #5364, .T. ) ;
#5490=CARTESIAN_POINT ( 'NONE',  ( 37.10248660225891371, 7.347880794884125653E-16, 165.2099845943227479 ) ) ;
#5496=CARTESIAN_POINT ( 'NONE',  ( 37.33780710767756972, 7.347880794884125653E-16, 167.8997102791704492 ) ) ;
#5501=DIRECTION ( 'NONE',  ( 0.000000000000000000, 0.000000000000000000, 1.000000000000000000 ) ) ;
#5504=EDGE_CURVE ( 'NONE', #19908, #22708, #36220, .T. ) ;
#5505=CARTESIAN_POINT ( 'NONE',  ( 26.99999999999999645, 7.347880794884117764E-16, -5.175000000000013145 ) ) ;
#5509=CARTESIAN_POINT ( 'NONE',  ( 25.33691262237273989, 0.000000000000000000, 169.8107417041232452 ) ) ;
#5511=CARTESIAN_POINT ( 'NONE',  ( 23.99999999999999645, 5.196152422706631135, -9.149999999999991473 ) ) ;
#5516=CARTESIAN_POINT ( 'NONE',  ( 26.75643035624999655, 7.049594010296217766E-16, -9.028124999385489957 ) ) ;
#5522=CARTESIAN_POINT ( 'NONE',  ( 28.16820783713129472, 5.407089921784862696, 167.7514543563617622 ) ) ;
#5528=CARTESIAN_POINT ( 'NONE',  ( 34.32634463103817524, 5.196152422706631135, 167.8996764003886994 ) ) ;
#5531=CARTESIAN_POINT ( 'NONE',  ( 20.99999999999999645, 6.928203230275506996, -0.5062499987709455640 ) ) ;
#5536=EDGE_CURVE ( 'NONE', #10052, #37220, #236, .T. ) ;
#5539=ORIENTED_EDGE ( 'NONE', *, *, #5885, .T. ) ;
#5541=AXIS2_PLACEMENT_3D ( 'NONE', #7346, #31024, #33862 ) ;
#5545=CARTESIAN_POINT ( 'NONE',  ( 26.99999999999999645, 7.347880794884117764E-16, -3.824999999999994849 ) ) ;
#5554=CARTESIAN_POINT ( 'NONE',  ( 25.17429694808911833, 3.464101615137614498, 166.5547119179464346 ) ) ;
#5556=ORIENTED_EDGE ( 'NONE', *, *, #24319, .F. ) ;
#5559=CARTESIAN_POINT ( 'NONE',  ( 30.71105627401454896, -7.209453229046475009, 160.9978811270534891 ) ) ;
#5560=CARTESIAN_POINT ( 'NONE',  ( 26.75643035624999655, 7.049594010296217766E-16, -2.278124999385483740 ) ) ;
#5563=VERTEX_POINT ( 'NONE', #6106 ) ;
#5566=CARTESIAN_POINT ( 'NONE',  ( 15.00000000000000000, 3.464101615137752166, -6.281249998770928045 ) ) ;
#5567=CARTESIAN_POINT ( 'NONE',  ( 15.24356964374999990, 3.323476615752268604, -3.778124999385444660 ) ) ;
#5575=CARTESIAN_POINT ( 'NONE',  ( 27.93736555800505172, -5.196152422706632912, 163.7155909083910501 ) ) ;
#5579=CARTESIAN_POINT ( 'NONE',  ( 26.75643035624999655, 3.323476615752271268, -4.490624999385483207 ) ) ;
#5584=CARTESIAN_POINT ( 'NONE',  ( 36.91292286189034400, -3.464101615137475942, 163.0432611271974679 ) ) ;
#5588=CARTESIAN_POINT ( 'NONE',  ( 37.01094158893428698, -3.604726614523238837, 161.3689720562275340 ) ) ;
#5601=CARTESIAN_POINT ( 'NONE',  ( 26.99999999999999645, 7.347880794884117764E-16, -4.725000000000006750 ) ) ;
#5603=CARTESIAN_POINT ( 'NONE',  ( 31.19395356112219986, -6.928203230275514990, 166.5174223755558955 ) ) ;
#5604=CARTESIAN_POINT ( 'NONE',  ( 24.39482925732963281, 3.604726614523240613, 160.4400036919872150 ) ) ;
#5606=CARTESIAN_POINT ( 'NONE',  ( 24.62194742831900030, -3.464101615137761048, 160.2413280175656212 ) ) ;
#5611=ORIENTED_EDGE ( 'NONE', *, *, #15016, .F. ) ;
#5613=CARTESIAN_POINT ( 'NONE',  ( 20.99999999999999645, 0.000000000000000000, -8.000000000000000000 ) ) ;
#5615=VECTOR ( 'NONE', #34016, 1000.000000000000000 ) ;
#5618=CARTESIAN_POINT ( 'NONE',  ( 23.87821517812499650, 4.985214923628404904, -9.403124999385475746 ) ) ;
#5621=CARTESIAN_POINT ( 'NONE',  ( 21.00000000000000355, 0.000000000000000000, 50.00000000000001421 ) ) ;
#5622=CARTESIAN_POINT ( 'NONE',  ( 33.85854767620964623, -5.407089921784861808, 161.1554086157566985 ) ) ;
#5625=ADVANCED_FACE ( 'NONE', ( #12562 ), #32644, .F. ) ;
#5629=B_SPLINE_CURVE_WITH_KNOTS ( 'NONE', 1,
 ( #32774, #27095 ),
 .UNSPECIFIED., .F., .F.,
 ( 2, 2 ),
 ( 0.000000000000000000, 1.000000000000000000 ),
 .UNSPECIFIED. ) ;
#5632=ORIENTED_EDGE ( 'NONE', *, *, #12144, .T. ) ;
#5636=CARTESIAN_POINT ( 'NONE',  ( 31.39250523762275691, 7.209453229046482114, 168.7868784227583205 ) ) ;
#5637=CARTESIAN_POINT ( 'NONE',  ( 18.00000000000000000, 5.196152422706630247, -3.618749998770959486 ) ) ;
#5646=CARTESIAN_POINT ( 'NONE',  ( 20.99999999999999645, 0.000000000000000000, -8.000000000000000000 ) ) ;
#5648=CARTESIAN_POINT ( 'NONE',  ( 27.67632261399923976, -5.407089921784859143, 162.1291805290064474 ) ) ;
#5649=CARTESIAN_POINT ( 'NONE',  ( 26.75643035624999655, -3.323476615752267715, -7.153124999385460647 ) ) ;
#5651=CARTESIAN_POINT ( 'NONE',  ( 34.49914238540488043, 5.407089921784862696, 168.4774396467310282 ) ) ;
#5652=CARTESIAN_POINT ( 'NONE',  ( 31.09590335053109555, 6.928203230275514990, 165.3967033402026914 ) ) ;
#5660=ORIENTED_EDGE ( 'NONE', *, *, #12641, .T. ) ;
#5666=CARTESIAN_POINT ( 'NONE',  ( 15.24356964375000167, -3.323476615752272600, -2.915624999385482141 ) ) ;
#5678=LINE ( 'NONE', #19749, #16152 ) ;
#5685=CARTESIAN_POINT ( 'NONE',  ( 36.74950584413092258, 7.347880794884125653E-16, 161.1753960670511674 ) ) ;
#5687=CARTESIAN_POINT ( 'NONE',  ( 31.41701779027052766, -7.209453229046475009, 169.0670581815966216 ) ) ;
#5691=CARTESIAN_POINT ( 'NONE',  ( 26.75643035624999655, -3.323476615752267715, -0.8531249993854884694 ) ) ;
#5705=CARTESIAN_POINT ( 'NONE',  ( 21.00000000000000000, -6.646953231504538984, -9.140624999385492444 ) ) ;
#5711=CARTESIAN_POINT ( 'NONE',  ( 24.86873860851999041, 0.000000000000000000, 165.8568123628610920 ) ) ;
#5718=CARTESIAN_POINT ( 'NONE',  ( 28.22540379330944660, -5.407089921784859143, 168.4052071269844930 ) ) ;
#5719=ORIENTED_EDGE ( 'NONE', *, *, #21771, .T. ) ;
#5730=EDGE_CURVE ( 'NONE', #31332, #31979, #16874, .T. ) ;
#5742=CARTESIAN_POINT ( 'NONE',  ( 34.13024420985595953, 5.196152422706631135, 165.6582383296822343 ) ) ;
#5747=CARTESIAN_POINT ( 'NONE',  ( 33.74578993402985816, -5.407089921784855591, 159.8665817251004739 ) ) ;
#5748=VECTOR ( 'NONE', #24135, 1000.000000000000000 ) ;
#5749=CARTESIAN_POINT ( 'NONE',  ( 15.24356964374999990, 0.000000000000000000, -2.503124999385486493 ) ) ;
#5754=EDGE_LOOP ( 'NONE', ( #5802, #16177, #4061 ) ) ;
#5756=CARTESIAN_POINT ( 'NONE',  ( 21.00000000000000000, 6.928203230275506996, -7.256249998770945453 ) ) ;
#5757=CARTESIAN_POINT ( 'NONE',  ( 26.75643035624999655, -3.323476615752267271, -2.653124999385471305 ) ) ;
#5765=CARTESIAN_POINT ( 'NONE',  ( 24.90629303914032988, -3.464101615137757051, 163.4914132213143034 ) ) ;
#5769=EDGE_CURVE ( 'NONE', #27974, #14162, #11976, .T. ) ;
#5770=CARTESIAN_POINT ( 'NONE',  ( 15.24356964374999990, 0.000000000000000000, -5.203124999385494220 ) ) ;
#5771=CARTESIAN_POINT ( 'NONE',  ( 27.00000000000031619, -3.464101615137567869, -1.612499999999994049 ) ) ;
#5781=CARTESIAN_POINT ( 'NONE',  ( 24.51575785039200284, 0.000000000000000000, 161.8222238355895399 ) ) ;
#5784=CARTESIAN_POINT ( 'NONE',  ( 14.99999999999992184, 3.464101615137706425, -4.087499999999989697 ) ) ;
#5789=CARTESIAN_POINT ( 'NONE',  ( 28.08117253353866971, 5.196152422706630247, 165.3593121602424674 ) ) ;
#5793=CARTESIAN_POINT ( 'NONE',  ( 18.00000000000000000, 5.196152422706630247, -5.025000000000002132 ) ) ;
#5794=CARTESIAN_POINT ( 'NONE',  ( 15.00000000000000000, 0.000000000000000000, -3.149999999999986144 ) ) ;
#5795=CARTESIAN_POINT ( 'NONE',  ( 30.58849351077567036, -7.209453229046482114, 159.5969823328619555 ) ) ;
#5797=CARTESIAN_POINT ( 'NONE',  ( 31.35818766391586365, 7.209453229046475009, 168.3946267603846820 ) ) ;
#5802=ORIENTED_EDGE ( 'NONE', *, *, #27416, .F. ) ;
#5803=CARTESIAN_POINT ( 'NONE',  ( 37.18092677073180141, 7.347880794884125653E-16, 166.1065598226053055 ) ) ;
#5805=FACE_OUTER_BOUND ( 'NONE', #34773, .T. ) ;
#5806=CARTESIAN_POINT ( 'NONE',  ( 15.24356964374999990, 0.000000000000000000, -6.890624999385474680 ) ) ;
#5809=CARTESIAN_POINT ( 'NONE',  ( 37.02404643378602600, 7.347880794884125653E-16, 164.3134093660401618 ) ) ;
#5814=CARTESIAN_POINT ( 'NONE',  ( 25.37693404997765256, -3.464101615137757051, 168.8708645910097346 ) ) ;
#5822=AXIS2_PLACEMENT_3D ( 'NONE', #13334, #18853, #7838 ) ;
#5823=ORIENTED_EDGE ( 'NONE', *, *, #13538, .T. ) ;
#5826=EDGE_CURVE ( 'NONE', #27950, #35077, #28466, .T. ) ;
#5828=CARTESIAN_POINT ( 'NONE',  ( 24.43895185209563792, 3.604726614523236616, 160.9443272578961626 ) ) ;
#5829=CARTESIAN_POINT ( 'NONE',  ( 26.99999999999999645, 3.464101615137755275, -3.281249998770945808 ) ) ;
#5831=CARTESIAN_POINT ( 'NONE',  ( 24.61867908796596183, 0.000000000000000000, 160.2039707163872038 ) ) ;
#5835=CYLINDRICAL_SURFACE ( 'NONE', #2084, 5.999999999999994671 ) ;
#5840=CARTESIAN_POINT ( 'NONE',  ( 27.71554269823568362, -5.407089921784859143, 162.5774681431477404 ) ) ;
#5841=CARTESIAN_POINT ( 'NONE',  ( 23.87821517812500005, -4.985214923628404016, -8.090624999385454430 ) ) ;
#5843=CARTESIAN_POINT ( 'NONE',  ( 28.28586808984062628, 5.407089921784862696, 169.0963171987856128 ) ) ;
#5844=CARTESIAN_POINT ( 'NONE',  ( 37.05999817766942783, -3.464101615137755275, 164.7243396790030090 ) ) ;
#5845=DIRECTION ( 'NONE',  ( 0.08715574274765150453, 0.000000000000000000, 0.9961946980917461003 ) ) ;
#5856=CARTESIAN_POINT ( 'NONE',  ( 21.00000000000000000, -6.646953231504538984, -3.740624999385479654 ) ) ;
#5870=AXIS2_PLACEMENT_3D ( 'NONE', #12967, #15624, #3866 ) ;
#5872=CARTESIAN_POINT ( 'NONE',  ( 27.95370725966311554, 5.196152422706636465, 163.9023774130589288 ) ) ;
#5878=DIRECTION ( 'NONE',  ( 1.000000000000000000, 0.000000000000000000, 0.000000000000000000 ) ) ;
#5880=CARTESIAN_POINT ( 'NONE',  ( 23.87821517812499650, 4.985214923628404904, -1.190624999385464511 ) ) ;
#5881=DIRECTION ( 'NONE',  ( 0.000000000000000000, 0.000000000000000000, 1.000000000000000000 ) ) ;
#5885=EDGE_CURVE ( 'NONE', #4551, #972, #7440, .T. ) ;
#5886=CYLINDRICAL_SURFACE ( 'NONE', #9092, 6.000000000000001776 ) ;
#5890=ORIENTED_EDGE ( 'NONE', *, *, #6458, .F. ) ;
#5891=( BOUNDED_CURVE ( )  B_SPLINE_CURVE ( 2, ( #23506, #25781, #2841, #20297, #29173, #36636, #34499 ),
 .UNSPECIFIED., .F., .F. ) 
 B_SPLINE_CURVE_WITH_KNOTS ( ( 3, 2, 2, 3 ),
 ( 0.02173913043478289606, 0.02898550724637719705, 0.03623188405797149458, 0.04347826086956579211 ),
 .UNSPECIFIED. ) 
 CURVE ( )  GEOMETRIC_REPRESENTATION_ITEM ( )  RATIONAL_B_SPLINE_CURVE ( ( 0.9999999999999946709, 0.8660254037844440367, 1.000000000000000000, 0.8660254037844387076, 1.000000000000000000, 0.8660254037844280495, 1.000000000000010658 ) ) 
 REPRESENTATION_ITEM ( '' )  );
#5895=CARTESIAN_POINT ( 'NONE',  ( 18.12178482187499640, 4.985214923628404904, -9.778124999385489957 ) ) ;
#5900=CARTESIAN_POINT ( 'NONE',  ( 28.08976766865841057, 5.407089921784862696, 166.8548791280792045 ) ) ;
#5903=ADVANCED_FACE ( 'NONE', ( #24316 ), #36604, .T. ) ;
#5907=CARTESIAN_POINT ( 'NONE',  ( 25.14818170870464797, 0.000000000000000000, 169.0508616136177409 ) ) ;
#5916=VERTEX_POINT ( 'NONE', #4587 ) ;
#5921=CARTESIAN_POINT ( 'NONE',  ( 26.99999999999999645, 7.347880794884117764E-16, -4.218749998770948473 ) ) ;
#5932=VERTEX_POINT ( 'NONE', #27712 ) ;
#5935=CARTESIAN_POINT ( 'NONE',  ( 30.63261610554165770, -7.209453229046475009, 160.1013058987709030 ) ) ;
#5936=( BOUNDED_SURFACE ( )  B_SPLINE_SURFACE ( 1, 2, ( 
 ( #37338, #26344, #22775, #35062, #6263, #28996, #11388, #8548, #17088, #26532, #34508, #34323, #19940, #8735, #8369, #11572, #14240, #29184, #20306, #5691, #20114, #14799, #3226, #34878, #28811, #31479, #3038, #31847, #5880, #2848, #380, #11947, #14609, #26160, #23516, #193, #9112, #20677, #32224, #17841, #29376, #3414, #32411, #29755, #21250, #18400, #35814, #15362, #3786, #9300, #15930, #23896, #12517, #27479, #32789, #20872, #12323, #15550, #6452, #24081, #35626, #18214, #18024, #36003, #26915, #35438, #9856, #6824, #943, #21061, #21435, #9672, #6639, #29949, #27290, #32599, #33169, #3977, #27108, #1132, #29569, #12698, #24270, #32975, #7029, #3606, #12129, #7214, #18595, #15173, #30139, #4169, #15739, #753, #1320, #12888, #24453, #26720, #9485, #10040, #21617, #18786, #30327, #4351, #23705, #35247, #28037, #16677, #31257, #28224, #30520, #2252, #22362, #4540, #4725, #5283, #5098, #16863, #1505, #2069, #1693, #24819, #27848, #16116, #13832, #13081, #25378, #22546, #33725, #27668, #36372, #21805, #24635, #13267, #36186, #10230, #1881, #33358, #13452, #7393, #36748, #16301, #10418, #18966, #31075, #25196, #13643, #21993, #33540, #7767, #25002, #36558, #7580, #33911, #7953, #30885, #10599, #10789, #19156, #30704, #22179, #19346, #4908, #16489, #19528, #36927, #10975, #34095, #8145, #19717, #31621, #20076, #25563, #32184, #2621, #28770, #6218, #37481, #37115, #28583, #31804, #22736, #2810, #14380, #34467, #11163, #14757, #5649, #14197, #14567, #23103, #17232, #37301, #151, #25938, #22922, #11532, #6024, #11350, #11903, #34646, #8691, #20265, #34285, #2997, #26300, #25748, #23290, #20638, #8510, #8328, #338, #5841, #17419, #26119, #28959, #11715, #34835, #8875, #20453, #31995, #17610, #29141, #3181, #23470, #35023, #9067, #28400, #19899, #2438, #14012, #31440, #5462, #17045, #18169, #29710, #12279, #3935, #35205, #33128, #12846, #12471, #23661, #24225, #24039, #18357, #6407, #21018, #15510, #1090, #20827, #9254, #12660, #3744, #9440, #35771, #32552, #32368, #520, #6783, #32934, #10000, #6987, #17980, #18556, #9815, #29524, #6595, #21581 ),
 ( #21392, #17791, #30096, #1275, #35584, #3564, #15126, #12087, #29334, #26677, #3371, #14941, #15317, #26488, #26870, #708, #27065, #900, #23853, #35391, #4129, #15701, #29906, #9629, #21206, #32746, #27252, #24413, #35962, #27995, #13603, #36518, #21952, #33685, #22508, #7171, #30665, #19115, #18744, #33497, #36331, #27434, #24780, #16264, #13412, #30846, #10377, #7543, #4311, #10933, #18928, #4682, #30285, #27814, #15890, #7356, #10562, #1467, #1842, #24960, #4870, #2025, #10190, #24596, #25153, #22139, #7725, #36708, #19308, #13041, #36147, #16450, #22320, #36887, #33872, #21766, #7913, #10747, #33316, #19487, #30480, #31034, #4501, #16078, #5055, #27627, #1657, #16638, #13231, #28179, #2210, #13791, #25339, #28727, #11120, #19857, #16820, #289, #8284, #8101, #31214, #34426, #11855, #22875, #28362, #31763, #37259, #5419, #2398, #26076, #20215, #23058, #34241, #26254, #2765, #8463, #31578, #13972, #17373, #2950, #25891, #11307, #34604, #34055, #19675, #20033, #5601, #5243, #17187, #25707, #25521, #14153, #14337, #37440, #5793, #11489, #8646, #37074, #22697, #31400, #28914, #17000, #14520, #28540, #2583, #104, #11668, #23243, #34790, #8834, #20406, #31947, #5979, #17560, #29094, #3137, #14705, #32319, #32693, #9395, #17931, #23801, #1038, #6360, #6931, #35339, #20969, #32502, #29284, #35536, #21344, #9206, #18309, #15647, #6548, #18121, #29475, #9581, #3323, #1747, #18502, #29664, #14894, #29849, #3699, #23992, #12042, #26629, #12421, #21155, #32883, #3885, #6736, #15459, #27011, #15267, #26820, #850, #27717, #12609, #24175, #35720, #9767, #30041, #4075, #3511, #23424, #34975, #9018, #20589, #32131, #6169, #17743, #20775, #658, #12229, #26442, #15079, #474, #23610, #35155, #2305, #37169, #25429, #2117, #36795, #8002, #28085, #22228, #17095, #36982, #22782, #25056, #16725, #13694, #10650, #34331, #11025, #34145, #19575, #33960, #13881, #19207, #19767, #5511, #31487, #31305, #28634, #5332, #24872, #33593, #11209, #31127, #25244, #16350, #13314, #10838, #16910, #33779, #14063, #19947, #7818, #5144, #28271, #22412, #22599, #30754, #19395, #8192 ) ),
 .UNSPECIFIED., .F., .F., .F. ) 
 B_SPLINE_SURFACE_WITH_KNOTS ( ( 2, 2 ),
 ( 3, 2, 2, 2, 2, 2, 2, 2, 2, 2, 2, 2, 2, 2, 2, 2, 2, 2, 2, 2, 2, 2, 2, 2, 2, 2, 2, 2, 2, 2, 2, 2, 2, 2, 2, 2, 2, 2, 2, 2, 2, 2, 2, 2, 2, 2, 2, 2, 2, 2, 2, 2, 2, 2, 2, 2, 2, 2, 2, 2, 2, 2, 2, 2, 2, 2, 2, 2, 2, 2, 2, 2, 2, 2, 2, 2, 2, 2, 2, 2, 2, 2, 2, 2, 2, 2, 2, 2, 2, 2, 2, 2, 2, 2, 2, 2, 2, 2, 2, 2, 2, 2, 2, 2, 2, 2, 2, 2, 2, 2, 2, 2, 2, 2, 2, 2, 2, 2, 2, 2, 2, 2, 2, 2, 2, 2, 2, 2, 2, 2, 2, 2, 2, 2, 3 ),
 ( 0.000000000000000000, 1.000000000000000000 ),
 ( 0.000000000000000000, 0.007246376811594202987, 0.01449275362318840597, 0.02173913043478260809, 0.02898550724637681195, 0.03623188405797101580, 0.04347826086956521618, 0.05072463768115942351, 0.05797101449275362389, 0.06521739130434782428, 0.07246376811594203160, 0.07971014492753622505, 0.08695652173913043237, 0.09420289855072463969, 0.1014492753623188470, 0.1086956521739130405, 0.1159420289855072478, 0.1231884057971014551, 0.1304347826086956486, 0.1376811594202898559, 0.1449275362318840632, 0.1521739130434782705, 0.1594202898550724501, 0.1666666666666666574, 0.1739130434782608647, 0.1811594202898550721, 0.1884057971014492794, 0.1956521739130434867, 0.2028985507246376940, 0.2101449275362318736, 0.2173913043478260809, 0.2246376811594202882, 0.2318840579710144956, 0.2391304347826087029, 0.2463768115942029102, 0.2536231884057971175, 0.2608695652173912971, 0.2681159420289855322, 0.2753623188405797118, 0.2826086956521738913, 0.2898550724637681264, 0.2971014492753623060, 0.3043478260869565410, 0.3115942028985507206, 0.3188405797101449002, 0.3260869565217391353, 0.3333333333333333148, 0.3405797101449275499, 0.3478260869565217295, 0.3550724637681159646, 0.3623188405797101441, 0.3695652173913043237, 0.3768115942028985588, 0.3840579710144927383, 0.3913043478260869734, 0.3985507246376811530, 0.4057971014492753881, 0.4130434782608695676, 0.4202898550724637472, 0.4275362318840579823, 0.4347826086956521618, 0.4420289855072463969, 0.4492753623188405765, 0.4565217391304347561, 0.4637681159420289911, 0.4710144927536231707, 0.4782608695652174058, 0.4855072463768115854, 0.4927536231884058204, 0.5000000000000000000, 0.5072463768115942351, 0.5144927536231883591, 0.5217391304347825942, 0.5289855072463768293, 0.5362318840579710644, 0.5434782608695651884, 0.5507246376811594235, 0.5579710144927536586, 0.5652173913043477826, 0.5724637681159420177, 0.5797101449275362528, 0.5869565217391304879, 0.5942028985507246119, 0.6014492753623188470, 0.6086956521739130821, 0.6159420289855072062, 0.6231884057971014412, 0.6304347826086956763, 0.6376811594202898004, 0.6449275362318840354, 0.6521739130434782705, 0.6594202898550725056, 0.6666666666666666297, 0.6739130434782608647, 0.6811594202898550998, 0.6884057971014492239, 0.6956521739130434590, 0.7028985507246376940, 0.7101449275362319291, 0.7173913043478260532, 0.7246376811594202882, 0.7318840579710145233, 0.7391304347826086474, 0.7463768115942028825, 0.7536231884057971175, 0.7608695652173913526, 0.7681159420289854767, 0.7753623188405797118, 0.7826086956521739468, 0.7898550724637680709, 0.7971014492753623060, 0.8043478260869565410, 0.8115942028985507761, 0.8188405797101449002, 0.8260869565217391353, 0.8333333333333333703, 0.8405797101449274944, 0.8478260869565217295, 0.8550724637681159646, 0.8623188405797101996, 0.8695652173913043237, 0.8768115942028985588, 0.8840579710144927938, 0.8913043478260869179, 0.8985507246376811530, 0.9057971014492753881, 0.9130434782608695121, 0.9202898550724637472, 0.9275362318840579823, 0.9347826086956522174, 0.9420289855072463414, 0.9492753623188405765, 0.9565217391304348116, 0.9637681159420289356, 0.9662082973083874204 ),
 .UNSPECIFIED. ) 
 GEOMETRIC_REPRESENTATION_ITEM ( )  RATIONAL_B_SPLINE_SURFACE ( (
 ( 1.000000000000000000, 0.8660254037844387076, 1.000000000000000000, 0.8660254037844387076, 1.000000000000000000, 0.8660254037844387076, 1.000000000000000000, 0.8660254037844387076, 1.000000000000000000, 0.8660254037844387076, 1.000000000000000000, 0.8660254037844387076, 1.000000000000000000, 0.8660254037844387076, 1.000000000000000000, 0.8660254037844387076, 1.000000000000000000, 0.8660254037844387076, 1.000000000000000000, 0.8660254037844387076, 1.000000000000000000, 0.8660254037844387076, 1.000000000000000000, 0.8660254037844387076, 1.000000000000000000, 0.8660254037844387076, 1.000000000000000000, 0.8660254037844387076, 1.000000000000000000, 0.8660254037844387076, 1.000000000000000000, 0.8660254037844387076, 1.000000000000000000, 0.8660254037844387076, 1.000000000000000000, 0.8660254037844387076, 1.000000000000000000, 0.8660254037844387076, 1.000000000000000000, 0.8660254037844387076, 1.000000000000000000, 0.8660254037844387076, 1.000000000000000000, 0.8660254037844387076, 1.000000000000000000, 0.8660254037844387076, 1.000000000000000000, 0.8660254037844387076, 1.000000000000000000, 0.8660254037844387076, 1.000000000000000000, 0.8660254037844387076, 1.000000000000000000, 0.8660254037844387076, 1.000000000000000000, 0.8660254037844387076, 1.000000000000000000, 0.8660254037844387076, 1.000000000000000000, 0.8660254037844387076, 1.000000000000000000, 0.8660254037844387076, 1.000000000000000000, 0.8660254037844387076, 1.000000000000000000, 0.8660254037844387076, 1.000000000000000000, 0.8660254037844387076, 1.000000000000000000, 0.8660254037844387076, 1.000000000000000000, 0.8660254037844387076, 1.000000000000000000, 0.8660254037844387076, 1.000000000000000000, 0.8660254037844387076, 1.000000000000000000, 0.8660254037844387076, 1.000000000000000000, 0.8660254037844387076, 1.000000000000000000, 0.8660254037844387076, 1.000000000000000000, 0.8660254037844387076, 1.000000000000000000, 0.8660254037844387076, 1.000000000000000000, 0.8660254037844387076, 1.000000000000000000, 0.8660254037844387076, 1.000000000000000000, 0.8660254037844387076, 1.000000000000000000, 0.8660254037844387076, 1.000000000000000000, 0.8660254037844387076, 1.000000000000000000, 0.8660254037844387076, 1.000000000000000000, 0.8660254037844387076, 1.000000000000000000, 0.8660254037844387076, 1.000000000000000000, 0.8660254037844387076, 1.000000000000000000, 0.8660254037844387076, 1.000000000000000000, 0.8660254037844387076, 1.000000000000000000, 0.8660254037844387076, 1.000000000000000000, 0.8660254037844387076, 1.000000000000000000, 0.8660254037844387076, 1.000000000000000000, 0.8660254037844387076, 1.000000000000000000, 0.8660254037844387076, 1.000000000000000000, 0.8660254037844387076, 1.000000000000000000, 0.8660254037844387076, 1.000000000000000000, 0.8660254037844387076, 1.000000000000000000, 0.8660254037844387076, 1.000000000000000000, 0.8660254037844387076, 1.000000000000000000, 0.8660254037844387076, 1.000000000000000000, 0.8660254037844387076, 1.000000000000000000, 0.8660254037844387076, 1.000000000000000000, 0.8660254037844387076, 1.000000000000000000, 0.8660254037844387076, 1.000000000000000000, 0.8660254037844387076, 1.000000000000000000, 0.8660254037844387076, 1.000000000000000000, 0.8660254037844387076, 1.000000000000000000, 0.8660254037844387076, 1.000000000000000000, 0.8660254037844387076, 1.000000000000000000, 0.8660254037844387076, 1.000000000000000000, 0.8660254037844387076, 1.000000000000000000, 0.8660254037844387076, 1.000000000000000000, 0.8660254037844387076, 1.000000000000000000, 0.8660254037844387076, 1.000000000000000000, 0.8660254037844387076, 1.000000000000000000, 0.8660254037844387076, 1.000000000000000000, 0.8660254037844387076, 1.000000000000000000, 0.8660254037844387076, 1.000000000000000000, 0.8660254037844387076, 1.000000000000000000, 0.8660254037844387076, 1.000000000000000000, 0.8660254037844387076, 1.000000000000000000, 0.8660254037844387076, 1.000000000000000000, 0.8660254037844387076, 1.000000000000000000, 0.8660254037844387076, 1.000000000000000000, 0.8660254037844387076, 1.000000000000000000, 0.8660254037844387076, 1.000000000000000000, 0.8660254037844387076, 1.000000000000000000, 0.8660254037844387076, 1.000000000000000000, 0.8660254037844387076, 1.000000000000000000, 0.8660254037844387076, 1.000000000000000000, 0.8660254037844387076, 1.000000000000000000, 0.8660254037844387076, 1.000000000000000000, 0.8660254037844387076, 1.000000000000000000, 0.8660254037844387076, 1.000000000000000000, 0.8660254037844387076, 1.000000000000000000, 0.8660254037844387076, 1.000000000000000000, 0.8660254037844387076, 1.000000000000000000, 0.8660254037844387076, 1.000000000000000000, 0.8660254037844387076, 1.000000000000000000, 0.8660254037844387076, 1.000000000000000000, 0.8660254037844387076, 1.000000000000000000, 0.8660254037844387076, 1.000000000000000000, 0.8660254037844387076, 1.000000000000000000, 0.8660254037844387076, 1.000000000000000000, 0.8660254037844387076, 1.000000000000000000, 0.8660254037844387076, 1.000000000000000000, 0.8660254037844387076, 1.000000000000000000, 0.8660254037844387076, 1.000000000000000000, 0.8660254037844387076, 1.000000000000000000, 0.8660254037844387076, 1.000000000000000000, 0.8660254037844387076, 1.000000000000000000, 0.8660254037844387076, 1.000000000000000000, 0.8660254037844387076, 1.000000000000000000, 0.8660254037844387076, 1.000000000000000000, 0.8660254037844387076, 1.000000000000000000, 0.8660254037844387076, 1.000000000000000000, 0.8660254037844387076, 1.000000000000000000, 0.8660254037844387076, 1.000000000000000000, 0.8660254037844387076, 1.000000000000000000, 0.8660254037844387076, 1.000000000000000000, 0.8660254037844387076, 1.000000000000000000, 0.8660254037844387076, 1.000000000000000000, 0.8660254037844387076, 1.000000000000000000, 0.8660254037844387076, 1.000000000000000000, 0.8660254037844387076, 1.000000000000000000, 0.8660254037844387076, 1.000000000000000000, 0.8660254037844387076, 1.000000000000000000, 0.8660254037844387076, 1.000000000000000000, 0.9548847207714155072, 0.9401541335272467492),
 ( 1.000000000000000000, 0.8660254037844387076, 1.000000000000000000, 0.8660254037844387076, 1.000000000000000000, 0.8660254037844387076, 1.000000000000000000, 0.8660254037844387076, 1.000000000000000000, 0.8660254037844387076, 1.000000000000000000, 0.8660254037844387076, 1.000000000000000000, 0.8660254037844387076, 1.000000000000000000, 0.8660254037844387076, 1.000000000000000000, 0.8660254037844387076, 1.000000000000000000, 0.8660254037844387076, 1.000000000000000000, 0.8660254037844387076, 1.000000000000000000, 0.8660254037844387076, 1.000000000000000000, 0.8660254037844387076, 1.000000000000000000, 0.8660254037844387076, 1.000000000000000000, 0.8660254037844387076, 1.000000000000000000, 0.8660254037844387076, 1.000000000000000000, 0.8660254037844387076, 1.000000000000000000, 0.8660254037844387076, 1.000000000000000000, 0.8660254037844387076, 1.000000000000000000, 0.8660254037844387076, 1.000000000000000000, 0.8660254037844387076, 1.000000000000000000, 0.8660254037844387076, 1.000000000000000000, 0.8660254037844387076, 1.000000000000000000, 0.8660254037844387076, 1.000000000000000000, 0.8660254037844387076, 1.000000000000000000, 0.8660254037844387076, 1.000000000000000000, 0.8660254037844387076, 1.000000000000000000, 0.8660254037844387076, 1.000000000000000000, 0.8660254037844387076, 1.000000000000000000, 0.8660254037844387076, 1.000000000000000000, 0.8660254037844387076, 1.000000000000000000, 0.8660254037844387076, 1.000000000000000000, 0.8660254037844387076, 1.000000000000000000, 0.8660254037844387076, 1.000000000000000000, 0.8660254037844387076, 1.000000000000000000, 0.8660254037844387076, 1.000000000000000000, 0.8660254037844387076, 1.000000000000000000, 0.8660254037844387076, 1.000000000000000000, 0.8660254037844387076, 1.000000000000000000, 0.8660254037844387076, 1.000000000000000000, 0.8660254037844387076, 1.000000000000000000, 0.8660254037844387076, 1.000000000000000000, 0.8660254037844387076, 1.000000000000000000, 0.8660254037844387076, 1.000000000000000000, 0.8660254037844387076, 1.000000000000000000, 0.8660254037844387076, 1.000000000000000000, 0.8660254037844387076, 1.000000000000000000, 0.8660254037844387076, 1.000000000000000000, 0.8660254037844387076, 1.000000000000000000, 0.8660254037844387076, 1.000000000000000000, 0.8660254037844387076, 1.000000000000000000, 0.8660254037844387076, 1.000000000000000000, 0.8660254037844387076, 1.000000000000000000, 0.8660254037844387076, 1.000000000000000000, 0.8660254037844387076, 1.000000000000000000, 0.8660254037844387076, 1.000000000000000000, 0.8660254037844387076, 1.000000000000000000, 0.8660254037844387076, 1.000000000000000000, 0.8660254037844387076, 1.000000000000000000, 0.8660254037844387076, 1.000000000000000000, 0.8660254037844387076, 1.000000000000000000, 0.8660254037844387076, 1.000000000000000000, 0.8660254037844387076, 1.000000000000000000, 0.8660254037844387076, 1.000000000000000000, 0.8660254037844387076, 1.000000000000000000, 0.8660254037844387076, 1.000000000000000000, 0.8660254037844387076, 1.000000000000000000, 0.8660254037844387076, 1.000000000000000000, 0.8660254037844387076, 1.000000000000000000, 0.8660254037844387076, 1.000000000000000000, 0.8660254037844387076, 1.000000000000000000, 0.8660254037844387076, 1.000000000000000000, 0.8660254037844387076, 1.000000000000000000, 0.8660254037844387076, 1.000000000000000000, 0.8660254037844387076, 1.000000000000000000, 0.8660254037844387076, 1.000000000000000000, 0.8660254037844387076, 1.000000000000000000, 0.8660254037844387076, 1.000000000000000000, 0.8660254037844387076, 1.000000000000000000, 0.8660254037844387076, 1.000000000000000000, 0.8660254037844387076, 1.000000000000000000, 0.8660254037844387076, 1.000000000000000000, 0.8660254037844387076, 1.000000000000000000, 0.8660254037844387076, 1.000000000000000000, 0.8660254037844387076, 1.000000000000000000, 0.8660254037844387076, 1.000000000000000000, 0.8660254037844387076, 1.000000000000000000, 0.8660254037844387076, 1.000000000000000000, 0.8660254037844387076, 1.000000000000000000, 0.8660254037844387076, 1.000000000000000000, 0.8660254037844387076, 1.000000000000000000, 0.8660254037844387076, 1.000000000000000000, 0.8660254037844387076, 1.000000000000000000, 0.8660254037844387076, 1.000000000000000000, 0.8660254037844387076, 1.000000000000000000, 0.8660254037844387076, 1.000000000000000000, 0.8660254037844387076, 1.000000000000000000, 0.8660254037844387076, 1.000000000000000000, 0.8660254037844387076, 1.000000000000000000, 0.8660254037844387076, 1.000000000000000000, 0.8660254037844387076, 1.000000000000000000, 0.8660254037844387076, 1.000000000000000000, 0.8660254037844387076, 1.000000000000000000, 0.8660254037844387076, 1.000000000000000000, 0.8660254037844387076, 1.000000000000000000, 0.8660254037844387076, 1.000000000000000000, 0.8660254037844387076, 1.000000000000000000, 0.8660254037844387076, 1.000000000000000000, 0.8660254037844387076, 1.000000000000000000, 0.8660254037844387076, 1.000000000000000000, 0.8660254037844387076, 1.000000000000000000, 0.8660254037844387076, 1.000000000000000000, 0.8660254037844387076, 1.000000000000000000, 0.8660254037844387076, 1.000000000000000000, 0.8660254037844387076, 1.000000000000000000, 0.8660254037844387076, 1.000000000000000000, 0.8660254037844387076, 1.000000000000000000, 0.8660254037844387076, 1.000000000000000000, 0.8660254037844387076, 1.000000000000000000, 0.8660254037844387076, 1.000000000000000000, 0.8660254037844387076, 1.000000000000000000, 0.8660254037844387076, 1.000000000000000000, 0.8660254037844387076, 1.000000000000000000, 0.8660254037844387076, 1.000000000000000000, 0.8660254037844387076, 1.000000000000000000, 0.8660254037844387076, 1.000000000000000000, 0.8660254037844387076, 1.000000000000000000, 0.8660254037844387076, 1.000000000000000000, 0.8660254037844387076, 1.000000000000000000, 0.8660254037844387076, 1.000000000000000000, 0.8660254037844387076, 1.000000000000000000, 0.8660254037844387076, 1.000000000000000000, 0.8660254037844387076, 1.000000000000000000, 0.9548847207714155072, 0.9401541335272467492) ) ) 
 REPRESENTATION_ITEM ( '' )  SURFACE ( )  );
#5937=CARTESIAN_POINT ( 'NONE',  ( 18.12178482187499640, 4.985214923628404904, -2.128124999385472282 ) ) ;
#5942=ORIENTED_EDGE ( 'NONE', *, *, #16906, .T. ) ;
#5943=CARTESIAN_POINT ( 'NONE',  ( 26.75643035624999655, -3.323476615752267271, -5.353124999385477700 ) ) ;
#5944=CARTESIAN_POINT ( 'NONE',  ( 33.61057809361597748, 5.196152422706637353, 159.7184274410858507 ) ) ;
#5949=VECTOR ( 'NONE', #32868, 1000.000000000000000 ) ;
#5952=CARTESIAN_POINT ( 'NONE',  ( 24.74287602148848464, 3.464101615137752166, 161.6235481623922681 ) ) ;
#5956=( BOUNDED_CURVE ( )  B_SPLINE_CURVE ( 2, ( #37036, #22659, #34204, #12145, #28507, #14117, #26736 ),
 .UNSPECIFIED., .F., .F. ) 
 B_SPLINE_CURVE_WITH_KNOTS ( ( 3, 2, 2, 3 ),
 ( 0.1956521739130427651, 0.2028985507246371112, 0.2101449275362314573, 0.2173913043478258034 ),
 .UNSPECIFIED. ) 
 CURVE ( )  GEOMETRIC_REPRESENTATION_ITEM ( )  RATIONAL_B_SPLINE_CURVE ( ( 1.000000000000013323, 0.8660254037844252739, 1.000000000000000000, 0.8660254037844387076, 1.000000000000000000, 0.8660254037844438146, 0.9999999999999948930 ) ) 
 REPRESENTATION_ITEM ( '' )  );
#5957=CARTESIAN_POINT ( 'NONE',  ( 15.24356964374999990, 0.000000000000000000, -4.303124999385482319 ) ) ;
#5965=CARTESIAN_POINT ( 'NONE',  ( 25.01527935017339743, -2.343145750507547032, 50.00000000000000000 ) ) ;
#5966=CARTESIAN_POINT ( 'NONE',  ( 24.66936984698473623, 3.604726614523240613, 163.5780169909762094 ) ) ;
#5979=CARTESIAN_POINT ( 'NONE',  ( 24.00000000000000000, -5.196152422706629359, -5.700000000000010836 ) ) ;
#5981=ADVANCED_FACE ( 'NONE', ( #27528 ), #21849, .T. ) ;
#5982=CARTESIAN_POINT ( 'NONE',  ( 30.90960795051509891, 6.928203230275506996, 163.2673371742559141 ) ) ;
#5984=CARTESIAN_POINT ( 'NONE',  ( 37.41131328218130392, 7.646167579472015790E-16, 165.9452414505865079 ) ) ;
#5994=CARTESIAN_POINT ( 'NONE',  ( 26.75643035624999655, -3.323476615752267715, -7.153124999385460647 ) ) ;
#5996=CARTESIAN_POINT ( 'NONE',  ( 18.12178482187499640, 4.985214923628404904, -10.22812499938549635 ) ) ;
#6001=CARTESIAN_POINT ( 'NONE',  ( 27.55375985076035761, -5.407089921784865361, 160.7282817348149706 ) ) ;
#6011=CARTESIAN_POINT ( 'NONE',  ( 25.23192384099550267, 3.919932473903637860, -7.999999999999996447 ) ) ;
#6012=CARTESIAN_POINT ( 'NONE',  ( 24.36704836432882004, -3.604726614523240613, 160.1224666319704681 ) ) ;
#6013=CARTESIAN_POINT ( 'NONE',  ( 26.99999999999999645, -3.464101615137751278, -2.006249998770952558 ) ) ;
#6020=CARTESIAN_POINT ( 'NONE',  ( 36.63184559142159458, 7.347880794884125653E-16, 159.8305332246273167 ) ) ;
#6022=VERTEX_POINT ( 'NONE', #22222 ) ;
#6023=CARTESIAN_POINT ( 'NONE',  ( 24.63832061363088854, 0.000000000000000000, 163.2231226297810451 ) ) ;
#6024=CARTESIAN_POINT ( 'NONE',  ( 26.75643035624999655, 3.323476615752271712, -7.528124999385462424 ) ) ;
#6026=CARTESIAN_POINT ( 'NONE',  ( 24.87200694887302888, -3.604726614523244610, 165.8941696640395378 ) ) ;
#6027=CARTESIAN_POINT ( 'NONE',  ( 31.05668326629465170, 6.928203230275514990, 164.9484157260613699 ) ) ;
#6028=DIRECTION ( 'NONE',  ( 1.000000000000000000, 0.000000000000000000, 0.000000000000000000 ) ) ;
#6038=CARTESIAN_POINT ( 'NONE',  ( 15.24356964374999990, 3.323476615752268604, -5.240624999385486760 ) ) ;
#6050=CARTESIAN_POINT ( 'NONE',  ( 27.00000000000047251, 3.464101615137479495, -7.331249998770944742 ) ) ;
#6051=CARTESIAN_POINT ( 'NONE',  ( 25.00000000000001421, 2.343145750507542147, 49.82535622836641664 ) ) ;
#6060=ORIENTED_EDGE ( 'NONE', *, *, #12969, .T. ) ;
#6063=FACE_OUTER_BOUND ( 'NONE', #11698, .T. ) ;
#6066=LINE ( 'NONE', #11021, #10606 ) ;
#6067=CARTESIAN_POINT ( 'NONE',  ( 24.98146486726017912, 0.000000000000000000, 164.3506311484184437 ) ) ;
#6077=CARTESIAN_POINT ( 'NONE',  ( 15.24356964374999990, 0.000000000000000000, -0.1406249993854691294 ) ) ;
#6082=ORIENTED_EDGE ( 'NONE', *, *, #11242, .F. ) ;
#6084=CARTESIAN_POINT ( 'NONE',  ( 37.40967911200478824, 3.604726614523243278, 165.9265627999972992 ) ) ;
#6085=AXIS2_PLACEMENT_3D ( 'NONE', #5613, #32141, #17198 ) ;
#6092=CARTESIAN_POINT ( 'NONE',  ( 31.34102887711597774, 6.928203230275506996, 168.1985009298100522 ) ) ;
#6094=CARTESIAN_POINT ( 'NONE',  ( 28.31976137920325698, -5.196152422706638241, 168.0863951450442642 ) ) ;
#6106=CARTESIAN_POINT ( 'NONE',  ( 36.87697111800645899, 7.347880794884117764E-16, 162.6323308142347059 ) ) ;
#6107=CARTESIAN_POINT ( 'NONE',  ( 23.99999999999999645, 5.196152422706631135, -4.143749998770957177 ) ) ;
#6110=CARTESIAN_POINT ( 'NONE',  ( 31.32141883499775403, -6.928203230275506996, 167.9743571227394341 ) ) ;
#6114=AXIS2_PLACEMENT_3D ( 'NONE', #6558, #18704, #6945 ) ;
#6122=CARTESIAN_POINT ( 'NONE',  ( 24.36704836432882004, -3.604726614523240613, 160.1224666319704681 ) ) ;
#6123=CARTESIAN_POINT ( 'NONE',  ( 21.00000000000000000, 6.646953231504538984, -3.065624999385470062 ) ) ;
#6128=VERTEX_POINT ( 'NONE', #10832 ) ;
#6129=CARTESIAN_POINT ( 'NONE',  ( 18.12178482187500350, -4.985214923628407568, -4.115624999385475213 ) ) ;
#6137=CARTESIAN_POINT ( 'NONE',  ( 36.72335912141372205, 3.464101615137755275, 160.8765376588480080 ) ) ;
#6142=CARTESIAN_POINT ( 'NONE',  ( 15.24356964375000167, -3.323476615752272600, -3.365624999385477878 ) ) ;
#6147=EDGE_CURVE ( 'NONE', #22401, #20504, #9295, .T. ) ;
#6148=VERTEX_POINT ( 'NONE', #8187 ) ;
#6149=CARTESIAN_POINT ( 'NONE',  ( 20.99999999999999645, -6.928203230275506996, -0.7312499987709595306 ) ) ;
#6152=CARTESIAN_POINT ( 'NONE',  ( 23.99999999999999645, 5.196152422706631135, -5.943749998770952558 ) ) ;
#6153=ADVANCED_FACE ( 'NONE', ( #17461 ), #33955, .T. ) ;
#6154=CARTESIAN_POINT ( 'NONE',  ( 24.44058602227215005, -3.604726614523244610, 160.9630059084853997 ) ) ;
#6160=CARTESIAN_POINT ( 'NONE',  ( 15.00000000000000355, 7.347880794884112834E-16, -8.000000000000000000 ) ) ;
#6169=CARTESIAN_POINT ( 'NONE',  ( 26.99999999999999645, -3.464101615137751278, -7.912500000000003197 ) ) ;
#6172=ADVANCED_FACE ( 'NONE', ( #28445 ), #22963, .T. ) ;
#6175=CARTESIAN_POINT ( 'NONE',  ( 37.53224187524366329, 3.604726614523238837, 167.3274615941888044 ) ) ;
#6177=CARTESIAN_POINT ( 'NONE',  ( 33.62038311478219299, 5.196152422706631135, 159.8304993458455385 ) ) ;
#6183=CARTESIAN_POINT ( 'NONE',  ( 26.97716818855048260, 0.000000000000000000, 49.47706554351410801 ) ) ;
#6184=CARTESIAN_POINT ( 'NONE',  ( 18.12178482187499640, 4.985214923628404904, -6.065624999385454963 ) ) ;
#6187=CARTESIAN_POINT ( 'NONE',  ( 25.05010001456683710, 0.000000000000000000, 165.1351344719413419 ) ) ;
#6192=CARTESIAN_POINT ( 'NONE',  ( 24.36214585379926589, -3.604726614523244610, 160.0664306802028136 ) ) ;
#6204=CARTESIAN_POINT ( 'NONE',  ( 23.34314575050773044, -3.999999999999902744, 49.89769604716121876 ) ) ;
#6205=CARTESIAN_POINT ( 'NONE',  ( 24.94717877699287811, 0.000000000000000000, 166.7533875911436780 ) ) ;
#6206=CARTESIAN_POINT ( 'NONE',  ( 18.00000000000000355, -5.196152422706632912, -2.118749998770957710 ) ) ;
#6218=CARTESIAN_POINT ( 'NONE',  ( 23.87821517812500005, -4.985214923628404016, -6.740624999385463667 ) ) ;
#6220=CARTESIAN_POINT ( 'NONE',  ( 31.17679477432231394, -7.209453229046482114, 166.3212965449812657 ) ) ;
#6221=CARTESIAN_POINT ( 'NONE',  ( 33.96355885174396860, 5.196152422706637353, 163.7530159683574311 ) ) ;
#6222=CARTESIAN_POINT ( 'NONE',  ( 24.00000000000000000, -5.196152422706629359, -6.993749998770947940 ) ) ;
#6233=CARTESIAN_POINT ( 'NONE',  ( 18.12178482187499640, 4.985214923628404904, -4.378124999385474503 ) ) ;
#6262=CARTESIAN_POINT ( 'NONE',  ( 24.91286120328598841, 0.000000000000000000, 166.3611359287700395 ) ) ;
#6263=CARTESIAN_POINT ( 'NONE',  ( 23.87821517812499650, 4.985214923628404904, -0.2906249993854803648 ) ) ;
#6264=CARTESIAN_POINT ( 'NONE',  ( 15.00000000000000000, 0.000000000000000000, -7.649999999999989697 ) ) ;
#6274=CARTESIAN_POINT ( 'NONE',  ( 21.00000000000000000, -6.646953231504538984, -8.690624999385464733 ) ) ;
#6282=CARTESIAN_POINT ( 'NONE',  ( 24.94391043663983965, 3.604726614523240613, 166.7160302899652322 ) ) ;
#6288=CARTESIAN_POINT ( 'NONE',  ( 37.48648511030114605, -3.604726614523235284, 166.8044593776906197 ) ) ;
#6289=ORIENTED_EDGE ( 'NONE', *, *, #9460, .F. ) ;
#6290=CARTESIAN_POINT ( 'NONE',  ( 37.29858702344112231, 7.347880794884125653E-16, 167.4514226650291562 ) ) ;
#6298=VECTOR ( 'NONE', #12788, 1000.000000000000000 ) ;
#6307=DIRECTION ( 'NONE',  ( 0.000000000000000000, -1.000000000000000000, 0.000000000000000000 ) ) ;
#6308=CARTESIAN_POINT ( 'NONE',  ( 21.00000000000000355, 0.000000000000000000, 50.00000000000001421 ) ) ;
#6313=ORIENTED_EDGE ( 'NONE', *, *, #24239, .T. ) ;
#6318=CARTESIAN_POINT ( 'NONE',  ( 36.82628035898769525, 3.604726614523238837, 159.2582845396456719 ) ) ;
#6319=CARTESIAN_POINT ( 'NONE',  ( 18.12178482187500350, -4.985214923628407568, -1.078124999385476901 ) ) ;
#6322=EDGE_CURVE ( 'NONE', #20178, #10985, #19759, .T. ) ;
#6325=ORIENTED_EDGE ( 'NONE', *, *, #27983, .F. ) ;
#6326=CARTESIAN_POINT ( 'NONE',  ( 23.87821517812500005, -4.985214923628404016, -5.390624999385473792 ) ) ;
#6333=CARTESIAN_POINT ( 'NONE',  ( 36.83448269341698733, -3.464101615137751278, 162.1466858989149387 ) ) ;
#6337=EDGE_CURVE ( 'NONE', #22269, #17991, #7900, .T. ) ;
#6338=CARTESIAN_POINT ( 'NONE',  ( 23.87821517812499650, 4.985214923628404904, -7.603124999385480365 ) ) ;
#6348=CARTESIAN_POINT ( 'NONE',  ( 24.47326942580252407, 3.604726614523240613, 161.3365789202697727 ) ) ;
#6356=CARTESIAN_POINT ( 'NONE',  ( 26.99999999999999645, 7.347880794884117764E-16, -3.768749998770942966 ) ) ;
#6360=CARTESIAN_POINT ( 'NONE',  ( 26.99999999999999645, -3.464101615137751278, -6.112499999999988276 ) ) ;
#6362=CARTESIAN_POINT ( 'NONE',  ( 26.99999999999999645, 7.347880794884117764E-16, -1.968749998770946696 ) ) ;
#6364=CARTESIAN_POINT ( 'NONE',  ( 25.02725311564228505, 3.604726614523236616, 167.6686414700154444 ) ) ;
#6369=VERTEX_POINT ( 'NONE', #21064 ) ;
#6370=CARTESIAN_POINT ( 'NONE',  ( 33.95048549033182184, -5.196152422706635576, 163.6035867636436478 ) ) ;
#6372=CARTESIAN_POINT ( 'NONE',  ( 18.12178482187500350, -4.985214923628407568, -6.815624999385455851 ) ) ;
#6379=CARTESIAN_POINT ( 'NONE',  ( 36.82137784845814821, 3.604726614523243278, 159.2022485878779889 ) ) ;
#6395=CARTESIAN_POINT ( 'NONE',  ( 28.20742792136773858, 5.407089921784862696, 168.1997419705030552 ) ) ;
#6396=CARTESIAN_POINT ( 'NONE',  ( 24.00000000000000000, -5.196152422706629359, -3.393749998770956289 ) ) ;
#6406=CARTESIAN_POINT ( 'NONE',  ( 36.82301201863464968, 7.646167579472015790E-16, 159.2209272384671976 ) ) ;
#6407=CARTESIAN_POINT ( 'NONE',  ( 26.75643035624999655, 7.049594010296217766E-16, -9.365624999385479654 ) ) ;
#6409=CARTESIAN_POINT ( 'NONE',  ( 27.93288733171263516, 5.407089921784862696, 165.0617286715140608 ) ) ;
#6410=CARTESIAN_POINT ( 'NONE',  ( 27.92756053683882911, -5.196152422706638241, 163.6035190036313622 ) ) ;
#6411=CARTESIAN_POINT ( 'NONE',  ( 37.10575494261148322, 3.464101615138019508, 165.2473418955011937 ) ) ;
#6415=( BOUNDED_CURVE ( )  B_SPLINE_CURVE ( 2, ( #2877, #14450, #17118, #5531, #35, #11600, #25449 ),
 .UNSPECIFIED., .F., .F. ) 
 B_SPLINE_CURVE_WITH_KNOTS ( ( 3, 2, 2, 3 ),
 ( 0.000000000000000000, 0.007246376811594299264, 0.01449275362318859853, 0.02173913043478289606 ),
 .UNSPECIFIED. ) 
 CURVE ( )  GEOMETRIC_REPRESENTATION_ITEM ( )  RATIONAL_B_SPLINE_CURVE ( ( 1.000000000000000000, 0.8660254037844387076, 1.000000000000000000, 0.8660254037844387076, 1.000000000000000000, 0.8660254037844333785, 1.000000000000005329 ) ) 
 REPRESENTATION_ITEM ( '' )  );
#6423=CARTESIAN_POINT ( 'NONE',  ( 15.24356964375000167, -3.323476615752272600, -4.265624999385501326 ) ) ;
#6438=CARTESIAN_POINT ( 'NONE',  ( 34.13799077639428958, -5.407089921784855591, 164.3494578665133474 ) ) ;
#6450=CARTESIAN_POINT ( 'NONE',  ( 28.18618370907300275, -5.407089921784859143, 167.9569195128432000 ) ) ;
#6452=CARTESIAN_POINT ( 'NONE',  ( 18.12178482187500350, -4.985214923628407568, -2.315624999385479388 ) ) ;
#6453=VECTOR ( 'NONE', #1858, 1000.000000000000000 ) ;
#6458=EDGE_CURVE ( 'NONE', #29003, #33644, #20970, .T. ) ;
#6459=CARTESIAN_POINT ( 'NONE',  ( 31.07629330841286830, -6.928203230275514990, 165.1725595331320449 ) ) ;
#6460=DIRECTION ( 'NONE',  ( 0.08715574274765150453, 0.000000000000000000, 0.9961946980917461003 ) ) ;
#6463=ORIENTED_EDGE ( 'NONE', *, *, #26275, .F. ) ;
#6466=EDGE_CURVE ( 'NONE', #25042, #8199, #29757, .T. ) ;
#6467=CARTESIAN_POINT ( 'NONE',  ( 15.24356964374999990, 3.323476615752268604, -1.978124999385461935 ) ) ;
#6470=CARTESIAN_POINT ( 'NONE',  ( 21.00000000000000000, -6.928203230275506996, -7.031249998770932486 ) ) ;
#6475=CARTESIAN_POINT ( 'NONE',  ( 24.71512661192725702, -3.604726614523244610, 164.1010192074743657 ) ) ;
#6482=CARTESIAN_POINT ( 'NONE',  ( 28.13389026342440857, 5.407089921784856479, 167.3592026939881237 ) ) ;
#6499=CARTESIAN_POINT ( 'NONE',  ( 31.41211527974097706, -7.209453229046482114, 169.0110222298289671 ) ) ;
#6503=ORIENTED_EDGE ( 'NONE', *, *, #13571, .T. ) ;
#6508=CARTESIAN_POINT ( 'NONE',  ( 18.12178482187499640, 4.985214923628404904, -4.828124999385480010 ) ) ;
#6512=ORIENTED_EDGE ( 'NONE', *, *, #22570, .F. ) ;
#6513=CARTESIAN_POINT ( 'NONE',  ( 23.87821517812499650, 4.985214923628404904, -5.690624999385468286 ) ) ;
#6514=B_SPLINE_CURVE_WITH_KNOTS ( 'NONE', 1,
 ( #15281, #1236 ),
 .UNSPECIFIED., .F., .F.,
 ( 2, 2 ),
 ( 0.000000000000000000, 1.000000000000000000 ),
 .UNSPECIFIED. ) ;
#6523=CARTESIAN_POINT ( 'NONE',  ( 24.86707295490388958, -3.464101615137757051, 163.0431256071730104 ) ) ;
#6527=CARTESIAN_POINT ( 'NONE',  ( 26.75643035624999655, 7.049594010296217766E-16, -7.228124999385493687 ) ) ;
#6547=ORIENTED_EDGE ( 'NONE', *, *, #24892, .F. ) ;
#6548=CARTESIAN_POINT ( 'NONE',  ( 26.99999999999999645, 7.347880794884117764E-16, -6.525000000000003020 ) ) ;
#6552=CARTESIAN_POINT ( 'NONE',  ( 24.95534962787547073, -3.604726614523240613, 166.8467808440897500 ) ) ;
#6558=CARTESIAN_POINT ( 'NONE',  ( 20.99999999999999645, 0.000000000000000000, -8.000000000000000000 ) ) ;
#6561=CARTESIAN_POINT ( 'NONE',  ( 23.87821517812499650, 4.985214923628404904, -7.040624999385459049 ) ) ;
#6564=FACE_OUTER_BOUND ( 'NONE', #25971, .T. ) ;
#6566=VECTOR ( 'NONE', #18369, 1000.000000000000000 ) ;
#6569=CARTESIAN_POINT ( 'NONE',  ( 37.38683221308021842, 7.347880794884117764E-16, 168.4600697980714017 ) ) ;
#6582=CARTESIAN_POINT ( 'NONE',  ( 37.52733936471412335, 3.604726614523243278, 167.2714256424211499 ) ) ;
#6594=CARTESIAN_POINT ( 'NONE',  ( 36.89818384675449181, -3.604726614523235284, 160.0801451655713379 ) ) ;
#6595=CARTESIAN_POINT ( 'NONE',  ( 19.00081571707362116, 5.492723647597327563, -10.12707781181606492 ) ) ;
#6597=CARTESIAN_POINT ( 'NONE',  ( 37.29201885929546734, 3.604726614523243278, 164.5816999575734201 ) ) ;
#6599=CARTESIAN_POINT ( 'NONE',  ( 24.89321967762106169, 0.000000000000000000, 163.3419840153761982 ) ) ;
#6600=CARTESIAN_POINT ( 'NONE',  ( 15.00000000000000000, 0.000000000000000000, -6.750000000000006217 ) ) ;
#6608=ADVANCED_FACE ( 'NONE', ( #36005 ), #21437, .T. ) ;
#6610=CARTESIAN_POINT ( 'NONE',  ( 18.12178482187499640, 4.985214923628404904, -3.928124999385496086 ) ) ;
#6620=FACE_OUTER_BOUND ( 'NONE', #26973, .T. ) ;
#6625=CARTESIAN_POINT ( 'NONE',  ( 24.75271252598717808, 3.604726614523236616, 164.5306281710264216 ) ) ;
#6628=CARTESIAN_POINT ( 'NONE',  ( 20.99999999999999645, -6.928203230275506996, -4.837499999999994138 ) ) ;
#6638=CARTESIAN_POINT ( 'NONE',  ( 31.26013745332475224, -7.209453229046475009, 167.2739077250314779 ) ) ;
#6639=CARTESIAN_POINT ( 'NONE',  ( 15.24356964374999990, 0.000000000000000000, -2.840624999385477079 ) ) ;
#6641=EDGE_CURVE ( 'NONE', #34104, #16979, #1355, .T. ) ;
#6648=ORIENTED_EDGE ( 'NONE', *, *, #4990, .F. ) ;
#6651=CARTESIAN_POINT ( 'NONE',  ( 15.24356964374999990, 0.000000000000000000, -2.390624999385471128 ) ) ;
#6653=CARTESIAN_POINT ( 'NONE',  ( 18.00000000000000000, 5.196152422706630247, -8.118749998770963927 ) ) ;
#6660=CARTESIAN_POINT ( 'NONE',  ( 37.28548217858939040, -3.604726614523238837, 164.5069853552165284 ) ) ;
#6666=CARTESIAN_POINT ( 'NONE',  ( 31.16208724273364084, 7.209453229046475009, 166.1531886896782737 ) ) ;
#6667=ORIENTED_EDGE ( 'NONE', *, *, #9927, .F. ) ;
#6682=FACE_OUTER_BOUND ( 'NONE', #9451, .T. ) ;
#6686=DIRECTION ( 'NONE',  ( 1.000000000000000000, 0.000000000000000000, 0.000000000000000000 ) ) ;
#6688=CARTESIAN_POINT ( 'NONE',  ( 16.50512534395675601, 3.755008844408135094, -7.999999999999996447 ) ) ;
#6692=EDGE_LOOP ( 'NONE', ( #6648, #17752, #23113, #17056 ) ) ;
#6697=CARTESIAN_POINT ( 'NONE',  ( 21.00000000000000000, -6.646953231504538984, -3.740624999385479654 ) ) ;
#6701=ORIENTED_EDGE ( 'NONE', *, *, #32582, .T. ) ;
#6702=CARTESIAN_POINT ( 'NONE',  ( 18.12178482187500350, -4.985214923628407568, -4.565624999385481608 ) ) ;
#6709=CARTESIAN_POINT ( 'NONE',  ( 30.59584727662355164, 6.928203230275506996, 159.6810362611256267 ) ) ;
#6714=CARTESIAN_POINT ( 'NONE',  ( 26.75643035624999655, 3.323476615752271268, -7.190624999385489602 ) ) ;
#6715=CARTESIAN_POINT ( 'NONE',  ( 15.00000000000000000, 0.000000000000000000, -2.250000000000001776 ) ) ;
#6720=EDGE_CURVE ( 'NONE', #20504, #34009, #12669, .T. ) ;
#6723=CARTESIAN_POINT ( 'NONE',  ( 36.81484116775207127, -3.604726614523238837, 159.1275339855211257 ) ) ;
#6728=CARTESIAN_POINT ( 'NONE',  ( 20.99999999999999645, -6.928203230275506996, -1.181249998770955045 ) ) ;
#6736=CARTESIAN_POINT ( 'NONE',  ( 15.00000000000000000, 0.000000000000000000, -7.200000000000011724 ) ) ;
#6739=CARTESIAN_POINT ( 'NONE',  ( 37.32960477335537774, -3.604726614523235284, 165.0113089211254760 ) ) ;
#6747=CARTESIAN_POINT ( 'NONE',  ( 36.55994210376140785, -3.464101615138027057, 159.0086725999260011 ) ) ;
#6749=CARTESIAN_POINT ( 'NONE',  ( 23.87821517812499650, 4.985214923628404904, -9.290624999385460825 ) ) ;
#6752=CARTESIAN_POINT ( 'NONE',  ( 30.77233765568754720, -6.928203230275506996, 161.6983305247614453 ) ) ;
#6756=CARTESIAN_POINT ( 'NONE',  ( 25.21678537267883868, 0.000000000000000000, 167.0403568332661450 ) ) ;
#6768=CARTESIAN_POINT ( 'NONE',  ( 37.48485094012463748, 7.646167579472024665E-16, 166.7857807271014394 ) ) ;
#6777=CARTESIAN_POINT ( 'NONE',  ( 24.69711925643884598, 0.000000000000000000, 161.1005459446697614 ) ) ;
#6780=CARTESIAN_POINT ( 'NONE',  ( 18.00000000000000000, 5.196152422706630247, -5.475000000000007638 ) ) ;
#6783=CARTESIAN_POINT ( 'NONE',  ( 26.75643035624999655, -3.323476615752267715, -9.853124999385466154 ) ) ;
#6785=CARTESIAN_POINT ( 'NONE',  ( 34.17230835010118994, -5.407089921784861808, 164.7417095288869859 ) ) ;
#6786=CARTESIAN_POINT ( 'NONE',  ( 25.00761158997735478, 3.464101615137757051, 164.6494895566215746 ) ) ;
#6797=CARTESIAN_POINT ( 'NONE',  ( 26.75643035624999655, -3.323476615752267715, -6.815624999385487826 ) ) ;
#6809=EDGE_CURVE ( 'NONE', #1170, #35303, #134, .T. ) ;
#6811=CARTESIAN_POINT ( 'NONE',  ( 27.89856975800574546, 5.407089921784856479, 164.6694770091404223 ) ) ;
#6815=DIRECTION ( 'NONE',  ( 0.9961946980917462113, 0.000000000000000000, -0.08715574274765118534 ) ) ;
#6823=CARTESIAN_POINT ( 'NONE',  ( 34.29487111334006499, -5.407089921784855591, 166.1426083230784911 ) ) ;
#6824=CARTESIAN_POINT ( 'NONE',  ( 26.75643035624999655, -3.323476615752267715, -2.653124999385471305 ) ) ;
#6837=CARTESIAN_POINT ( 'NONE',  ( 26.75643035624999655, 7.049594010296217766E-16, -2.615624999385474325 ) ) ;
#6840=CARTESIAN_POINT ( 'NONE',  ( 15.00000000000000000, 3.464101615137752166, -9.431249998770962151 ) ) ;
#6850=CARTESIAN_POINT ( 'NONE',  ( 31.07874456373121319, 7.209453229046482114, 165.2005775096280615 ) ) ;
#6858=CARTESIAN_POINT ( 'NONE',  ( 24.95534962787547073, -3.604726614523240613, 166.8467808440897500 ) ) ;
#6859=ORIENTED_EDGE ( 'NONE', *, *, #26272, .T. ) ;
#6860=( BOUNDED_CURVE ( )  B_SPLINE_CURVE ( 2, ( #11139, #34071, #28199, #24797, #19692, #24975, #25173 ),
 .UNSPECIFIED., .F., .F. ) 
 B_SPLINE_CURVE_WITH_KNOTS ( ( 3, 2, 2, 3 ),
 ( 0.06521739130434746345, 0.07246376811594175404, 0.07971014492753603076, 0.08695652173913032135 ),
 .UNSPECIFIED. ) 
 CURVE ( )  GEOMETRIC_REPRESENTATION_ITEM ( )  RATIONAL_B_SPLINE_CURVE ( ( 1.000000000000006661, 0.8660254037844320463, 1.000000000000000000, 0.8660254037844387076, 1.000000000000000000, 0.8660254037844407060, 0.9999999999999980016 ) ) 
 REPRESENTATION_ITEM ( '' )  );
#6864=ADVANCED_FACE ( 'NONE', ( #17001 ), #28916, .T. ) ;
#6878=CARTESIAN_POINT ( 'NONE',  ( 25.22171936664797798, 0.000000000000000000, 169.8914008901326724 ) ) ;
#6879=CARTESIAN_POINT ( 'NONE',  ( 27.75760683848089982, 5.196152422706636465, 161.6609393423525205 ) ) ;
#6888=CARTESIAN_POINT ( 'NONE',  ( 26.75643035624999655, -3.323476615752267715, -5.015624999385472904 ) ) ;
#6893=CARTESIAN_POINT ( 'NONE',  ( 15.24356964375000167, -3.323476615752272600, -6.403124999385489069 ) ) ;
#6903=CARTESIAN_POINT ( 'NONE',  ( 24.66770419336863185, 0.000000000000000000, 160.7643302352881278 ) ) ;
#6908=CARTESIAN_POINT ( 'NONE',  ( 23.87821517812500005, -4.985214923628404016, -7.753124999385491378 ) ) ;
#6917=CARTESIAN_POINT ( 'NONE',  ( 36.89328133622495898, -3.604726614523238837, 160.0241092138036834 ) ) ;
#6929=CIRCLE ( 'NONE', #11758, 3.999999999999996447 ) ;
#6931=CARTESIAN_POINT ( 'NONE',  ( 24.00000000000000000, -5.196152422706629359, -6.149999999999988809 ) ) ;
#6933=CARTESIAN_POINT ( 'NONE',  ( 23.99999999999999645, 5.196152422706631135, -3.299999999999997158 ) ) ;
#6935=ADVANCED_FACE ( 'NONE', ( #3324 ), #9019, .T. ) ;
#6938=CARTESIAN_POINT ( 'NONE',  ( 37.21848120135211957, 3.604726614523238837, 163.7411606810585170 ) ) ;
#6939=CARTESIAN_POINT ( 'NONE',  ( 26.99999999999995737, 3.464101615137778811, -1.987499999999999156 ) ) ;
#6943=ORIENTED_EDGE ( 'NONE', *, *, #28922, .F. ) ;
#6945=DIRECTION ( 'NONE',  ( 1.000000000000000000, 0.000000000000000000, 0.000000000000000000 ) ) ;
#6946=CARTESIAN_POINT ( 'NONE',  ( 18.12178482187500350, -4.985214923628407568, -1.415624999385467486 ) ) ;
#6949=CARTESIAN_POINT ( 'NONE',  ( 15.24356964375000167, -3.323476615752272600, -9.553124999385460114 ) ) ;
#6957=FACE_OUTER_BOUND ( 'NONE', #25657, .T. ) ;
#6958=CARTESIAN_POINT ( 'NONE',  ( 28.15961270201155742, 5.196152422706630247, 166.2558873885250250 ) ) ;
#6963=LINE ( 'NONE', #30069, #2196 ) ;
#6971=CARTESIAN_POINT ( 'NONE',  ( 28.12898775289485442, 5.407089921784862696, 167.3031667422204691 ) ) ;
#6979=( BOUNDED_CURVE ( )  B_SPLINE_CURVE ( 2, ( #10572, #4693, #36157, #27638, #24791, #7736, #30857 ),
 .UNSPECIFIED., .F., .F. ) 
 B_SPLINE_CURVE_WITH_KNOTS ( ( 3, 2, 2, 3 ),
 ( 0.3695652173913039351, 0.3768115942028982257, 0.3840579710144925163, 0.3913043478260868069 ),
 .UNSPECIFIED. ) 
 CURVE ( )  GEOMETRIC_REPRESENTATION_ITEM ( )  RATIONAL_B_SPLINE_CURVE ( ( 1.000000000000007105, 0.8660254037844313801, 1.000000000000000000, 0.8660254037844387076, 1.000000000000000000, 0.8660254037844418162, 0.9999999999999968914 ) ) 
 REPRESENTATION_ITEM ( '' )  );
#6985=CARTESIAN_POINT ( 'NONE',  ( 30.69144623189632526, 7.209453229046475009, 160.7737373199828426 ) ) ;
#6986=ORIENTED_EDGE ( 'NONE', *, *, #32567, .T. ) ;
#6987=CARTESIAN_POINT ( 'NONE',  ( 18.12178482187500350, -4.985214923628407568, -9.965624999385468641 ) ) ;
#6989=CARTESIAN_POINT ( 'NONE',  ( 27.78908035617901717, -5.407089921784865361, 163.4180074196626720 ) ) ;
#6990=CARTESIAN_POINT ( 'NONE',  ( 24.73960768102833185, -3.464101615137761048, 161.5861908599894718 ) ) ;
#6995=ORIENTED_EDGE ( 'NONE', *, *, #36066, .F. ) ;
#7000=CARTESIAN_POINT ( 'NONE',  ( 18.12178482187499640, 4.985214923628404904, -6.178124999385470772 ) ) ;
#7007=EDGE_CURVE ( 'NONE', #17676, #3429, #4011, .T. ) ;
#7009=DIRECTION ( 'NONE',  ( 0.9961946980917462113, 0.000000000000000000, -0.08715574274765118534 ) ) ;
#7014=CARTESIAN_POINT ( 'NONE',  ( 34.03340388509710834, 5.407089921784857367, 163.1540242288032232 ) ) ;
#7019=CARTESIAN_POINT ( 'NONE',  ( 20.99999999999999645, -6.928203230275506996, -5.681249998770944387 ) ) ;
#7028=CARTESIAN_POINT ( 'NONE',  ( 28.06852345636367119, -5.407089921784859143, 166.6120566704193493 ) ) ;
#7029=CARTESIAN_POINT ( 'NONE',  ( 15.24356964374999990, 0.000000000000000000, -3.290624999385455496 ) ) ;
#7031=CARTESIAN_POINT ( 'NONE',  ( 31.16453849805197507, -6.928203230275506996, 166.1812066661742904 ) ) ;
#7035=FACE_OUTER_BOUND ( 'NONE', #35435, .T. ) ;
#7042=CARTESIAN_POINT ( 'NONE',  ( 18.12178482187499640, 4.985214923628404904, -2.015624999385456917 ) ) ;
#7044=CARTESIAN_POINT ( 'NONE',  ( 15.24356964374999990, 3.323476615752268604, -0.2906249993854697622 ) ) ;
#7051=CARTESIAN_POINT ( 'NONE',  ( 31.01991443737654564, -7.209453229046482114, 164.5281460884161220 ) ) ;
#7057=CARTESIAN_POINT ( 'NONE',  ( 28.17311034766084887, 5.407089921784856479, 167.8074903081294167 ) ) ;
#7066=ADVANCED_FACE ( 'NONE', ( #29285 ), #476, .T. ) ;
#7072=CARTESIAN_POINT ( 'NONE',  ( 15.02283181144952628, 7.347880794884122694E-16, 50.52293445648592751 ) ) ;
#7075=( BOUNDED_CURVE ( )  B_SPLINE_CURVE ( 2, ( #11841, #3308, #23410, #460, #6152, #34590, #20200 ),
 .UNSPECIFIED., .F., .F. ) 
 B_SPLINE_CURVE_WITH_KNOTS ( ( 3, 2, 2, 3 ),
 ( 0.5217391304347814840, 0.5289855072463758301, 0.5362318840579701762, 0.5434782608695644113 ),
 .UNSPECIFIED. ) 
 CURVE ( )  GEOMETRIC_REPRESENTATION_ITEM ( )  RATIONAL_B_SPLINE_CURVE ( ( 1.000000000000020428, 0.8660254037844181685, 1.000000000000000000, 0.8660254037844387076, 1.000000000000000000, 0.8660254037844530295, 0.9999999999999856781 ) ) 
 REPRESENTATION_ITEM ( '' )  );
#7076=DIRECTION ( 'NONE',  ( 0.08715574274765150453, 0.000000000000000000, 0.9961946980917461003 ) ) ;
#7079=CARTESIAN_POINT ( 'NONE',  ( 24.77555942491173369, 0.000000000000000000, 161.9971211729523475 ) ) ;
#7086=CARTESIAN_POINT ( 'NONE',  ( 15.24356964375000167, -3.323476615752272600, -5.165624999385460825 ) ) ;
#7096=CARTESIAN_POINT ( 'NONE',  ( 36.64491895294083434, 3.464101615137755275, 159.9799624305654220 ) ) ;
#7100=CARTESIAN_POINT ( 'NONE',  ( 18.12178482187500350, -4.985214923628407568, -6.028124999385486404 ) ) ;
#7101=CARTESIAN_POINT ( 'NONE',  ( 24.94224478302373527, 0.000000000000000000, 163.9023435342771506 ) ) ;
#7108=ORIENTED_EDGE ( 'NONE', *, *, #9183, .T. ) ;
#7113=LINE ( 'NONE', #15451, #35204 ) ;
#7115=CARTESIAN_POINT ( 'NONE',  ( 21.00000000000016342, 4.000000000000002665, 50.00000000000000000 ) ) ;
#7120=EDGE_LOOP ( 'NONE', ( #21216, #20886, #8745, #8788 ) ) ;
#7124=CARTESIAN_POINT ( 'NONE',  ( 27.89856975800574546, 5.407089921784856479, 164.6694770091404223 ) ) ;
#7129=ORIENTED_EDGE ( 'NONE', *, *, #7177, .F. ) ;
#7132=CARTESIAN_POINT ( 'NONE',  ( 23.87821517812500005, -4.985214923628404016, -1.340624999385475746 ) ) ;
#7135=FACE_OUTER_BOUND ( 'NONE', #14437, .T. ) ;
#7136=CARTESIAN_POINT ( 'NONE',  ( 15.24356964374999990, 0.000000000000000000, -8.240624999385465443 ) ) ;
#7142=CARTESIAN_POINT ( 'NONE',  ( 31.20375858228842603, -6.928203230275506996, 166.6294942803155550 ) ) ;
#7147=CARTESIAN_POINT ( 'NONE',  ( 15.24356964374999990, 3.323476615752268604, -0.7406249993854976399 ) ) ;
#7153=CARTESIAN_POINT ( 'NONE',  ( 24.74941270219519751, -3.464101615138124757, 161.6982627647491597 ) ) ;
#7155=CARTESIAN_POINT ( 'NONE',  ( 34.17230835010118994, -5.407089921784861808, 164.7417095288869859 ) ) ;
#7163=EDGE_CURVE ( 'NONE', #31911, #22619, #5229, .T. ) ;
#7171=CARTESIAN_POINT ( 'NONE',  ( 15.00000000000000178, -3.464101615137757051, -1.312499999999990230 ) ) ;
#7173=CARTESIAN_POINT ( 'NONE',  ( 24.66936984698473623, 3.604726614523240613, 163.5780169909762094 ) ) ;
#7174=CARTESIAN_POINT ( 'NONE',  ( 30.86058284511243599, 6.928203230275514990, 162.7069776553549616 ) ) ;
#7177=EDGE_CURVE ( 'NONE', #11864, #24223, #14420, .T. ) ;
#7181=ORIENTED_EDGE ( 'NONE', *, *, #12144, .F. ) ;
#7182=AXIS2_PLACEMENT_3D ( 'NONE', #15901, #27447, #1478 ) ;
#7185=CARTESIAN_POINT ( 'NONE',  ( 24.97819652690671788, 3.464101615137507473, 164.3132738472399978 ) ) ;
#7188=CARTESIAN_POINT ( 'NONE',  ( 21.00000000000000000, -6.646953231504538984, -5.990624999385490312 ) ) ;
#7191=CARTESIAN_POINT ( 'NONE',  ( 15.00000000000000000, 0.000000000000000000, -6.693749998770953447 ) ) ;
#7194=VECTOR ( 'NONE', #18538, 1000.000000000000000 ) ;
#7202=CARTESIAN_POINT ( 'NONE',  ( 24.83442103481310781, 0.000000000000000000, 165.4645607004874535 ) ) ;
#7205=CARTESIAN_POINT ( 'NONE',  ( 15.00000000000000000, 0.000000000000000000, -4.950000000000009948 ) ) ;
#7208=CARTESIAN_POINT ( 'NONE',  ( 14.99999999999982414, 3.464101615137652246, -2.231249998770932219 ) ) ;
#7213=CARTESIAN_POINT ( 'NONE',  ( 24.72002912245681472, -3.604726614523240613, 164.1570551592420202 ) ) ;
#7214=CARTESIAN_POINT ( 'NONE',  ( 21.00000000000000000, 6.646953231504538984, -3.403124999385474858 ) ) ;
#7216=CARTESIAN_POINT ( 'NONE',  ( 37.37375885156096444, -3.464101615137755275, 168.3106405921333248 ) ) ;
#7223=EDGE_LOOP ( 'NONE', ( #18130, #12430, #29578, #27605 ) ) ;
#7226=CARTESIAN_POINT ( 'NONE',  ( 23.87821517812499650, 4.985214923628404904, -0.7406249993854585600 ) ) ;
#7228=CARTESIAN_POINT ( 'NONE',  ( 23.99999999999999645, 5.196152422706631135, -9.093749998770938703 ) ) ;
#7234=CARTESIAN_POINT ( 'NONE',  ( 27.77600699476686330, 5.407089921784862696, 163.2685782149489171 ) ) ;
#7241=ORIENTED_EDGE ( 'NONE', *, *, #10058, .T. ) ;
#7242=CARTESIAN_POINT ( 'NONE',  ( 24.00000000000000000, -5.196152422706629359, -5.250000000000004441 ) ) ;
#7249=ORIENTED_EDGE ( 'NONE', *, *, #24892, .T. ) ;
#7258=CYLINDRICAL_SURFACE ( 'NONE', #12111, 5.999999999999994671 ) ;
#7265=CARTESIAN_POINT ( 'NONE',  ( 26.75643035624999655, 3.323476615752271712, -4.940624999385510918 ) ) ;
#7268=CARTESIAN_POINT ( 'NONE',  ( 15.24356964374999990, 3.323476615752268604, -6.928124999385478766 ) ) ;
#7275=CARTESIAN_POINT ( 'NONE',  ( 27.58438479987706415, -5.196152422706632912, 159.6810023811194981 ) ) ;
#7300=AXIS2_PLACEMENT_3D ( 'NONE', #14421, #31662, #32033 ) ;
#7306=CARTESIAN_POINT ( 'NONE',  ( 37.13677269252619340, 7.646167579472015790E-16, 162.8072281515975135 ) ) ;
#7307=CARTESIAN_POINT ( 'NONE',  ( 18.00000000000000000, 5.196152422706630247, -1.874999999999987788 ) ) ;
#7309=ORIENTED_EDGE ( 'NONE', *, *, #21463, .F. ) ;
#7311=ORIENTED_EDGE ( 'NONE', *, *, #36224, .T. ) ;
#7312=ORIENTED_EDGE ( 'NONE', *, *, #30081, .T. ) ;
#7313=CARTESIAN_POINT ( 'NONE',  ( 36.64165061258780298, 7.347880794884117764E-16, 159.9426051293869477 ) ) ;
#7317=CARTESIAN_POINT ( 'NONE',  ( 26.75643035624999655, 7.049594010296217766E-16, -8.465624999385468641 ) ) ;
#7324=CARTESIAN_POINT ( 'NONE',  ( 25.22005371303187715, -3.464101615137757051, 167.0777141344445624 ) ) ;
#7330=VECTOR ( 'NONE', #3813, 1000.000000000000000 ) ;
#7331=CARTESIAN_POINT ( 'NONE',  ( 15.24356964374999990, 3.323476615752268604, -2.540624999385480809 ) ) ;
#7340=CARTESIAN_POINT ( 'NONE',  ( 37.33123894353190764, 3.604726614523243278, 165.0299875717147415 ) ) ;
#7343=EDGE_CURVE ( 'NONE', #23173, #8675, #12991, .T. ) ;
#7346=CARTESIAN_POINT ( 'NONE',  ( 21.00000000000000355, 0.000000000000000000, 50.00000000000001421 ) ) ;
#7356=CARTESIAN_POINT ( 'NONE',  ( 26.99999999999999645, -3.464101615137751278, -2.062499999999993339 ) ) ;
#7357=CARTESIAN_POINT ( 'NONE',  ( 30.78459393195788607, -7.209453229046482114, 161.8384204035683922 ) ) ;
#7358=CARTESIAN_POINT ( 'NONE',  ( 33.71516498491316582, -5.196152422706635576, 160.9138610787959465 ) ) ;
#7369=CARTESIAN_POINT ( 'NONE',  ( 18.12178482187500350, -4.985214923628407568, -7.378124999385477167 ) ) ;
#7382=CARTESIAN_POINT ( 'NONE',  ( 33.94189035521207387, -5.407089921784855591, 162.1080197958069107 ) ) ;
#7387=FACE_OUTER_BOUND ( 'NONE', #17940, .T. ) ;
#7392=CARTESIAN_POINT ( 'NONE',  ( 24.79846929092969887, -3.604726614523240613, 165.0536303875245778 ) ) ;
#7393=CARTESIAN_POINT ( 'NONE',  ( 26.75643035624999655, -3.323476615752267715, -5.353124999385477700 ) ) ;
#7397=CARTESIAN_POINT ( 'NONE',  ( 27.69224003142016954, -5.196152422706638241, 160.9137933187836609 ) ) ;
#7406=CARTESIAN_POINT ( 'NONE',  ( 15.24356964374999990, 3.323476615752268604, -4.228124999385472371 ) ) ;
#7410=CARTESIAN_POINT ( 'NONE',  ( 26.99999999999999645, 3.464101615137755275, -8.681249998770958598 ) ) ;
#7414=ORIENTED_EDGE ( 'NONE', *, *, #35342, .F. ) ;
#7418=CARTESIAN_POINT ( 'NONE',  ( 30.76498388983966237, 7.209453229046482114, 161.6142765964977741 ) ) ;
#7423=PRODUCT_DEFINITION ( 'UNKNOWN', '', #32950, #9257 ) ;
#7428=ORIENTED_EDGE ( 'NONE', *, *, #16906, .F. ) ;
#7440=LINE ( 'NONE', #16532, #28065 ) ;
#7443=FACE_OUTER_BOUND ( 'NONE', #5198, .T. ) ;
#7445=ORIENTED_EDGE ( 'NONE', *, *, #12185, .T. ) ;
#7450=CARTESIAN_POINT ( 'NONE',  ( 18.12178482187500350, -4.985214923628407568, -7.828124999385482674 ) ) ;
#7453=ORIENTED_EDGE ( 'NONE', *, *, #23541, .T. ) ;
#7454=CARTESIAN_POINT ( 'NONE',  ( 15.24356964375000167, -3.323476615752272600, -6.853124999385484806 ) ) ;
#7458=CARTESIAN_POINT ( 'NONE',  ( 27.70204505258639216, -5.196152422706632912, 161.0258652235433487 ) ) ;
#7478=EDGE_CURVE ( 'NONE', #24079, #22329, #19622, .T. ) ;
#7484=EDGE_CURVE ( 'NONE', #29149, #21861, #21895, .T. ) ;
#7487=CARTESIAN_POINT ( 'NONE',  ( 25.16449192692294545, 3.464101615137650025, 166.4426400131867751 ) ) ;
#7490=CARTESIAN_POINT ( 'NONE',  ( 31.00520690578787253, 7.209453229046475009, 164.3600382331131300 ) ) ;
#7497=CARTESIAN_POINT ( 'NONE',  ( 18.00000000000000000, 5.196152422706630247, -5.868749998770961263 ) ) ;
#7500=( GEOMETRIC_REPRESENTATION_CONTEXT ( 3 ) GLOBAL_UNCERTAINTY_ASSIGNED_CONTEXT ( ( #903 ) ) GLOBAL_UNIT_ASSIGNED_CONTEXT ( ( #4566, #10070, #33195 ) ) REPRESENTATION_CONTEXT ( 'NONE', 'WORKASPACE' ) );
#7502=CARTESIAN_POINT ( 'NONE',  ( 18.12178482187499640, 4.985214923628404904, -8.765624999385462246 ) ) ;
#7510=CARTESIAN_POINT ( 'NONE',  ( 25.33771396574120516, -3.464101615137757051, 168.4225769768684131 ) ) ;
#7515=EDGE_CURVE ( 'NONE', #25852, #19565, #24912, .T. ) ;
#7516=CARTESIAN_POINT ( 'NONE',  ( 26.75643035624999655, 3.323476615752271268, -2.240624999385472549 ) ) ;
#7520=ORIENTED_EDGE ( 'NONE', *, *, #26777, .F. ) ;
#7525=CARTESIAN_POINT ( 'NONE',  ( 24.87200694887302532, -3.604726614523244610, 165.8941696640395378 ) ) ;
#7526=AXIS2_PLACEMENT_3D ( 'NONE', #13681, #16709, #22024 ) ;
#7535=FACE_OUTER_BOUND ( 'NONE', #23386, .T. ) ;
#7538=CARTESIAN_POINT ( 'NONE',  ( 26.97716818855048260, 0.000000000000000000, 49.47706554351410801 ) ) ;
#7543=CARTESIAN_POINT ( 'NONE',  ( 15.00000000000000178, -3.464101615137757051, -1.762499999999985967 ) ) ;
#7544=CARTESIAN_POINT ( 'NONE',  ( 37.05669835387679711, 3.604726614523243278, 161.8919742727257187 ) ) ;
#7545=CARTESIAN_POINT ( 'NONE',  ( 30.76253263452132458, -6.928203230275514990, 161.5862586200017574 ) ) ;
#7550=ORIENTED_EDGE ( 'NONE', *, *, #17453, .T. ) ;
#7551=VERTEX_POINT ( 'NONE', #30425 ) ;
#7555=CARTESIAN_POINT ( 'NONE',  ( 15.24356964375000167, -3.323476615752272600, -6.515624999385480010 ) ) ;
#7558=ADVANCED_FACE ( 'NONE', ( #16025 ), #27574, .T. ) ;
#7559=CARTESIAN_POINT ( 'NONE',  ( 26.99999999999999645, 7.347880794884117764E-16, -7.424999999999987388 ) ) ;
#7568=CARTESIAN_POINT ( 'NONE',  ( 36.94394061169700905, 3.604726614523238837, 160.6031473820695226 ) ) ;
#7569=CARTESIAN_POINT ( 'NONE',  ( 28.19883278624800127, 5.196152422706630247, 166.7041750026663181 ) ) ;
#7571=CARTESIAN_POINT ( 'NONE',  ( 36.86716609684025059, 7.347880794884125653E-16, 162.5202589094750181 ) ) ;
#7572=CARTESIAN_POINT ( 'NONE',  ( 29.53112584896062032, 5.988803496771940793, 159.6272768299058669 ) ) ;
#7579=CARTESIAN_POINT ( 'NONE',  ( 37.29365302947196881, 7.646167579472015790E-16, 164.6003786081626572 ) ) ;
#7580=CARTESIAN_POINT ( 'NONE',  ( 23.87821517812500005, -4.985214923628404016, -5.840624999385479299 ) ) ;
#7582=CARTESIAN_POINT ( 'NONE',  ( 18.85832510013969454, 5.387298466171131395, -8.000000000000000000 ) ) ;
#7584=CARTESIAN_POINT ( 'NONE',  ( 37.38029553226704138, 3.464101615137759271, 168.3853551944901596 ) ) ;
#7587=CARTESIAN_POINT ( 'NONE',  ( 29.48995970988985604, 6.148715791637016537, 159.4803054849043917 ) ) ;
#7595=CARTESIAN_POINT ( 'NONE',  ( 18.12178482187499640, 4.985214923628404904, -3.815624999385480720 ) ) ;
#7598=CARTESIAN_POINT ( 'NONE',  ( 21.00000000000000000, 6.928203230275506996, -8.606249998770964638 ) ) ;
#7600=EDGE_LOOP ( 'NONE', ( #16594, #26037, #26562, #27503 ) ) ;
#7617=CARTESIAN_POINT ( 'NONE',  ( 24.00000000000000000, -5.196152422706629359, -2.493749998770944387 ) ) ;
#7621=DIRECTION ( 'NONE',  ( 0.000000000000000000, 0.000000000000000000, 1.000000000000000000 ) ) ;
#7633=ORIENTED_EDGE ( 'NONE', *, *, #17453, .F. ) ;
#7638=CARTESIAN_POINT ( 'NONE',  ( 15.24356964375000167, -3.323476615752272600, -6.515624999385480010 ) ) ;
#7643=CARTESIAN_POINT ( 'NONE',  ( 33.99951059573448475, -5.196152422706629359, 164.1639462825446003 ) ) ;
#7645=CARTESIAN_POINT ( 'NONE',  ( 25.14654753852813229, -3.604726614523244610, 169.0321829630285322 ) ) ;
#7668=CARTESIAN_POINT ( 'NONE',  ( 33.63672481644027812, -5.196152422706635576, 160.0172858505133604 ) ) ;
#7674=EDGE_LOOP ( 'NONE', ( #5556, #35476, #7550, #17939 ) ) ;
#7678=CARTESIAN_POINT ( 'NONE',  ( 30.98559686366965238, -7.209453229046475009, 164.1358944260424835 ) ) ;
#7679=CARTESIAN_POINT ( 'NONE',  ( 15.24356964374999990, 0.000000000000000000, -0.7031249993854904456 ) ) ;
#7684=ORIENTED_EDGE ( 'NONE', *, *, #25354, .T. ) ;
#7685=CARTESIAN_POINT ( 'NONE',  ( 26.99999999999999645, 3.464101615137755275, -5.531249998770956466 ) ) ;
#7686=CARTESIAN_POINT ( 'NONE',  ( 20.99999999999999645, 6.646953231504538984, -0.7031249993854685743 ) ) ;
#7694=CARTESIAN_POINT ( 'NONE',  ( 36.78872592836736288, 7.347880794884125653E-16, 161.6236836811924604 ) ) ;
#7695=AXIS2_PLACEMENT_3D ( 'NONE', #15820, #33431, #19051 ) ;
#7696=CARTESIAN_POINT ( 'NONE',  ( 25.09912511996950713, 0.000000000000000000, 165.6954939908422944 ) ) ;
#7700=CARTESIAN_POINT ( 'NONE',  ( 15.24356964375000167, -3.323476615752272600, -2.465624999385486849 ) ) ;
#7706=CARTESIAN_POINT ( 'NONE',  ( 27.74126513682283601, -5.196152422706632912, 161.4741528376846134 ) ) ;
#7709=DIRECTION ( 'NONE',  ( 0.08715574274765150453, 0.000000000000000000, 0.9961946980917461003 ) ) ;
#7710=CARTESIAN_POINT ( 'NONE',  ( 37.17109026623309376, 7.646167579472024665E-16, 163.1994798139711520 ) ) ;
#7723=CARTESIAN_POINT ( 'NONE',  ( 20.99999999999999645, -6.928203230275506996, -6.131249998770972098 ) ) ;
#7724=ORIENTED_EDGE ( 'NONE', *, *, #17525, .F. ) ;
#7725=CARTESIAN_POINT ( 'NONE',  ( 26.99999999999999645, 7.347880794884117764E-16, -2.475000000000004974 ) ) ;
#7727=CARTESIAN_POINT ( 'NONE',  ( 33.91084112185822619, 5.407089921784862696, 161.7531254346117464 ) ) ;
#7728=CARTESIAN_POINT ( 'NONE',  ( 27.75760683848089982, 5.196152422706636465, 161.6609393423525205 ) ) ;
#7730=DIRECTION ( 'NONE',  ( 0.08715574274765150453, 0.000000000000000000, 0.9961946980917461003 ) ) ;
#7736=CARTESIAN_POINT ( 'NONE',  ( 15.00000000000008171, -3.464101615137802348, -4.012499999999994849 ) ) ;
#7738=CARTESIAN_POINT ( 'NONE',  ( 21.00000000000000000, 6.646953231504538984, -9.365624999385474325 ) ) ;
#7741=CARTESIAN_POINT ( 'NONE',  ( 34.43419986258128773, 5.196152422706637353, 169.1324673380528623 ) ) ;
#7752=CARTESIAN_POINT ( 'NONE',  ( 27.71554269823568362, -5.407089921784859143, 162.5774681431477404 ) ) ;
#7759=CYLINDRICAL_SURFACE ( 'NONE', #14640, 6.000000000000001776 ) ;
#7763=CARTESIAN_POINT ( 'NONE',  ( 15.00000000000000000, 0.000000000000000000, -0.3937499987709536242 ) ) ;
#7764=ORIENTED_EDGE ( 'NONE', *, *, #35157, .T. ) ;
#7765=CARTESIAN_POINT ( 'NONE',  ( 24.71676078210377625, 0.000000000000000000, 164.1196978580636028 ) ) ;
#7767=CARTESIAN_POINT ( 'NONE',  ( 26.75643035624999655, 3.323476615752271712, -5.728124999385479477 ) ) ;
#7770=CARTESIAN_POINT ( 'NONE',  ( 17.59114475875851014, 4.706365066813837039, -7.999999999999998224 ) ) ;
#7771=FACE_OUTER_BOUND ( 'NONE', #23621, .T. ) ;
#7777=EDGE_LOOP ( 'NONE', ( #911, #8927, #21930, #4269 ) ) ;
#7781=CARTESIAN_POINT ( 'NONE',  ( 26.75643035624999655, -3.323476615752267715, -3.553124999385494753 ) ) ;
#7784=CARTESIAN_POINT ( 'NONE',  ( 26.75643035624999655, -3.323476615752267715, -2.315624999385466509 ) ) ;
#7799=EDGE_CURVE ( 'NONE', #35303, #34054, #19538, .T. ) ;
#7818=CARTESIAN_POINT ( 'NONE',  ( 21.00000000000000000, -6.928203230275506996, -9.787500000000010303 ) ) ;
#7824=CARTESIAN_POINT ( 'NONE',  ( 26.75643035624999655, 3.323476615752271712, -6.290624999385498128 ) ) ;
#7832=DIRECTION ( 'NONE',  ( 0.000000000000000000, 0.000000000000000000, 1.000000000000000000 ) ) ;
#7838=DIRECTION ( 'NONE',  ( 1.000000000000000000, 0.000000000000000000, 0.000000000000000000 ) ) ;
#7843=CARTESIAN_POINT ( 'NONE',  ( 30.93902301358532014, 6.928203230275514990, 163.6035528836375477 ) ) ;
#7852=CARTESIAN_POINT ( 'NONE',  ( 25.12854018303972126, 0.000000000000000000, 166.0317097002238995 ) ) ;
#7853=CARTESIAN_POINT ( 'NONE',  ( 30.64487238181199658, -6.928203230275514990, 160.2413957775779068 ) ) ;
#7860=VERTEX_POINT ( 'NONE', #25593 ) ;
#7865=CARTESIAN_POINT ( 'NONE',  ( 27.78090950529641745, 5.407089921784856479, 163.3246141667165716 ) ) ;
#7871=VECTOR ( 'NONE', #7944, 1000.000000000000000 ) ;
#7873=CARTESIAN_POINT ( 'NONE',  ( 24.00000000000000000, -5.196152422706629359, -4.743749998770946164 ) ) ;
#7874=CARTESIAN_POINT ( 'NONE',  ( 26.75643035624999655, -3.323476615752267271, -2.203124999385475569 ) ) ;
#7878=ADVANCED_FACE ( 'NONE', ( #19378 ), #5128, .F. ) ;
#7882=VECTOR ( 'NONE', #31668, 1000.000000000000114 ) ;
#7883=CARTESIAN_POINT ( 'NONE',  ( 30.96843807686976291, -6.928203230275506996, 163.9397685954678536 ) ) ;
#7889=CARTESIAN_POINT ( 'NONE',  ( 15.24356964375000167, -3.323476615752272600, -1.115624999385467442 ) ) ;
#7893=EDGE_LOOP ( 'NONE', ( #8702, #29721, #25430, #8762 ) ) ;
#7897=CARTESIAN_POINT ( 'NONE',  ( 15.02283181144952628, 7.347880794884122694E-16, 50.52293445648592751 ) ) ;
#7898=CARTESIAN_POINT ( 'NONE',  ( 31.07874456373121319, 7.209453229046482114, 165.2005775096280615 ) ) ;
#7900=( BOUNDED_CURVE ( )  B_SPLINE_CURVE ( 2, ( #565, #14802, #26916, #20680, #35064, #8921, #35249 ),
 .UNSPECIFIED., .F., .F. ) 
 B_SPLINE_CURVE_WITH_KNOTS ( ( 3, 2, 2, 3 ),
 ( 0.4130434782608697342, 0.4202898550724640248, 0.4275362318840583153, 0.4347826086956526059 ),
 .UNSPECIFIED. ) 
 CURVE ( )  GEOMETRIC_REPRESENTATION_ITEM ( )  RATIONAL_B_SPLINE_CURVE ( ( 0.9999999999999968914, 0.8660254037844418162, 1.000000000000000000, 0.8660254037844387076, 1.000000000000000000, 0.8660254037844304920, 1.000000000000008216 ) ) 
 REPRESENTATION_ITEM ( '' )  );
#7904=CARTESIAN_POINT ( 'NONE',  ( 26.99999999999999645, 7.347880794884117764E-16, -3.374999999999989342 ) ) ;
#7909=CARTESIAN_POINT ( 'NONE',  ( 21.00000000000000355, 0.000000000000000000, 50.00000000000001421 ) ) ;
#7912=VERTEX_POINT ( 'NONE', #8175 ) ;
#7913=CARTESIAN_POINT ( 'NONE',  ( 23.99999999999999645, 5.196152422706631135, -2.849999999999991651 ) ) ;
#7914=CARTESIAN_POINT ( 'NONE',  ( 25.83310289917887559, -3.320084631957848309, -8.000000000000000000 ) ) ;
#7916=CARTESIAN_POINT ( 'NONE',  ( 33.75396078491245078, 5.407089921784862696, 159.9599749780466027 ) ) ;
#7918=CARTESIAN_POINT ( 'NONE',  ( 33.59750473220383071, -5.196152422706635576, 159.5689982363720674 ) ) ;
#7924=VERTEX_POINT ( 'NONE', #19189 ) ;
#7928=CARTESIAN_POINT ( 'NONE',  ( 26.75643035624999655, 7.049594010296217766E-16, -9.928124999385474325 ) ) ;
#7940=CARTESIAN_POINT ( 'NONE',  ( 36.89818384675449892, -3.604726614523235284, 160.0801451655713663 ) ) ;
#7941=CARTESIAN_POINT ( 'NONE',  ( 34.16946429409239983, 5.196152422706631135, 166.1065259438235557 ) ) ;
#7944=DIRECTION ( 'NONE',  ( 0.000000000000000000, 0.000000000000000000, 1.000000000000000000 ) ) ;
#7949=FACE_OUTER_BOUND ( 'NONE', #5096, .T. ) ;
#7951=ORIENTED_EDGE ( 'NONE', *, *, #20756, .F. ) ;
#7952=CARTESIAN_POINT ( 'NONE',  ( 30.98559686366964883, -7.209453229046475009, 164.1358944260424835 ) ) ;
#7953=CARTESIAN_POINT ( 'NONE',  ( 18.12178482187500350, -4.985214923628407568, -5.915624999385471483 ) ) ;
#7955=CARTESIAN_POINT ( 'NONE',  ( 28.16820783713129472, 5.407089921784862696, 167.7514543563617622 ) ) ;
#7956=CARTESIAN_POINT ( 'NONE',  ( 37.41951561650348168, 3.464101615137759271, 168.8336428086314527 ) ) ;
#7964=ORIENTED_EDGE ( 'NONE', *, *, #25867, .T. ) ;
#7967=CARTESIAN_POINT ( 'NONE',  ( 18.12178482187499640, 4.985214923628404904, -5.165624999385470595 ) ) ;
#7970=CARTESIAN_POINT ( 'NONE',  ( 15.24356964374999990, 3.323476615752268604, -2.990624999385476102 ) ) ;
#7983=EDGE_CURVE ( 'NONE', #15182, #21163, #23391, .T. ) ;
#7991=ORIENTED_EDGE ( 'NONE', *, *, #23485, .T. ) ;
#7997=CARTESIAN_POINT ( 'NONE',  ( 20.99999999999999645, 0.000000000000000000, -8.000000000000000000 ) ) ;
#8002=CARTESIAN_POINT ( 'NONE',  ( 18.00000000000000355, -5.196152422706632912, -8.475000000000010303 ) ) ;
#8007=CARTESIAN_POINT ( 'NONE',  ( 15.24356964374999990, 0.000000000000000000, -6.553124999385484983 ) ) ;
#8012=EDGE_CURVE ( 'NONE', #29322, #6148, #10771, .T. ) ;
#8013=CARTESIAN_POINT ( 'NONE',  ( 37.56002276824448671, -3.604726614523238837, 167.6449986542055797 ) ) ;
#8048=EDGE_CURVE ( 'NONE', #31903, #16958, #26041, .T. ) ;
#8051=CARTESIAN_POINT ( 'NONE',  ( 37.02238078016989675, 3.604726614523238837, 161.4997226103520802 ) ) ;
#8052=CARTESIAN_POINT ( 'NONE',  ( 36.90311784072428480, -3.464101615137388013, 162.9311892224378369 ) ) ;
#8055=VERTEX_POINT ( 'NONE', #3214 ) ;
#8058=CARTESIAN_POINT ( 'NONE',  ( 15.00000000000000000, 0.000000000000000000, -3.993749998770945719 ) ) ;
#8059=CARTESIAN_POINT ( 'NONE',  ( 26.75643035624999655, 7.049594010296217766E-16, -1.715624999385462202 ) ) ;
#8070=CARTESIAN_POINT ( 'NONE',  ( 36.99463137071579411, 7.347880794884117764E-16, 163.9771936566585566 ) ) ;
#8075=CARTESIAN_POINT ( 'NONE',  ( 20.99999999999999645, -6.646953231504538984, -1.940624999385496929 ) ) ;
#8079=EDGE_LOOP ( 'NONE', ( #18501, #24789, #750, #15110 ) ) ;
#8080=DIRECTION ( 'NONE',  ( 0.08715574274765150453, 0.000000000000000000, 0.9961946980917461003 ) ) ;
#8083=CARTESIAN_POINT ( 'NONE',  ( 25.13507686385270290, 3.464101615137630485, 166.1064243038051416 ) ) ;
#8085=CARTESIAN_POINT ( 'NONE',  ( 24.55497793462844669, 0.000000000000000000, 162.2705114497308045 ) ) ;
#8101=CARTESIAN_POINT ( 'NONE',  ( 21.00000000000000000, 6.928203230275506996, -3.712500000000020339 ) ) ;
#8102=CARTESIAN_POINT ( 'NONE',  ( 26.60793733450167053, 1.299049382686714882, -8.000000000000000000 ) ) ;
#8103=CARTESIAN_POINT ( 'NONE',  ( 36.93576976081443775, 7.646167579472024665E-16, 160.5097541291234506 ) ) ;
#8105=CARTESIAN_POINT ( 'NONE',  ( 25.15145004905768644, -3.604726614523240613, 169.0882189147961583 ) ) ;
#8108=AXIS2_PLACEMENT_3D ( 'NONE', #5196, #1795, #28317 ) ;
#8112=ORIENTED_EDGE ( 'NONE', *, *, #32567, .F. ) ;
#8117=CARTESIAN_POINT ( 'NONE',  ( 21.00000000000000000, 6.646953231504538984, -8.465624999385484628 ) ) ;
#8122=CARTESIAN_POINT ( 'NONE',  ( 24.63341810310133084, 0.000000000000000000, 163.1670866780133906 ) ) ;
#8133=CARTESIAN_POINT ( 'NONE',  ( 37.05833252405330569, 7.646167579472015790E-16, 161.9106529233149274 ) ) ;
#8144=CARTESIAN_POINT ( 'NONE',  ( 24.55988044515800439, 0.000000000000000000, 162.3265474014984591 ) ) ;
#8145=CARTESIAN_POINT ( 'NONE',  ( 15.24356964374999990, 0.000000000000000000, -6.440624999385469174 ) ) ;
#8147=CARTESIAN_POINT ( 'NONE',  ( 37.56329110859752518, 7.646167579472024665E-16, 167.6823559553839971 ) ) ;
#8148=CARTESIAN_POINT ( 'NONE',  ( 28.20210112649392542, -5.196152422706638241, 166.7415323026203851 ) ) ;
#8159=CARTESIAN_POINT ( 'NONE',  ( 15.24356964374999990, 0.000000000000000000, -2.840624999385477079 ) ) ;
#8162=CARTESIAN_POINT ( 'NONE',  ( 18.12178482187499640, 4.985214923628404904, -1.228124999385488136 ) ) ;
#8175=CARTESIAN_POINT ( 'NONE',  ( 36.60243052835136268, 7.347880794884117764E-16, 159.4943175152456831 ) ) ;
#8187=CARTESIAN_POINT ( 'NONE',  ( 36.67106567565804198, 7.347880794884125653E-16, 160.2788208387686097 ) ) ;
#8189=CARTESIAN_POINT ( 'NONE',  ( 30.99785313993998059, -6.928203230275514990, 164.2759843048494588 ) ) ;
#8190=DIRECTION ( 'NONE',  ( 0.9961946980917462113, 0.000000000000000000, -0.08715574274765118534 ) ) ;
#8192=CARTESIAN_POINT ( 'NONE',  ( 19.95811783012620566, 5.908847734042487865, -9.999476472876560607 ) ) ;
#8197=CARTESIAN_POINT ( 'NONE',  ( 18.12178482187499640, 4.985214923628404904, -7.078124999385481786 ) ) ;
#8199=VERTEX_POINT ( 'NONE', #22765 ) ;
#8205=CARTESIAN_POINT ( 'NONE',  ( 30.67428744509644289, 6.928203230275506996, 160.5776114894081559 ) ) ;
#8212=LINE ( 'NONE', #31324, #18573 ) ;
#8213=CARTESIAN_POINT ( 'NONE',  ( 37.26263527955736521, 3.464101615137958667, 167.0404923520663090 ) ) ;
#8226=CARTESIAN_POINT ( 'NONE',  ( 27.91448717542667168, 5.196152422706636465, 163.4540897989176642 ) ) ;
#8235=DIRECTION ( 'NONE',  ( 0.9961946980917462113, 0.000000000000000000, -0.08715574274765118534 ) ) ;
#8240=CARTESIAN_POINT ( 'NONE',  ( 27.67632261399923976, -5.407089921784859143, 162.1291805290064474 ) ) ;
#8241=CARTESIAN_POINT ( 'NONE',  ( 26.99999999999999645, 7.347880794884117764E-16, -2.024999999999999023 ) ) ;
#8246=CARTESIAN_POINT ( 'NONE',  ( 18.00000000000000355, -5.196152422706632912, -5.268749998770943854 ) ) ;
#8247=CARTESIAN_POINT ( 'NONE',  ( 26.75643035624999655, 7.049594010296217766E-16, -3.515624999385458249 ) ) ;
#8256=CARTESIAN_POINT ( 'NONE',  ( 25.13834520420595098, 0.000000000000000000, 166.1437816049835874 ) ) ;
#8261=CARTESIAN_POINT ( 'NONE',  ( 18.12178482187500350, -4.985214923628407568, -4.678124999385496530 ) ) ;
#8269=CARTESIAN_POINT ( 'NONE',  ( 37.05669835387680422, 3.604726614523243278, 161.8919742727257187 ) ) ;
#8271=VECTOR ( 'NONE', #11231, 1000.000000000000000 ) ;
#8274=FACE_OUTER_BOUND ( 'NONE', #335, .T. ) ;
#8284=CARTESIAN_POINT ( 'NONE',  ( 18.00000000000000000, 5.196152422706630247, -3.675000000000011369 ) ) ;
#8285=CARTESIAN_POINT ( 'NONE',  ( 34.15639093268026016, -5.196152422706629359, 165.9570967391097440 ) ) ;
#8286=CARTESIAN_POINT ( 'NONE',  ( 36.93250142046139928, -3.604726614523238837, 160.4723968279449480 ) ) ;
#8288=CARTESIAN_POINT ( 'NONE',  ( 27.65301994718372569, -5.196152422706638241, 160.4655057046423678 ) ) ;
#8294=ORIENTED_EDGE ( 'NONE', *, *, #3854, .T. ) ;
#8296=CARTESIAN_POINT ( 'NONE',  ( 15.00000000000000000, 0.000000000000000000, -4.893749998770957177 ) ) ;
#8298=CARTESIAN_POINT ( 'NONE',  ( 15.24356964374999990, 3.323476615752268604, -8.390624999385488891 ) ) ;
#8302=VECTOR ( 'NONE', #308, 1000.000000000000000 ) ;
#8304=CARTESIAN_POINT ( 'NONE',  ( 27.63220001923324176, -5.407089921784865361, 161.6248569630975283 ) ) ;
#8306=CARTESIAN_POINT ( 'NONE',  ( 37.06653485837505713, 3.464101615138019508, 164.7990542813599006 ) ) ;
#8307=( BOUNDED_CURVE ( )  B_SPLINE_CURVE ( 2, ( #9977, #3542, #21183, #18721, #21370, #32909, #24573 ),
 .UNSPECIFIED., .F., .F. ) 
 B_SPLINE_CURVE_WITH_KNOTS ( ( 3, 2, 2, 3 ),
 ( 0.7391304347826077592, 0.7463768115942017722, 0.7536231884057958963, 0.7608695652173899093 ),
 .UNSPECIFIED. ) 
 CURVE ( )  GEOMETRIC_REPRESENTATION_ITEM ( )  RATIONAL_B_SPLINE_CURVE ( ( 1.000000000000016431, 0.8660254037844222763, 1.000000000000000000, 0.8660254037844387076, 1.000000000000000000, 0.8660254037844653530, 0.9999999999999733546 ) ) 
 REPRESENTATION_ITEM ( '' )  );
#8315=CARTESIAN_POINT ( 'NONE',  ( 37.02404643378602600, 7.347880794884125653E-16, 164.3134093660401618 ) ) ;
#8316=CARTESIAN_POINT ( 'NONE',  ( 34.49914238540488043, 5.407089921784862696, 168.4774396467310282 ) ) ;
#8320=CYLINDRICAL_SURFACE ( 'NONE', #24338, 6.000000000000001776 ) ;
#8327=CARTESIAN_POINT ( 'NONE',  ( 36.97662401522738662, -3.604726614523235284, 160.9767203938538955 ) ) ;
#8328=CARTESIAN_POINT ( 'NONE',  ( 26.75643035624999655, 7.049594010296217766E-16, -8.015624999385462246 ) ) ;
#8329=VECTOR ( 'NONE', #20193, 1000.000000000000000 ) ;
#8331=CARTESIAN_POINT ( 'NONE',  ( 34.34226204845910502, 5.407089921784862696, 166.6842891901658845 ) ) ;
#8332=CARTESIAN_POINT ( 'NONE',  ( 37.21687851461520324, -3.464101615137755275, 166.5174901355681527 ) ) ;
#8338=EDGE_LOOP ( 'NONE', ( #34435, #30896, #849, #29628 ) ) ;
#8344=CARTESIAN_POINT ( 'NONE',  ( 15.24356964374999990, 0.000000000000000000, -2.503124999385486493 ) ) ;
#8355=EDGE_CURVE ( 'NONE', #14365, #16958, #6929, .T. ) ;
#8357=CYLINDRICAL_SURFACE ( 'NONE', #36095, 5.999999999999994671 ) ;
#8365=CARTESIAN_POINT ( 'NONE',  ( 14.99999999999992184, 3.464101615137706425, -4.481249998770945098 ) ) ;
#8369=CARTESIAN_POINT ( 'NONE',  ( 18.12178482187499640, 4.985214923628404904, -0.6656249993854668201 ) ) ;
#8373=CARTESIAN_POINT ( 'NONE',  ( 36.95541128647934670, 7.347880794884117764E-16, 163.5289060425172636 ) ) ;
#8381=CARTESIAN_POINT ( 'NONE',  ( 21.00000000000000000, 6.646953231504538984, -8.915624999385478588 ) ) ;
#8383=ORIENTED_EDGE ( 'NONE', *, *, #24319, .T. ) ;
#8388=CARTESIAN_POINT ( 'NONE',  ( 28.01132750018552287, 5.407089921784862696, 165.9583038997966185 ) ) ;
#8390=CARTESIAN_POINT ( 'NONE',  ( 24.70692427760507570, 0.000000000000000000, 161.2126178494294493 ) ) ;
#8394=CARTESIAN_POINT ( 'NONE',  ( 37.61068204371655099, 3.604726614523238837, 168.2240368224713620 ) ) ;
#8398=CARTESIAN_POINT ( 'NONE',  ( 37.25936693920468201, 7.347880794884125653E-16, 167.0031350508878631 ) ) ;
#8410=CARTESIAN_POINT ( 'NONE',  ( 27.00000000000063238, 3.464101615137388013, -5.531249998770964460 ) ) ;
#8421=CARTESIAN_POINT ( 'NONE',  ( 27.70246933682352974, 5.407089921784856479, 162.4280389384339855 ) ) ;
#8422=CARTESIAN_POINT ( 'NONE',  ( 15.24356964374999990, 3.323476615752268604, -1.190624999385493377 ) ) ;
#8427=VERTEX_POINT ( 'NONE', #13783 ) ;
#8428=CARTESIAN_POINT ( 'NONE',  ( 21.00000000000000000, 6.928203230275506996, -6.806249998770949716 ) ) ;
#8429=CARTESIAN_POINT ( 'NONE',  ( 18.12178482187500350, -4.985214923628407568, -1.865624999385473437 ) ) ;
#8431=CARTESIAN_POINT ( 'NONE',  ( 15.24356964374999990, 0.000000000000000000, -10.04062499938546082 ) ) ;
#8436=CARTESIAN_POINT ( 'NONE',  ( 27.97658564224149558, -5.196152422706632912, 164.1638785225323431 ) ) ;
#8441=CARTESIAN_POINT ( 'NONE',  ( 23.87821517812500005, -4.985214923628404016, -4.153124999385471305 ) ) ;
#8451=CARTESIAN_POINT ( 'NONE',  ( 27.67142010346968561, -5.407089921784865361, 162.0731445772388213 ) ) ;
#8462=ORIENTED_EDGE ( 'NONE', *, *, #35322, .F. ) ;
#8463=CARTESIAN_POINT ( 'NONE',  ( 26.99999999999999645, -3.464101615137751278, -4.312500000000005329 ) ) ;
#8465=CARTESIAN_POINT ( 'NONE',  ( 33.78010750773675852, -5.407089921784861808, 160.2588333874741124 ) ) ;
#8467=CARTESIAN_POINT ( 'NONE',  ( 31.31896757967941625, 7.209453229046475009, 167.9463391462434174 ) ) ;
#8469=FACE_OUTER_BOUND ( 'NONE', #34614, .T. ) ;
#8471=ORIENTED_EDGE ( 'NONE', *, *, #22948, .F. ) ;
#8473=DIRECTION ( 'NONE',  ( 0.08715574274765150453, 0.000000000000000000, 0.9961946980917461003 ) ) ;
#8476=AXIS2_PLACEMENT_3D ( 'NONE', #26202, #26019, #17315 ) ;
#8479=CARTESIAN_POINT ( 'NONE',  ( 15.24356964374999990, 0.000000000000000000, -9.253124999385493155 ) ) ;
#8483=CARTESIAN_POINT ( 'NONE',  ( 30.72576380560321851, 7.209453229046482114, 161.1659889823564811 ) ) ;
#8492=EDGE_CURVE ( 'NONE', #805, #407, #14210, .T. ) ;
#8493=ORIENTED_EDGE ( 'NONE', *, *, #27064, .F. ) ;
#8497=CARTESIAN_POINT ( 'NONE',  ( 30.59339602130522096, -7.209453229046475009, 159.6530182846296384 ) ) ;
#8498=CARTESIAN_POINT ( 'NONE',  ( 18.00000000000000355, -5.196152422706632912, -3.468749998770948029 ) ) ;
#8509=CARTESIAN_POINT ( 'NONE',  ( 37.06160086440634416, 3.604726614523238837, 161.9480102244933732 ) ) ;
#8510=CARTESIAN_POINT ( 'NONE',  ( 26.75643035624999655, 3.323476615752271712, -7.978124999385458160 ) ) ;
#8512=CARTESIAN_POINT ( 'NONE',  ( 37.48158259977161322, -3.604726614523238837, 166.7484234259230220 ) ) ;
#8513=CARTESIAN_POINT ( 'NONE',  ( 37.10575494261194507, 3.464101615137759271, 165.2473418955011937 ) ) ;
#8520=ORIENTED_EDGE ( 'NONE', *, *, #36496, .T. ) ;
#8527=CARTESIAN_POINT ( 'NONE',  ( 15.24356964374999990, 3.323476615752268604, -2.540624999385480809 ) ) ;
#8537=VECTOR ( 'NONE', #8473, 1000.000000000000000 ) ;
#8546=CARTESIAN_POINT ( 'NONE',  ( 28.30384396178233075, -5.407089921784859143, 169.3017823552670507 ) ) ;
#8548=CARTESIAN_POINT ( 'NONE',  ( 26.75643035624999655, -3.323476615752267715, -0.4031249993854607028 ) ) ;
#8562=CARTESIAN_POINT ( 'NONE',  ( 21.00000000000000000, -6.646953231504538984, -8.240624999385500971 ) ) ;
#8568=CARTESIAN_POINT ( 'NONE',  ( 31.09835460584942624, -7.209453229046482114, 165.4247213166987081 ) ) ;
#8574=CARTESIAN_POINT ( 'NONE',  ( 25.18413345258806046, 3.604726614523236616, 169.4617919265805881 ) ) ;
#8577=CARTESIAN_POINT ( 'NONE',  ( 15.00000000000000000, 0.000000000000000000, -7.200000000000011724 ) ) ;
#8583=ORIENTED_EDGE ( 'NONE', *, *, #8896, .F. ) ;
#8587=CARTESIAN_POINT ( 'NONE',  ( 31.28219875076131018, -6.928203230275506996, 167.5260695085981411 ) ) ;
#8596=CARTESIAN_POINT ( 'NONE',  ( 28.15961270201155742, 5.196152422706630247, 166.2558873885250250 ) ) ;
#8601=CARTESIAN_POINT ( 'NONE',  ( 24.60236886974748316, -3.604726614523240613, 162.8121923168181695 ) ) ;
#8603=CARTESIAN_POINT ( 'NONE',  ( 15.24356964374999990, 3.323476615752268604, -2.990624999385476102 ) ) ;
#8608=EDGE_LOOP ( 'NONE', ( #3986, #5370, #2864, #5429 ) ) ;
#8609=CARTESIAN_POINT ( 'NONE',  ( 15.00000000000000000, 0.000000000000000000, -6.693749998770953447 ) ) ;
#8610=CARTESIAN_POINT ( 'NONE',  ( 23.87821517812499650, 4.985214923628404904, -2.090624999385476634 ) ) ;
#8619=CARTESIAN_POINT ( 'NONE',  ( 36.87697111800645899, 7.347880794884117764E-16, 162.6323308142347059 ) ) ;
#8623=( BOUNDED_CURVE ( )  B_SPLINE_CURVE ( 2, ( #3150, #31226, #11133, #16831, #17200, #28373, #22711 ),
 .UNSPECIFIED., .F., .F. ) 
 B_SPLINE_CURVE_WITH_KNOTS ( ( 3, 2, 2, 3 ),
 ( 0.7391304347826076482, 0.7463768115942017722, 0.7536231884057957853, 0.7608695652173899093 ),
 .UNSPECIFIED. ) 
 CURVE ( )  GEOMETRIC_REPRESENTATION_ITEM ( )  RATIONAL_B_SPLINE_CURVE ( ( 1.000000000000018430, 0.8660254037844202779, 1.000000000000000000, 0.8660254037844387076, 1.000000000000000000, 0.8660254037844653530, 0.9999999999999733546 ) ) 
 REPRESENTATION_ITEM ( '' )  );
#8624=CARTESIAN_POINT ( 'NONE',  ( 18.12178482187500350, -4.985214923628407568, -5.128124999385475391 ) ) ;
#8633=FACE_OUTER_BOUND ( 'NONE', #3706, .T. ) ;
#8634=CARTESIAN_POINT ( 'NONE',  ( 37.05016167317072728, -3.604726614523238837, 161.8172596703688555 ) ) ;
#8637=DIRECTION ( 'NONE',  ( 1.000000000000000000, 0.000000000000000000, 0.000000000000000000 ) ) ;
#8646=CARTESIAN_POINT ( 'NONE',  ( 23.99999999999999645, 5.196152422706631135, -5.099999999999993427 ) ) ;
#8649=CARTESIAN_POINT ( 'NONE',  ( 36.93903810116746911, 3.604726614523243278, 160.5471114303018680 ) ) ;
#8651=CARTESIAN_POINT ( 'NONE',  ( 25.19067013329413385, -3.604726614523240613, 169.5365065289374797 ) ) ;
#8653=CYLINDRICAL_SURFACE ( 'NONE', #36033, 6.000000000000001776 ) ;
#8656=ORIENTED_EDGE ( 'NONE', *, *, #11802, .T. ) ;
#8657=CARTESIAN_POINT ( 'NONE',  ( 27.62360488411350801, -5.196152422706632912, 160.1292899952607627 ) ) ;
#8662=CARTESIAN_POINT ( 'NONE',  ( 14.99999999999952394, -3.464101615137481716, -5.306249998770948828 ) ) ;
#8667=CARTESIAN_POINT ( 'NONE',  ( 28.36878648460592700, -5.196152422706632912, 168.6467546639452166 ) ) ;
#8670=SHAPE_DEFINITION_REPRESENTATION ( #32253, #29986 ) ;
#8675=VERTEX_POINT ( 'NONE', #21888 ) ;
#8680=CARTESIAN_POINT ( 'NONE',  ( 25.17923094205850276, 3.604726614523240613, 169.4057559748129336 ) ) ;
#8681=CARTESIAN_POINT ( 'NONE',  ( 26.99999999999999645, 3.464101615137755275, -2.831249998770950072 ) ) ;
#8684=FACE_OUTER_BOUND ( 'NONE', #16949, .T. ) ;
#8687=CARTESIAN_POINT ( 'NONE',  ( 15.02283181144952628, 7.347880794884122694E-16, 50.52293445648592751 ) ) ;
#8690=CARTESIAN_POINT ( 'NONE',  ( 37.10082094864278446, 3.604726614523238837, 162.3962978386346663 ) ) ;
#8691=CARTESIAN_POINT ( 'NONE',  ( 21.00000000000000000, -6.646953231504538984, -7.678124999385482319 ) ) ;
#8693=CARTESIAN_POINT ( 'NONE',  ( 25.10405911393864642, 0.000000000000000000, 168.5465380477087933 ) ) ;
#8694=CARTESIAN_POINT ( 'NONE',  ( 31.23317364535864371, -6.928203230275514990, 166.9657099896971602 ) ) ;
#8699=AXIS2_PLACEMENT_3D ( 'NONE', #25646, #11611, #23369 ) ;
#8701=ORIENTED_EDGE ( 'NONE', *, *, #35342, .T. ) ;
#8702=ORIENTED_EDGE ( 'NONE', *, *, #23541, .F. ) ;
#8708=CARTESIAN_POINT ( 'NONE',  ( 23.87821517812499650, 4.985214923628404904, -4.903124999385472194 ) ) ;
#8709=VECTOR ( 'NONE', #16765, 1000.000000000000000 ) ;
#8717=CARTESIAN_POINT ( 'NONE',  ( 21.00000000000016342, 4.000000000000002665, 50.00000000000000000 ) ) ;
#8722=CARTESIAN_POINT ( 'NONE',  ( 36.94887460566563675, 3.464101615138066137, 163.4541914389360784 ) ) ;
#8732=VECTOR ( 'NONE', #31338, 1000.000000000000000 ) ;
#8735=CARTESIAN_POINT ( 'NONE',  ( 15.24356964374999990, 3.323476615752268604, -0.6281249993854746139 ) ) ;
#8744=VERTEX_POINT ( 'NONE', #1032 ) ;
#8745=ORIENTED_EDGE ( 'NONE', *, *, #33601, .T. ) ;
#8749=CARTESIAN_POINT ( 'NONE',  ( 15.24356964374999990, 0.000000000000000000, -9.703124999385471128 ) ) ;
#8754=CARTESIAN_POINT ( 'NONE',  ( 34.36840877128340566, -5.407089921784861808, 166.9831475995933943 ) ) ;
#8761=CARTESIAN_POINT ( 'NONE',  ( 28.21233043189729273, 5.407089921784856479, 168.2557779222707097 ) ) ;
#8762=ORIENTED_EDGE ( 'NONE', *, *, #10856, .F. ) ;
#8770=EDGE_CURVE ( 'NONE', #18510, #19175, #24829, .T. ) ;
#8784=ORIENTED_EDGE ( 'NONE', *, *, #5504, .T. ) ;
#8788=ORIENTED_EDGE ( 'NONE', *, *, #11802, .F. ) ;
#8791=CARTESIAN_POINT ( 'NONE',  ( 36.82301201863464968, 7.646167579472015790E-16, 159.2209272384671976 ) ) ;
#8792=CARTESIAN_POINT ( 'NONE',  ( 18.12178482187500350, -4.985214923628407568, -3.328124999385479121 ) ) ;
#8799=CARTESIAN_POINT ( 'NONE',  ( 26.75643035624999655, 7.049594010296217766E-16, -4.865624999385476102 ) ) ;
#8807=CARTESIAN_POINT ( 'NONE',  ( 33.72497000607938844, -5.196152422706629359, 161.0259329835556059 ) ) ;
#8811=CARTESIAN_POINT ( 'NONE',  ( 18.12178482187500350, -4.985214923628407568, -3.778124999385484628 ) ) ;
#8819=CYLINDRICAL_SURFACE ( 'NONE', #21099, 5.999999999999994671 ) ;
#8820=CARTESIAN_POINT ( 'NONE',  ( 33.89776776044609363, -5.407089921784861808, 161.6036962298979915 ) ) ;
#8824=( BOUNDED_CURVE ( )  B_SPLINE_CURVE ( 2, ( #1871, #33715, #25186, #36739, #10778, #2801, #5831 ),
 .UNSPECIFIED., .F., .F. ) 
 B_SPLINE_CURVE_WITH_KNOTS ( ( 3, 2, 2, 3 ),
 ( 0.9347826086956505520, 0.9420289855072447871, 0.9492753623188391332, 0.9565217391304334793 ),
 .UNSPECIFIED. ) 
 CURVE ( )  GEOMETRIC_REPRESENTATION_ITEM ( )  RATIONAL_B_SPLINE_CURVE ( ( 1.000000000000030864, 0.8660254037844079544, 1.000000000000000000, 0.8660254037844387076, 1.000000000000000000, 0.8660254037844633546, 0.9999999999999753530 ) ) 
 REPRESENTATION_ITEM ( '' )  );
#8834=CARTESIAN_POINT ( 'NONE',  ( 26.99999999999999645, 3.464101615137755275, -5.587499999999997691 ) ) ;
#8835=CARTESIAN_POINT ( 'NONE',  ( 25.20698035151260896, 0.000000000000000000, 166.9282849285064856 ) ) ;
#8838=CARTESIAN_POINT ( 'NONE',  ( 31.29935753756119965, -7.209453229046475009, 167.7221953391727709 ) ) ;
#8840=CARTESIAN_POINT ( 'NONE',  ( 20.99999999999999645, 6.928203230275506996, -0.9562499987709413007 ) ) ;
#8844=CYLINDRICAL_SURFACE ( 'NONE', #6085, 5.999999999999994671 ) ;
#8847=CARTESIAN_POINT ( 'NONE',  ( 15.24356964374999990, 3.323476615752268604, -7.378124999385474503 ) ) ;
#8853=CARTESIAN_POINT ( 'NONE',  ( 34.32634463103817524, 5.196152422706631135, 167.8996764003886994 ) ) ;
#8857=DIRECTION ( 'NONE',  ( 0.08715574274765150453, 0.000000000000000000, 0.9961946980917461003 ) ) ;
#8860=ORIENTED_EDGE ( 'NONE', *, *, #7007, .T. ) ;
#8864=CARTESIAN_POINT ( 'NONE',  ( 24.40626844856526745, -3.604726614523240613, 160.5707542461117612 ) ) ;
#8865=CARTESIAN_POINT ( 'NONE',  ( 15.00000000000000000, 0.000000000000000000, -1.293749998770965526 ) ) ;
#8872=CARTESIAN_POINT ( 'NONE',  ( 33.64979817785242489, 5.196152422706637353, 160.1667150552271437 ) ) ;
#8874=CARTESIAN_POINT ( 'NONE',  ( 37.09428426793671463, -3.604726614523235284, 162.3215832362777746 ) ) ;
#8875=CARTESIAN_POINT ( 'NONE',  ( 18.12178482187499640, 4.985214923628404904, -8.315624999385457627 ) ) ;
#8877=CARTESIAN_POINT ( 'NONE',  ( 24.78703009969406779, 3.604726614523240613, 164.9228798334000601 ) ) ;
#8878=CARTESIAN_POINT ( 'NONE',  ( 31.07629330841286830, -6.928203230275514990, 165.1725595331320449 ) ) ;
#8891=CARTESIAN_POINT ( 'NONE',  ( 26.75643035624999655, 3.323476615752271712, -4.940624999385510918 ) ) ;
#8896=EDGE_CURVE ( 'NONE', #16958, #3817, #32572, .T. ) ;
#8899=CARTESIAN_POINT ( 'NONE',  ( 27.89814547376861142, -5.196152422706632912, 163.2673032942497571 ) ) ;
#8905=CARTESIAN_POINT ( 'NONE',  ( 36.94560626531313829, 7.347880794884125653E-16, 163.4168341377576041 ) ) ;
#8908=EDGE_CURVE ( 'NONE', #13274, #7860, #18310, .T. ) ;
#8920=CYLINDRICAL_SURFACE ( 'NONE', #25333, 5.999999999999994671 ) ;
#8921=CARTESIAN_POINT ( 'NONE',  ( 14.99999999999979039, -3.464101615137634038, -4.856249998770949539 ) ) ;
#8926=CARTESIAN_POINT ( 'NONE',  ( 26.99999999999999645, 7.347880794884117764E-16, -5.118749998770960374 ) ) ;
#8927=ORIENTED_EDGE ( 'NONE', *, *, #10754, .F. ) ;
#8932=CARTESIAN_POINT ( 'NONE',  ( 23.87821517812500005, -4.985214923628404016, -9.103124999385482141 ) ) ;
#8940=CARTESIAN_POINT ( 'NONE',  ( 37.48485094012463748, 7.646167579472024665E-16, 166.7857807271014394 ) ) ;
#8946=CYLINDRICAL_SURFACE ( 'NONE', #26687, 6.000000000000001776 ) ;
#8959=ORIENTED_EDGE ( 'NONE', *, *, #18561, .F. ) ;
#8963=CARTESIAN_POINT ( 'NONE',  ( 26.99999999999999645, 7.347880794884117764E-16, -1.574999999999993072 ) ) ;
#8966=CARTESIAN_POINT ( 'NONE',  ( 34.31327126962603558, -5.196152422706629359, 167.7502471956748877 ) ) ;
#8969=CARTESIAN_POINT ( 'NONE',  ( 36.78872592836736288, 7.347880794884125653E-16, 161.6236836811924604 ) ) ;
#8970=VECTOR ( 'NONE', #21963, 1000.000000000000000 ) ;
#8971=VERTEX_POINT ( 'NONE', #36648 ) ;
#8977=CARTESIAN_POINT ( 'NONE',  ( 15.24356964375000167, -3.323476615752272600, -2.465624999385486404 ) ) ;
#8980=EDGE_LOOP ( 'NONE', ( #15418, #5660, #34133, #7428 ) ) ;
#8982=CARTESIAN_POINT ( 'NONE',  ( 20.99999999999999645, -6.646953231504538984, -5.428124999385471661 ) ) ;
#8988=DIRECTION ( 'NONE',  ( 0.08715574274765150453, 0.000000000000000000, 0.9961946980917461003 ) ) ;
#8992=CARTESIAN_POINT ( 'NONE',  ( 33.81648353596441581, 5.196152422706631135, 162.0719374165519469 ) ) ;
#8996=CARTESIAN_POINT ( 'NONE',  ( 26.75643035624999655, 7.049594010296217766E-16, -5.428124999385497418 ) ) ;
#9000=ORIENTED_EDGE ( 'NONE', *, *, #32582, .F. ) ;
#9004=FACE_OUTER_BOUND ( 'NONE', #5323, .T. ) ;
#9014=CARTESIAN_POINT ( 'NONE',  ( 26.99999999999946354, 3.464101615138061696, -7.781249998770928933 ) ) ;
#9018=CARTESIAN_POINT ( 'NONE',  ( 23.99999999999999645, 5.196152422706631135, -7.800000000000001599 ) ) ;
#9019=CYLINDRICAL_SURFACE ( 'NONE', #33031, 6.000000000000001776 ) ;
#9020=CARTESIAN_POINT ( 'NONE',  ( 18.00000000000000000, 5.196152422706630247, -6.768749998770945631 ) ) ;
#9022=CARTESIAN_POINT ( 'NONE',  ( 37.40804494182826545, -3.604726614523235284, 165.9078841494080336 ) ) ;
#9024=EDGE_CURVE ( 'NONE', #8744, #3817, #30977, .T. ) ;
#9033=CARTESIAN_POINT ( 'NONE',  ( 23.87821517812500005, -4.985214923628404016, -5.390624999385473792 ) ) ;
#9040=CARTESIAN_POINT ( 'NONE',  ( 30.60810355289388696, 7.209453229046482114, 159.8211261399325736 ) ) ;
#9050=( BOUNDED_CURVE ( )  B_SPLINE_CURVE ( 2, ( #34992, #15097, #26091, #23072, #12058, #8662, #29109 ),
 .UNSPECIFIED., .F., .F. ) 
 B_SPLINE_CURVE_WITH_KNOTS ( ( 3, 2, 2, 3 ),
 ( 0.4565217391304355332, 0.4637681159420298238, 0.4710144927536241144, 0.4782608695652184050 ),
 .UNSPECIFIED. ) 
 CURVE ( )  GEOMETRIC_REPRESENTATION_ITEM ( )  RATIONAL_B_SPLINE_CURVE ( ( 0.9999999999999856781, 0.8660254037844530295, 1.000000000000000000, 0.8660254037844387076, 1.000000000000000000, 0.8660254037844202779, 1.000000000000018430 ) ) 
 REPRESENTATION_ITEM ( '' )  );
#9052=CARTESIAN_POINT ( 'NONE',  ( 15.00000000000000178, -3.464101615137757051, -6.262500000000007283 ) ) ;
#9054=CARTESIAN_POINT ( 'NONE',  ( 34.52528910822917396, -5.407089921784861808, 168.7762980561585380 ) ) ;
#9055=CARTESIAN_POINT ( 'NONE',  ( 18.00000000000000355, -5.196152422706632912, -3.018749998770942078 ) ) ;
#9063=CARTESIAN_POINT ( 'NONE',  ( 28.00273236506578201, 5.196152422706630247, 164.4627369319599097 ) ) ;
#9066=CARTESIAN_POINT ( 'NONE',  ( 33.78501001826630556, -5.407089921784855591, 160.3148693392417670 ) ) ;
#9067=CARTESIAN_POINT ( 'NONE',  ( 18.12178482187500350, -4.985214923628407568, -8.615624999385479654 ) ) ;
#9069=CARTESIAN_POINT ( 'NONE',  ( 24.82625018393051164, 3.604726614523240613, 165.3711674475414100 ) ) ;
#9070=CARTESIAN_POINT ( 'NONE',  ( 34.04199902021685631, 5.196152422706637353, 164.6495911966399888 ) ) ;
#9074=( BOUNDED_CURVE ( )  B_SPLINE_CURVE ( 2, ( #2694, #14270, #37002, #31692, #31880, #8213, #8398 ),
 .UNSPECIFIED., .F., .F. ) 
 B_SPLINE_CURVE_WITH_KNOTS ( ( 3, 2, 2, 3 ),
 ( 0.1739130434782606427, 0.1811594202898546835, 0.1884057971014487243, 0.1956521739130427651 ),
 .UNSPECIFIED. ) 
 CURVE ( )  GEOMETRIC_REPRESENTATION_ITEM ( )  RATIONAL_B_SPLINE_CURVE ( ( 1.000000000000003997, 0.8660254037844345998, 1.000000000000000000, 0.8660254037844387076, 1.000000000000000000, 0.8660254037844520303, 0.9999999999999866773 ) ) 
 REPRESENTATION_ITEM ( '' )  );
#9078=EDGE_LOOP ( 'NONE', ( #29235, #5460, #30093, #8701 ) ) ;
#9082=CARTESIAN_POINT ( 'NONE',  ( 23.87821517812500005, -4.985214923628404016, -4.153124999385471305 ) ) ;
#9092=AXIS2_PLACEMENT_3D ( 'NONE', #23152, #37167, #8190 ) ;
#9097=CARTESIAN_POINT ( 'NONE',  ( 33.68901826208886519, 5.196152422706637353, 160.6150026693684367 ) ) ;
#9108=ORIENTED_EDGE ( 'NONE', *, *, #19180, .T. ) ;
#9109=CARTESIAN_POINT ( 'NONE',  ( 25.02725311564228150, 3.604726614523236616, 167.6686414700154444 ) ) ;
#9112=CARTESIAN_POINT ( 'NONE',  ( 15.24356964374999990, 0.000000000000000000, -1.490624999385459226 ) ) ;
#9119=DIRECTION ( 'NONE',  ( 0.000000000000000000, 0.000000000000000000, 1.000000000000000000 ) ) ;
#9123=CARTESIAN_POINT ( 'NONE',  ( 26.75643035624999655, -3.323476615752267715, -9.065624999385498484 ) ) ;
#9131=CARTESIAN_POINT ( 'NONE',  ( 37.36392234706227811, -3.604726614523238837, 165.4035605834991145 ) ) ;
#9139=CARTESIAN_POINT ( 'NONE',  ( 28.26462387754589045, -5.407089921784859143, 168.8534947411257576 ) ) ;
#9153=DIRECTION ( 'NONE',  ( 0.08715574274765150453, 0.000000000000000000, 0.9961946980917461003 ) ) ;
#9155=CARTESIAN_POINT ( 'NONE',  ( 37.39010055343310768, 3.464101615137841872, 168.4974270992498475 ) ) ;
#9165=CARTESIAN_POINT ( 'NONE',  ( 27.50636891564131759, 5.407089921784856479, 160.1866008677275772 ) ) ;
#9166=CARTESIAN_POINT ( 'NONE',  ( 23.87821517812499650, 4.985214923628404904, -2.203124999385491556 ) ) ;
#9170=ORIENTED_EDGE ( 'NONE', *, *, #4266, .T. ) ;
#9171=CARTESIAN_POINT ( 'NONE',  ( 20.99999999999999645, -6.646953231504538984, -4.078124999385484450 ) ) ;
#9172=CARTESIAN_POINT ( 'NONE',  ( 36.59262550718515428, 7.347880794884125653E-16, 159.3822456104860237 ) ) ;
#9179=CARTESIAN_POINT ( 'NONE',  ( 36.72009078106068358, 7.347880794884117764E-16, 160.8391803576695622 ) ) ;
#9183=EDGE_CURVE ( 'NONE', #28874, #15760, #17880, .T. ) ;
#9184=CARTESIAN_POINT ( 'NONE',  ( 18.12178482187500350, -4.985214923628407568, -7.378124999385477167 ) ) ;
#9193=DIRECTION ( 'NONE',  ( 1.000000000000000000, 0.000000000000000000, 0.000000000000000000 ) ) ;
#9206=CARTESIAN_POINT ( 'NONE',  ( 21.00000000000000000, 6.928203230275506996, -6.412499999999995204 ) ) ;
#9210=CARTESIAN_POINT ( 'NONE',  ( 34.42560472746153977, 5.407089921784857367, 167.6369003702161251 ) ) ;
#9216=CARTESIAN_POINT ( 'NONE',  ( 24.62848410913218800, 0.000000000000000000, 160.3160426211468348 ) ) ;
#9217=CARTESIAN_POINT ( 'NONE',  ( 30.57623723450533504, -6.928203230275506996, 159.4568924540549517 ) ) ;
#9219=CARTESIAN_POINT ( 'NONE',  ( 26.75643035624999655, -3.323476615752267715, -5.353124999385477700 ) ) ;
#9225=CARTESIAN_POINT ( 'NONE',  ( 30.62771359501211066, -7.209453229046482114, 160.0452699470032485 ) ) ;
#9240=CARTESIAN_POINT ( 'NONE',  ( 20.16825598028117028, 5.708404836608378830, -8.000000000000001776 ) ) ;
#9241=CARTESIAN_POINT ( 'NONE',  ( 28.08976766865841057, 5.407089921784862696, 166.8548791280792045 ) ) ;
#9242=CARTESIAN_POINT ( 'NONE',  ( 26.99999999999999645, 7.347880794884117764E-16, -2.868749998770958598 ) ) ;
#9243=EDGE_CURVE ( 'NONE', #10376, #17383, #22569, .T. ) ;
#9246=CARTESIAN_POINT ( 'NONE',  ( 26.99999999999999289, 0.000000000000000000, -8.000000000000000000 ) ) ;
#9253=CARTESIAN_POINT ( 'NONE',  ( 28.41593846164884241, 5.957544813848093312, 159.6438083957854133 ) ) ;
#9254=CARTESIAN_POINT ( 'NONE',  ( 15.24356964375000167, -3.323476615752272600, -9.553124999385460114 ) ) ;
#9255=CARTESIAN_POINT ( 'NONE',  ( 37.34761212884377812, 7.347880794884117764E-16, 168.0117821839301087 ) ) ;
#9256=CARTESIAN_POINT ( 'NONE',  ( 27.97210741594907901, 5.407089921784862696, 165.5100162856553538 ) ) ;
#9257=PRODUCT_DEFINITION_CONTEXT ( 'detailed design', #23111, 'design' ) ;
#9258=CARTESIAN_POINT ( 'NONE',  ( 24.97165984609394940, 0.000000000000000000, 164.2385592436587558 ) ) ;
#9259=CARTESIAN_POINT ( 'NONE',  ( 25.16776026727616511, 0.000000000000000000, 166.4799973143651926 ) ) ;
#9265=ORIENTED_EDGE ( 'NONE', *, *, #1898, .F. ) ;
#9267=CARTESIAN_POINT ( 'NONE',  ( 36.91619120224290640, 7.347880794884117764E-16, 163.0806184283759706 ) ) ;
#9270=CARTESIAN_POINT ( 'NONE',  ( 21.00000000000000000, 6.646953231504538984, -3.065624999385470062 ) ) ;
#9280=CARTESIAN_POINT ( 'NONE',  ( 24.00000000000000000, -5.196152422706629359, -3.000000000000002665 ) ) ;
#9285=CARTESIAN_POINT ( 'NONE',  ( 37.25443294523552851, 7.646167579472015790E-16, 164.1520909940213642 ) ) ;
#9290=CARTESIAN_POINT ( 'NONE',  ( 26.99999999999999645, 7.347880794884117764E-16, -5.568749998770966769 ) ) ;
#9295=CIRCLE ( 'NONE', #36436, 5.999999999999994671 ) ;
#9299=CARTESIAN_POINT ( 'NONE',  ( 31.14247720061542068, -7.209453229046475009, 165.9290448826076272 ) ) ;
#9300=CARTESIAN_POINT ( 'NONE',  ( 15.24356964374999990, 3.323476615752268604, -1.978124999385461935 ) ) ;
#9304=LINE ( 'NONE', #26917, #2896 ) ;
#9312=CARTESIAN_POINT ( 'NONE',  ( 21.00000000000000000, -6.646953231504538984, -0.4781249993854547187 ) ) ;
#9314=CARTESIAN_POINT ( 'NONE',  ( 18.00000000000000355, -5.196152422706632912, -6.168749998770955756 ) ) ;
#9319=CARTESIAN_POINT ( 'NONE',  ( 24.67263818733777470, 0.000000000000000000, 163.6153742921546836 ) ) ;
#9326=CARTESIAN_POINT ( 'NONE',  ( 24.87037277869651319, 3.604726614523236616, 165.8754910134502722 ) ) ;
#9346=CARTESIAN_POINT ( 'NONE',  ( 33.64652983760650073, -5.196152422706629359, 160.1293577552730483 ) ) ;
#9355=CARTESIAN_POINT ( 'NONE',  ( 23.87821517812500005, -4.985214923628404016, -5.503124999385489602 ) ) ;
#9360=CARTESIAN_POINT ( 'NONE',  ( 20.99999999999999645, -6.646953231504538984, -4.978124999385475036 ) ) ;
#9368=CARTESIAN_POINT ( 'NONE',  ( 36.80179928988660976, 3.464101615137755275, 161.7731128871305657 ) ) ;
#9373=CARTESIAN_POINT ( 'NONE',  ( 15.24356964375000167, -3.323476615752272600, -7.865624999385466332 ) ) ;
#9381=CARTESIAN_POINT ( 'NONE',  ( 27.50146640511176344, 5.407089921784862696, 160.1305649159599227 ) ) ;
#9383=CARTESIAN_POINT ( 'NONE',  ( 37.03385145495223441, 7.347880794884117764E-16, 164.4254812707998497 ) ) ;
#9386=VECTOR ( 'NONE', #3463, 1000.000000000000000 ) ;
#9389=CARTESIAN_POINT ( 'NONE',  ( 31.37044394018620252, 6.928203230275514990, 168.5347166391916574 ) ) ;
#9395=CARTESIAN_POINT ( 'NONE',  ( 21.00000000000000000, 6.928203230275506996, -5.962499999999998579 ) ) ;
#9399=CARTESIAN_POINT ( 'NONE',  ( 24.90959286293295349, 3.604726614523236616, 166.3237786275915937 ) ) ;
#9403=VERTEX_POINT ( 'NONE', #11432 ) ;
#9404=ORIENTED_EDGE ( 'NONE', *, *, #36505, .F. ) ;
#9406=DIRECTION ( 'NONE',  ( 0.08715574274765150453, 0.000000000000000000, 0.9961946980917461003 ) ) ;
#9408=CARTESIAN_POINT ( 'NONE',  ( 26.75643035624999655, 3.323476615752271712, -6.628124999385471838 ) ) ;
#9411=CARTESIAN_POINT ( 'NONE',  ( 21.00000000000000355, 0.000000000000000000, 50.00000000000001421 ) ) ;
#9415=CARTESIAN_POINT ( 'NONE',  ( 36.85406125198851157, -3.604726614523238837, 159.5758215996624187 ) ) ;
#9428=CARTESIAN_POINT ( 'NONE',  ( 37.40314243129871841, -3.604726614523238837, 165.8518481976404360 ) ) ;
#9436=CARTESIAN_POINT ( 'NONE',  ( 27.67916667000801212, 5.196152422706636465, 160.7643641140699344 ) ) ;
#9439=CARTESIAN_POINT ( 'NONE',  ( 27.51944227705346790, -5.407089921784859143, 160.3360300724413321 ) ) ;
#9440=CARTESIAN_POINT ( 'NONE',  ( 18.12178482187499640, 4.985214923628404904, -9.665624999385475036 ) ) ;
#9441=CARTESIAN_POINT ( 'NONE',  ( 37.35088046919665317, 3.464101615137854751, 168.0491394851085829 ) ) ;
#9442=CARTESIAN_POINT ( 'NONE',  ( 31.09835460584942624, -7.209453229046482114, 165.4247213166986796 ) ) ;
#9443=CARTESIAN_POINT ( 'NONE',  ( 30.95863305570354385, -6.928203230275514990, 163.8276966907081658 ) ) ;
#9448=EDGE_CURVE ( 'NONE', #25471, #6369, #31707, .T. ) ;
#9451=EDGE_LOOP ( 'NONE', ( #30221, #2316, #13727, #34332 ) ) ;
#9455=CARTESIAN_POINT ( 'NONE',  ( 23.87821517812500005, -4.985214923628404016, -5.053124999385483207 ) ) ;
#9460=EDGE_CURVE ( 'NONE', #23156, #22401, #12899, .T. ) ;
#9467=LINE ( 'NONE', #17753, #8537 ) ;
#9472=CARTESIAN_POINT ( 'NONE',  ( 31.06403703214253653, -7.209453229046475009, 165.0324696543250411 ) ) ;
#9484=CARTESIAN_POINT ( 'NONE',  ( 31.31896757967941980, 7.209453229046475009, 167.9463391462434174 ) ) ;
#9485=CARTESIAN_POINT ( 'NONE',  ( 18.12178482187499640, 4.985214923628404904, -3.815624999385480720 ) ) ;
#9489=DIRECTION ( 'NONE',  ( 0.08715574274765150453, 0.000000000000000000, 0.9961946980917461003 ) ) ;
#9490=CARTESIAN_POINT ( 'NONE',  ( 15.00000000000000000, 0.000000000000000000, -7.593749998770965348 ) ) ;
#9498=CARTESIAN_POINT ( 'NONE',  ( 23.87821517812500005, -4.985214923628404016, -1.340624999385475746 ) ) ;
#9500=( BOUNDED_CURVE ( )  B_SPLINE_CURVE ( 2, ( #15693, #24588, #21573, #1834, #10554, #13403, #24952 ),
 .UNSPECIFIED., .F., .F. ) 
 B_SPLINE_CURVE_WITH_KNOTS ( ( 3, 2, 2, 3 ),
 ( 0.8043478260869548757, 0.8115942028985493328, 0.8188405797101435679, 0.8260869565217380250 ),
 .UNSPECIFIED. ) 
 CURVE ( )  GEOMETRIC_REPRESENTATION_ITEM ( )  RATIONAL_B_SPLINE_CURVE ( ( 1.000000000000030864, 0.8660254037844079544, 1.000000000000000000, 0.8660254037844387076, 1.000000000000000000, 0.8660254037844592467, 0.9999999999999794609 ) ) 
 REPRESENTATION_ITEM ( '' )  );
#9502=CARTESIAN_POINT ( 'NONE',  ( 15.00000000000000178, -3.464101615137757051, -8.006249998770949006 ) ) ;
#9506=EDGE_LOOP ( 'NONE', ( #27941, #21028, #28460, #9670 ) ) ;
#9508=CARTESIAN_POINT ( 'NONE',  ( 24.82951852428355011, 0.000000000000000000, 165.4085247487197989 ) ) ;
#9516=CARTESIAN_POINT ( 'NONE',  ( 34.30794447475221176, 5.407089921784857367, 166.2920375277922460 ) ) ;
#9531=CARTESIAN_POINT ( 'NONE',  ( 14.99999999999954348, 3.464101615137491930, -1.387499999999978417 ) ) ;
#9533=CARTESIAN_POINT ( 'NONE',  ( 37.64499961742345135, 3.604726614523243278, 168.6162884848450005 ) ) ;
#9536=CARTESIAN_POINT ( 'NONE',  ( 16.07192114941521766, -3.422577806627481234, -8.000000000000001776 ) ) ;
#9543=CARTESIAN_POINT ( 'NONE',  ( 15.24356964374999990, 3.323476615752268604, -4.340624999385463312 ) ) ;
#9548=CARTESIAN_POINT ( 'NONE',  ( 20.99999999999999645, -6.646953231504538984, -5.878124999385467397 ) ) ;
#9558=CARTESIAN_POINT ( 'NONE',  ( 26.75643035624999655, 7.049594010296217766E-16, -6.328124999385481786 ) ) ;
#9563=CARTESIAN_POINT ( 'NONE',  ( 33.84263025878871645, -5.196152422706629359, 162.3707958259794566 ) ) ;
#9567=CARTESIAN_POINT ( 'NONE',  ( 36.86059793269458140, 3.604726614523243278, 159.6505362020193104 ) ) ;
#9575=CARTESIAN_POINT ( 'NONE',  ( 37.30185536379384814, 3.464101615137935575, 167.4887799662076304 ) ) ;
#9581=CARTESIAN_POINT ( 'NONE',  ( 21.00000000000000000, -6.928203230275506996, -6.637499999999977085 ) ) ;
#9583=CARTESIAN_POINT ( 'NONE',  ( 20.99999999999999645, 6.928203230275506996, -6.806249998770949716 ) ) ;
#9585=CARTESIAN_POINT ( 'NONE',  ( 34.25565102910361759, -5.407089921784855591, 165.6943207089371981 ) ) ;
#9586=CARTESIAN_POINT ( 'NONE',  ( 29.51960950058489175, 6.028781714493277377, 159.5765249394674470 ) ) ;
#9591=ORIENTED_EDGE ( 'NONE', *, *, #5304, .F. ) ;
#9595=CARTESIAN_POINT ( 'NONE',  ( 37.14170668649535401, 7.347880794884125653E-16, 165.6582722084640125 ) ) ;
#9596=CARTESIAN_POINT ( 'NONE',  ( 23.87821517812500005, -4.985214923628404016, -8.990624999385465443 ) ) ;
#9600=EDGE_CURVE ( 'NONE', #15757, #18882, #14587, .T. ) ;
#9602=LINE ( 'NONE', #3535, #25814 ) ;
#9603=CARTESIAN_POINT ( 'NONE',  ( 25.25927379726832100, -3.464101615137757051, 167.5260017485858555 ) ) ;
#9613=ORIENTED_EDGE ( 'NONE', *, *, #33334, .T. ) ;
#9615=CARTESIAN_POINT ( 'NONE',  ( 20.99999999999999645, 6.928203230275506996, -7.762500000000014388 ) ) ;
#9616=CARTESIAN_POINT ( 'NONE',  ( 24.98477879236699195, 0.000000000000000000, 49.65137702900941008 ) ) ;
#9617=CARTESIAN_POINT ( 'NONE',  ( 24.98639886122932197, 0.000000000000000000, 167.2016752052849426 ) ) ;
#9623=( BOUNDED_CURVE ( )  B_SPLINE_CURVE ( 2, ( #21066, #30143, #3611, #757, #23900, #35442, #9490 ),
 .UNSPECIFIED., .F., .F. ) 
 B_SPLINE_CURVE_WITH_KNOTS ( ( 3, 2, 2, 3 ),
 ( 0.6739130434782618639, 0.6811594202898562100, 0.6884057971014503341, 0.6956521739130446802 ),
 .UNSPECIFIED. ) 
 CURVE ( )  GEOMETRIC_REPRESENTATION_ITEM ( )  RATIONAL_B_SPLINE_CURVE ( ( 0.9999999999999815703, 0.8660254037844571373, 1.000000000000000000, 0.8660254037844387076, 1.000000000000000000, 0.8660254037844161701, 1.000000000000022649 ) ) 
 REPRESENTATION_ITEM ( '' )  );
#9627=CARTESIAN_POINT ( 'NONE',  ( 14.99999999999946709, 3.464101615137446188, -5.437500000000002665 ) ) ;
#9629=CARTESIAN_POINT ( 'NONE',  ( 15.00000000000000178, -3.464101615137757051, -0.8624999999999944933 ) ) ;
#9630=CARTESIAN_POINT ( 'NONE',  ( 37.18092677073180141, 7.347880794884125653E-16, 166.1065598226053055 ) ) ;
#9632=CARTESIAN_POINT ( 'NONE',  ( 37.36392234706227811, -3.604726614523238837, 165.4035605834991145 ) ) ;
#9633=CARTESIAN_POINT ( 'NONE',  ( 28.03214742813599969, 5.196152422706636465, 164.7989526413415149 ) ) ;
#9638=ORIENTED_EDGE ( 'NONE', *, *, #19300, .F. ) ;
#9641=LINE ( 'NONE', #9826, #6566 ) ;
#9644=CARTESIAN_POINT ( 'NONE',  ( 26.75643035624999655, -3.323476615752267715, -7.715624999385478411 ) ) ;
#9654=CARTESIAN_POINT ( 'NONE',  ( 31.45868912971818432, 0.000000000000000000, 169.5433637710095809 ) ) ;
#9658=CARTESIAN_POINT ( 'NONE',  ( 18.00000000000000000, 5.196152422706630247, -1.818749998770963217 ) ) ;
#9659=CARTESIAN_POINT ( 'NONE',  ( 37.29038468911893034, -3.604726614523235284, 164.5630213069841830 ) ) ;
#9664=CARTESIAN_POINT ( 'NONE',  ( 25.36712902881149745, -3.464101615137806345, 168.7587926862500183 ) ) ;
#9670=ORIENTED_EDGE ( 'NONE', *, *, #25721, .F. ) ;
#9671=CARTESIAN_POINT ( 'NONE',  ( 25.06647319987872535, 3.604726614523236616, 168.1169290841567090 ) ) ;
#9672=CARTESIAN_POINT ( 'NONE',  ( 15.24356964375000167, -3.323476615752272600, -2.803124999385491645 ) ) ;
#9677=CARTESIAN_POINT ( 'NONE',  ( 28.13346597918727099, -5.196152422706632912, 165.9570289790974869 ) ) ;
#9685=CARTESIAN_POINT ( 'NONE',  ( 15.24356964374999990, 3.323476615752268604, -2.428124999385457894 ) ) ;
#9687=CARTESIAN_POINT ( 'NONE',  ( 24.00000000000000000, -5.196152422706629359, -8.343749998770967125 ) ) ;
#9695=CARTESIAN_POINT ( 'NONE',  ( 24.83278686463658502, -3.604726614523244610, 165.4458820498982163 ) ) ;
#9699=DIRECTION ( 'NONE',  ( 0.08715574274765150453, 0.000000000000000000, 0.9961946980917461003 ) ) ;
#9702=CARTESIAN_POINT ( 'NONE',  ( 31.18169728485186454, -7.209453229046475009, 166.3773324967488918 ) ) ;
#9710=CARTESIAN_POINT ( 'NONE',  ( 26.99999999999999289, 0.000000000000000000, -8.000000000000000000 ) ) ;
#9719=AXIS2_PLACEMENT_3D ( 'NONE', #25908, #37454, #35926 ) ;
#9721=( BOUNDED_CURVE ( )  B_SPLINE_CURVE ( 2, ( #31950, #28918, #14708, #5982, #2952, #14522, #29097 ),
 .UNSPECIFIED., .F., .F. ) 
 B_SPLINE_CURVE_WITH_KNOTS ( ( 3, 2, 2, 3 ),
 ( 0.5652173913043470055, 0.5724637681159411295, 0.5797101449275352536, 0.5869565217391293777 ),
 .UNSPECIFIED. ) 
 CURVE ( )  GEOMETRIC_REPRESENTATION_ITEM ( )  RATIONAL_B_SPLINE_CURVE ( ( 1.000000000000014433, 0.8660254037844243857, 1.000000000000000000, 0.8660254037844387076, 1.000000000000000000, 0.8660254037844592467, 0.9999999999999794609 ) ) 
 REPRESENTATION_ITEM ( '' )  );
#9725=EDGE_CURVE ( 'NONE', #12708, #4247, #31512, .T. ) ;
#9727=CARTESIAN_POINT ( 'NONE',  ( 36.71028575989448228, 7.347880794884125653E-16, 160.7271084529098744 ) ) ;
#9735=CARTESIAN_POINT ( 'NONE',  ( 15.24356964374999990, 3.323476615752268604, -3.890624999385467575 ) ) ;
#9738=ORIENTED_EDGE ( 'NONE', *, *, #17124, .F. ) ;
#9739=CARTESIAN_POINT ( 'NONE',  ( 23.87821517812500005, -4.985214923628404016, -7.640624999385475569 ) ) ;
#9744=CARTESIAN_POINT ( 'NONE',  ( 30.65467740297821919, -6.928203230275506996, 160.3534676823375378 ) ) ;
#9748=CARTESIAN_POINT ( 'NONE',  ( 18.12178482187499640, 4.985214923628404904, -7.078124999385481786 ) ) ;
#9757=ORIENTED_EDGE ( 'NONE', *, *, #9243, .F. ) ;
#9760=CARTESIAN_POINT ( 'NONE',  ( 18.00000000000000355, -5.196152422706632912, -1.218749998770946030 ) ) ;
#9767=CARTESIAN_POINT ( 'NONE',  ( 18.00000000000000355, -5.196152422706632912, -7.574999999999998401 ) ) ;
#9770=CARTESIAN_POINT ( 'NONE',  ( 27.97700992647863316, 5.407089921784856479, 165.5660522374229799 ) ) ;
#9772=EDGE_CURVE ( 'NONE', #30148, #5563, #9721, .T. ) ;
#9775=ORIENTED_EDGE ( 'NONE', *, *, #9460, .T. ) ;
#9781=CARTESIAN_POINT ( 'NONE',  ( 15.24356964375000167, -3.323476615752272600, -8.203124999385472904 ) ) ;
#9788=CARTESIAN_POINT ( 'NONE',  ( 25.29195720079868792, 3.464101615137752166, 167.8995747603702853 ) ) ;
#9798=CARTESIAN_POINT ( 'NONE',  ( 14.99999999999962874, 3.464101615137538115, -7.687499999999983125 ) ) ;
#9800=CARTESIAN_POINT ( 'NONE',  ( 37.36392234706227811, -3.604726614523238837, 165.4035605834991145 ) ) ;
#9813=CARTESIAN_POINT ( 'NONE',  ( 26.99999999999962341, 3.464101615137969770, -5.587499999999994138 ) ) ;
#9815=CARTESIAN_POINT ( 'NONE',  ( 15.24356964374999990, 3.323476615752268604, -10.07812499938544804 ) ) ;
#9817=CARTESIAN_POINT ( 'NONE',  ( 27.67142010346968561, -5.407089921784865361, 162.0731445772388213 ) ) ;
#9818=CARTESIAN_POINT ( 'NONE',  ( 24.85073125303158292, 3.464101615137757051, 162.8563391000564593 ) ) ;
#9824=VERTEX_POINT ( 'NONE', #6362 ) ;
#9826=CARTESIAN_POINT ( 'NONE',  ( 15.02283181144952628, 7.347880794884122694E-16, 50.52293445648592751 ) ) ;
#9829=CARTESIAN_POINT ( 'NONE',  ( 21.00000000000000000, 6.646953231504538984, -5.765624999385476457 ) ) ;
#9835=ADVANCED_FACE ( 'NONE', ( #32133 ), #17933, .T. ) ;
#9839=DIRECTION ( 'NONE',  ( 0.000000000000000000, 0.000000000000000000, 1.000000000000000000 ) ) ;
#9843=CARTESIAN_POINT ( 'NONE',  ( 15.00000000000000000, 0.000000000000000000, -0.07031249969274844247 ) ) ;
#9844=CARTESIAN_POINT ( 'NONE',  ( 27.83320295094501162, -5.407089921784859143, 163.9223309855715911 ) ) ;
#9848=CARTESIAN_POINT ( 'NONE',  ( 26.99999999999936051, -3.464101615138118984, -5.606249998770957532 ) ) ;
#9855=CARTESIAN_POINT ( 'NONE',  ( 37.45380170677077558, 3.604726614523238837, 166.4308863659062183 ) ) ;
#9856=CARTESIAN_POINT ( 'NONE',  ( 26.75643035624999655, 7.049594010296217766E-16, -2.615624999385474325 ) ) ;
#9858=CARTESIAN_POINT ( 'NONE',  ( 24.53624671473563623, -4.728541327911522707, -8.000000000000000000 ) ) ;
#9864=ORIENTED_EDGE ( 'NONE', *, *, #15765, .T. ) ;
#9868=CARTESIAN_POINT ( 'NONE',  ( 18.12178482187500350, -4.985214923628407568, -0.5156249993854555846 ) ) ;
#9870=CARTESIAN_POINT ( 'NONE',  ( 24.00000000000000000, -5.196152422706629359, -9.243749998770949716 ) ) ;
#9875=ORIENTED_EDGE ( 'NONE', *, *, #28642, .F. ) ;
#9879=CARTESIAN_POINT ( 'NONE',  ( 30.94147426890365438, -7.209453229046482114, 163.6315708601335359 ) ) ;
#9882=LINE ( 'NONE', #24109, #35143 ) ;
#9885=CARTESIAN_POINT ( 'NONE',  ( 31.14247720061542424, -7.209453229046475009, 165.9290448826076272 ) ) ;
#9894=ORIENTED_EDGE ( 'NONE', *, *, #11097, .T. ) ;
#9895=( NAMED_UNIT ( * ) PLANE_ANGLE_UNIT ( ) SI_UNIT ( $, .RADIAN. ) );
#9912=CARTESIAN_POINT ( 'NONE',  ( 18.12178482187499640, 4.985214923628404904, -4.378124999385474503 ) ) ;
#9916=CARTESIAN_POINT ( 'NONE',  ( 18.12178482187499640, 4.985214923628404904, -7.415624999385473259 ) ) ;
#9921=CARTESIAN_POINT ( 'NONE',  ( 27.62360488411350801, -5.196152422706632912, 160.1292899952607627 ) ) ;
#9927=EDGE_CURVE ( 'NONE', #26175, #4869, #2266, .T. ) ;
#9928=CARTESIAN_POINT ( 'NONE',  ( 15.24356964374999990, 3.323476615752268604, -7.040624999385501681 ) ) ;
#9951=DIRECTION ( 'NONE',  ( 0.000000000000000000, 0.000000000000000000, 1.000000000000000000 ) ) ;
#9954=CARTESIAN_POINT ( 'NONE',  ( 27.83320295094501162, -5.407089921784859143, 163.9223309855715911 ) ) ;
#9957=VERTEX_POINT ( 'NONE', #13844 ) ;
#9962=CARTESIAN_POINT ( 'NONE',  ( 23.87821517812499650, 4.985214923628404904, -1.190624999385464511 ) ) ;
#9965=CARTESIAN_POINT ( 'NONE',  ( 26.75643035624999655, -3.323476615752267715, -8.053124999385453009 ) ) ;
#9972=CARTESIAN_POINT ( 'NONE',  ( 34.24790446256528753, 5.196152422706631135, 167.0031011721061134 ) ) ;
#9977=CARTESIAN_POINT ( 'NONE',  ( 24.81477950914817754, 0.000000000000000000, 162.4454087870936121 ) ) ;
#9981=ORIENTED_EDGE ( 'NONE', *, *, #29819, .T. ) ;
#9985=CARTESIAN_POINT ( 'NONE',  ( 24.91122703310946918, -3.604726614523244610, 166.3424572781808024 ) ) ;
#9997=CARTESIAN_POINT ( 'NONE',  ( 27.97700992647863316, 5.407089921784856479, 165.5660522374229799 ) ) ;
#10000=CARTESIAN_POINT ( 'NONE',  ( 21.00000000000000000, -6.646953231504538984, -9.928124999385461891 ) ) ;
#10002=CARTESIAN_POINT ( 'NONE',  ( 30.84342405831255007, 7.209453229046482114, 162.5108518247803318 ) ) ;
#10003=CARTESIAN_POINT ( 'NONE',  ( 27.79682692271734012, 5.196152422706636465, 162.1092269564937851 ) ) ;
#10008=ORIENTED_EDGE ( 'NONE', *, *, #25253, .T. ) ;
#10013=CARTESIAN_POINT ( 'NONE',  ( 15.24356964375000167, -3.323476615752272600, -6.065624999385484273 ) ) ;
#10017=CARTESIAN_POINT ( 'NONE',  ( 20.99999999999999645, -6.928203230275506996, -6.581249998770967835 ) ) ;
#10026=CARTESIAN_POINT ( 'NONE',  ( 24.67427235751429393, 3.604726614523236616, 163.6340529427438639 ) ) ;
#10029=CARTESIAN_POINT ( 'NONE',  ( 26.99999999999999645, 7.347880794884117764E-16, -4.725000000000006750 ) ) ;
#10036=DIRECTION ( 'NONE',  ( 0.000000000000000000, 0.000000000000000000, 1.000000000000000000 ) ) ;
#10039=CARTESIAN_POINT ( 'NONE',  ( 37.33287311370841621, 7.646167579472015790E-16, 165.0486662223039218 ) ) ;
#10040=CARTESIAN_POINT ( 'NONE',  ( 21.00000000000000000, 6.646953231504538984, -3.853124999385470595 ) ) ;
#10044=CARTESIAN_POINT ( 'NONE',  ( 28.38512818626399081, 5.196152422706636465, 168.8335411686130669 ) ) ;
#10051=ORIENTED_EDGE ( 'NONE', *, *, #30342, .T. ) ;
#10052=VERTEX_POINT ( 'NONE', #10987 ) ;
#10055=CARTESIAN_POINT ( 'NONE',  ( 26.75643035624999655, 7.049594010296217766E-16, -0.8156249993854780556 ) ) ;
#10057=CARTESIAN_POINT ( 'NONE',  ( 21.00000000000000000, -6.646953231504538984, -0.5906249993854776337 ) ) ;
#10058=EDGE_CURVE ( 'NONE', #31332, #11570, #34106, .T. ) ;
#10059=ORIENTED_EDGE ( 'NONE', *, *, #36489, .F. ) ;
#10064=CARTESIAN_POINT ( 'NONE',  ( 24.67590652769081316, -3.604726614523244610, 163.6527315933331295 ) ) ;
#10070=( NAMED_UNIT ( * ) PLANE_ANGLE_UNIT ( ) SI_UNIT ( $, .RADIAN. ) );
#10075=CARTESIAN_POINT ( 'NONE',  ( 37.45380170677077558, 3.604726614523238837, 166.4308863659062183 ) ) ;
#10077=ORIENTED_EDGE ( 'NONE', *, *, #13809, .F. ) ;
#10097=ORIENTED_EDGE ( 'NONE', *, *, #30257, .T. ) ;
#10102=CARTESIAN_POINT ( 'NONE',  ( 26.97716818855048260, 0.000000000000000000, 49.47706554351410801 ) ) ;
#10103=CARTESIAN_POINT ( 'NONE',  ( 15.24356964374999990, 0.000000000000000000, -4.753124999385488714 ) ) ;
#10106=CARTESIAN_POINT ( 'NONE',  ( 26.04366382382454859, 3.734992565117459140, -7.968838429997217254 ) ) ;
#10121=CARTESIAN_POINT ( 'NONE',  ( 20.00000000000024869, -5.916079783099657874, -7.999999999999998224 ) ) ;
#10138=ORIENTED_EDGE ( 'NONE', *, *, #26533, .T. ) ;
#10139=DIRECTION ( 'NONE',  ( 0.08715574274765150453, 0.000000000000000000, 0.9961946980917461003 ) ) ;
#10143=CARTESIAN_POINT ( 'NONE',  ( 30.96598682155142868, 7.209453229046475009, 163.9117506189718370 ) ) ;
#10149=ORIENTED_EDGE ( 'NONE', *, *, #29307, .F. ) ;
#10151=CARTESIAN_POINT ( 'NONE',  ( 20.99999999999999645, -6.646953231504538984, -0.4781249993854547187 ) ) ;
#10153=CARTESIAN_POINT ( 'NONE',  ( 21.00000000000000000, -6.646953231504538984, -7.678124999385482319 ) ) ;
#10156=CARTESIAN_POINT ( 'NONE',  ( 36.75931086529713099, 7.347880794884117764E-16, 161.2874679718108553 ) ) ;
#10159=CARTESIAN_POINT ( 'NONE',  ( 15.00000000000000355, 7.347880794884112834E-16, 50.26196565745150480 ) ) ;
#10160=CARTESIAN_POINT ( 'NONE',  ( 34.16946429409239983, 5.196152422706631135, 166.1065259438235557 ) ) ;
#10165=CARTESIAN_POINT ( 'NONE',  ( 23.87821517812499650, 4.985214923628404904, -1.753124999385485827 ) ) ;
#10171=CARTESIAN_POINT ( 'NONE',  ( 37.22668353578169587, -3.464101615137590073, 166.6295620403278122 ) ) ;
#10174=CARTESIAN_POINT ( 'NONE',  ( 37.20704201011650269, -3.604726614523238837, 163.6104101269339424 ) ) ;
#10190=CARTESIAN_POINT ( 'NONE',  ( 18.00000000000000000, 5.196152422706630247, -2.324999999999993960 ) ) ;
#10191=CARTESIAN_POINT ( 'NONE',  ( 24.59092967851185207, 3.604726614523240613, 162.6814417626936518 ) ) ;
#10192=CARTESIAN_POINT ( 'NONE',  ( 33.76745843056175289, 5.196152422706637353, 161.5115778976509944 ) ) ;
#10205=CARTESIAN_POINT ( 'NONE',  ( 23.87821517812500005, -4.985214923628404016, -7.303124999385484983 ) ) ;
#10218=CARTESIAN_POINT ( 'NONE',  ( 24.59583218904140978, 3.604726614523236616, 162.7374777144612779 ) ) ;
#10221=CARTESIAN_POINT ( 'NONE',  ( 24.00000000000000000, -5.196152422706629359, -3.843749998770962240 ) ) ;
#10228=EDGE_LOOP ( 'NONE', ( #23702, #4805, #8471, #29708, #35245, #3368, #31267, #31177, #24684, #10149, #14924, #11173, #773, #23433, #14704, #9404, #28967, #33137, #27626, #37011, #18458, #37479, #19196, #31222, #17591, #14716, #24736, #4500, #10077, #27748, #12658, #7181, #10427, #26265, #21309, #19263, #13602, #9757, #35338, #5378, #20013, #2774, #23288, #4402, #28047, #19356, #22556, #35706 ) ) ;
#10229=CARTESIAN_POINT ( 'NONE',  ( 37.17599277676264080, 7.646167579472015790E-16, 163.2555157657388065 ) ) ;
#10230=CARTESIAN_POINT ( 'NONE',  ( 21.00000000000000000, 6.646953231504538984, -5.203124999385457805 ) ) ;
#10232=CARTESIAN_POINT ( 'NONE',  ( 31.35083389806797527, -6.928203230275514990, 168.3105728321210393 ) ) ;
#10233=CARTESIAN_POINT ( 'NONE',  ( 15.00000000000000355, 7.347880794884112834E-16, -8.000000000000000000 ) ) ;
#10241=CARTESIAN_POINT ( 'NONE',  ( 23.87821517812499650, 4.985214923628404904, -3.890624999385472460 ) ) ;
#10243=CARTESIAN_POINT ( 'NONE',  ( 15.00000000000000000, 3.464101615137752166, -9.881249998770957887 ) ) ;
#10251=CARTESIAN_POINT ( 'NONE',  ( 30.68654372136677821, 7.209453229046482114, 160.7177013682151596 ) ) ;
#10254=DIRECTION ( 'NONE',  ( 0.08715574274765150453, 0.000000000000000000, 0.9961946980917461003 ) ) ;
#10257=EDGE_CURVE ( 'NONE', #24412, #20178, #16043, .T. ) ;
#10260=LINE ( 'NONE', #33576, #2793 ) ;
#10261=EDGE_CURVE ( 'NONE', #952, #18435, #20279, .T. ) ;
#10264=( BOUNDED_CURVE ( )  B_SPLINE_CURVE ( 2, ( #13146, #1764, #22427, #31320, #19592, #31141, #2503 ),
 .UNSPECIFIED., .F., .F. ) 
 B_SPLINE_CURVE_WITH_KNOTS ( ( 3, 2, 2, 3 ),
 ( 0.7173913043478249429, 0.7246376811594192890, 0.7318840579710136351, 0.7391304347826078702 ),
 .UNSPECIFIED. ) 
 CURVE ( )  GEOMETRIC_REPRESENTATION_ITEM ( )  RATIONAL_B_SPLINE_CURVE ( ( 1.000000000000020428, 0.8660254037844181685, 1.000000000000000000, 0.8660254037844387076, 1.000000000000000000, 0.8660254037844530295, 0.9999999999999856781 ) ) 
 REPRESENTATION_ITEM ( '' )  );
#10276=CARTESIAN_POINT ( 'NONE',  ( 27.00000000000058620, -3.464101615137410661, -1.556249998770949716 ) ) ;
#10278=CARTESIAN_POINT ( 'NONE',  ( 24.67097253372098820, -3.464101615137358703, 160.8016875364666305 ) ) ;
#10285=CARTESIAN_POINT ( 'NONE',  ( 15.24356964375000167, -3.323476615752272600, -7.865624999385466332 ) ) ;
#10290=CARTESIAN_POINT ( 'NONE',  ( 15.24356964374999990, 3.323476615752268604, -6.478124999385451055 ) ) ;
#10292=CARTESIAN_POINT ( 'NONE',  ( 34.44684893975629336, -5.407089921784861808, 167.8797228278759803 ) ) ;
#10293=VECTOR ( 'NONE', #19798, 1000.000000000000000 ) ;
#10295=CARTESIAN_POINT ( 'NONE',  ( 24.70365593725203368, 3.464101615137752166, 161.1752605482509750 ) ) ;
#10300=DIRECTION ( 'NONE',  ( 0.000000000000000000, 0.000000000000000000, 1.000000000000000000 ) ) ;
#10305=CARTESIAN_POINT ( 'NONE',  ( 27.00000000000031619, -3.464101615137567869, -7.912499999999997868 ) ) ;
#10309=DIRECTION ( 'NONE',  ( 0.08715574274765150453, 0.000000000000000000, 0.9961946980917461003 ) ) ;
#10314=CARTESIAN_POINT ( 'NONE',  ( 37.09921826190632999, -3.464101615137494594, 165.1726272931442452 ) ) ;
#10317=CARTESIAN_POINT ( 'NONE',  ( 25.09912511996950713, 0.000000000000000000, 165.6954939908422944 ) ) ;
#10329=CARTESIAN_POINT ( 'NONE',  ( 24.79520095057666396, 0.000000000000000000, 165.0162730863461604 ) ) ;
#10336=CARTESIAN_POINT ( 'NONE',  ( 26.99999999999999645, -3.464101615137751278, -4.256249998770931242 ) ) ;
#10337=CARTESIAN_POINT ( 'NONE',  ( 20.99999999999999645, 6.646953231504538984, -0.2531249993854407521 ) ) ;
#10339=CARTESIAN_POINT ( 'NONE',  ( 33.77726345172796840, 5.196152422706631135, 161.6236498024106822 ) ) ;
#10340=CARTESIAN_POINT ( 'NONE',  ( 18.12178482187499640, 4.985214923628404904, -7.865624999385478766 ) ) ;
#10346=CARTESIAN_POINT ( 'NONE',  ( 37.11555996377816058, 3.464101615137755275, 165.3594138002608247 ) ) ;
#10352=CARTESIAN_POINT ( 'NONE',  ( 18.12178482187500350, -4.985214923628407568, -2.878124999385472726 ) ) ;
#10358=CARTESIAN_POINT ( 'NONE',  ( 34.23483110115314787, -5.196152422706629359, 166.8536719673923017 ) ) ;
#10362=CARTESIAN_POINT ( 'NONE',  ( 37.21031035046954116, 7.646167579472024665E-16, 163.6477674281124450 ) ) ;
#10367=CARTESIAN_POINT ( 'NONE',  ( 20.99999999999999645, 6.928203230275506996, -2.756249998770956111 ) ) ;
#10376=VERTEX_POINT ( 'NONE', #30438 ) ;
#10377=CARTESIAN_POINT ( 'NONE',  ( 18.00000000000000355, -5.196152422706632912, -1.725000000000004308 ) ) ;
#10378=CARTESIAN_POINT ( 'NONE',  ( 27.81522707900330715, 5.407089921784862696, 163.7168658290902101 ) ) ;
#10379=CARTESIAN_POINT ( 'NONE',  ( 27.69224003142016954, -5.196152422706638241, 160.9137933187836609 ) ) ;
#10387=CARTESIAN_POINT ( 'NONE',  ( 15.00000000000000355, 7.347880794884112834E-16, -8.000000000000000000 ) ) ;
#10389=CARTESIAN_POINT ( 'NONE',  ( 26.75643035624999655, 7.049594010296217766E-16, -5.428124999385497418 ) ) ;
#10396=EDGE_CURVE ( 'NONE', #27950, #7860, #4457, .T. ) ;
#10401=EDGE_CURVE ( 'NONE', #34897, #34009, #10712, .T. ) ;
#10404=EDGE_CURVE ( 'NONE', #15602, #1464, #18478, .T. ) ;
#10406=CARTESIAN_POINT ( 'NONE',  ( 37.01911243981686539, 7.646167579472015790E-16, 161.4623653091736628 ) ) ;
#10416=VERTEX_POINT ( 'NONE', #24144 ) ;
#10417=CARTESIAN_POINT ( 'NONE',  ( 24.83115269446006934, 3.604726614523236616, 165.4272033993090076 ) ) ;
#10418=CARTESIAN_POINT ( 'NONE',  ( 18.12178482187500350, -4.985214923628407568, -5.465624999385465088 ) ) ;
#10420=CARTESIAN_POINT ( 'NONE',  ( 31.39005398230442268, -6.928203230275514990, 168.7588604462623039 ) ) ;
#10421=CARTESIAN_POINT ( 'NONE',  ( 30.68409246604844043, -6.928203230275514990, 160.6896833917191714 ) ) ;
#10423=DIRECTION ( 'NONE',  ( 0.08715574274765150453, 0.000000000000000000, 0.9961946980917461003 ) ) ;
#10426=ORIENTED_EDGE ( 'NONE', *, *, #15759, .F. ) ;
#10427=ORIENTED_EDGE ( 'NONE', *, *, #34596, .F. ) ;
#10428=VECTOR ( 'NONE', #12836, 1000.000000000000000 ) ;
#10431=CARTESIAN_POINT ( 'NONE',  ( 15.24356964375000167, -3.323476615752272600, -2.803124999385491645 ) ) ;
#10434=CARTESIAN_POINT ( 'NONE',  ( 21.00000000000000000, 6.928203230275506996, -9.056249998770928400 ) ) ;
#10436=ORIENTED_EDGE ( 'NONE', *, *, #31965, .F. ) ;
#10440=CARTESIAN_POINT ( 'NONE',  ( 33.79318086914889818, 5.407089921784862696, 160.4082625921878673 ) ) ;
#10454=LINE ( 'NONE', #4767, #34862 ) ;
#10458=DIRECTION ( 'NONE',  ( 0.9961946980917462113, 0.000000000000000000, -0.08715574274765118534 ) ) ;
#10465=AXIS2_PLACEMENT_3D ( 'NONE', #23912, #769, #18420 ) ;
#10470=CARTESIAN_POINT ( 'NONE',  ( 21.00000000000000000, -6.646953231504538984, -7.790624999385473259 ) ) ;
#10473=CARTESIAN_POINT ( 'NONE',  ( 23.87821517812499650, 4.985214923628404904, -7.940624999385470062 ) ) ;
#10475=CARTESIAN_POINT ( 'NONE',  ( 25.18576762276457259, -3.604726614523244610, 169.4804705771697968 ) ) ;
#10483=CARTESIAN_POINT ( 'NONE',  ( 26.99999999999999645, 7.347880794884117764E-16, -2.868749998770958598 ) ) ;
#10497=CARTESIAN_POINT ( 'NONE',  ( 37.22995187613445012, 7.347880794884117764E-16, 166.6669193415062580 ) ) ;
#10505=EDGE_LOOP ( 'NONE', ( #26264, #20176, #6313, #35665 ) ) ;
#10509=CARTESIAN_POINT ( 'NONE',  ( 24.68080903822037087, -3.604726614523240613, 163.7087675451007271 ) ) ;
#10510=CARTESIAN_POINT ( 'NONE',  ( 24.93243976185750554, 0.000000000000000000, 163.7902716295174912 ) ) ;
#10516=ORIENTED_EDGE ( 'NONE', *, *, #6720, .F. ) ;
#10517=CARTESIAN_POINT ( 'NONE',  ( 18.00000000000000000, 5.196152422706630247, -4.068749998770964993 ) ) ;
#10518=CARTESIAN_POINT ( 'NONE',  ( 26.75643035624999655, -3.323476615752267271, -0.4031249993854607028 ) ) ;
#10531=CARTESIAN_POINT ( 'NONE',  ( 24.94551312337678084, -3.464101615137757051, 163.9397008354555965 ) ) ;
#10535=CARTESIAN_POINT ( 'NONE',  ( 15.24356964375000167, -3.323476615752272600, -2.015624999385490668 ) ) ;
#10541=CARTESIAN_POINT ( 'NONE',  ( 30.86058284511243599, 6.928203230275514990, 162.7069776553549616 ) ) ;
#10545=CARTESIAN_POINT ( 'NONE',  ( 24.79029844004710625, 0.000000000000000000, 164.9602371345785343 ) ) ;
#10548=( BOUNDED_CURVE ( )  B_SPLINE_CURVE ( 2, ( #15259, #24166, #29274, #6728, #9760, #29841, #3313 ),
 .UNSPECIFIED., .F., .F. ) 
 B_SPLINE_CURVE_WITH_KNOTS ( ( 3, 2, 2, 3 ),
 ( 0.06521739130434869858, 0.07246376811594300305, 0.07971014492753727976, 0.08695652173913158423 ),
 .UNSPECIFIED. ) 
 CURVE ( )  GEOMETRIC_REPRESENTATION_ITEM ( )  RATIONAL_B_SPLINE_CURVE ( ( 0.9999999999999837907, 0.8660254037844549169, 1.000000000000000000, 0.8660254037844387076, 1.000000000000000000, 0.8660254037844173913, 1.000000000000021316 ) ) 
 REPRESENTATION_ITEM ( '' )  );
#10554=CARTESIAN_POINT ( 'NONE',  ( 27.73146011565660984, -5.196152422706638241, 161.3620809329249539 ) ) ;
#10562=CARTESIAN_POINT ( 'NONE',  ( 24.00000000000000000, -5.196152422706629359, -2.099999999999990763 ) ) ;
#10563=CARTESIAN_POINT ( 'NONE',  ( 27.86752052465190133, -5.407089921784865361, 164.3145826479452296 ) ) ;
#10564=CARTESIAN_POINT ( 'NONE',  ( 27.67916667000801212, 5.196152422706636465, 160.7643641140699344 ) ) ;
#10566=CARTESIAN_POINT ( 'NONE',  ( 29.51984228635672380, 5.908847293266075162, 159.3365288790247121 ) ) ;
#10572=CARTESIAN_POINT ( 'NONE',  ( 26.99999999999999645, 7.347880794884117764E-16, -3.824999999999994849 ) ) ;
#10575=CARTESIAN_POINT ( 'NONE',  ( 15.24356964374999990, 0.000000000000000000, -7.903124999385474858 ) ) ;
#10588=CARTESIAN_POINT ( 'NONE',  ( 30.76988640036921652, 7.209453229046475009, 161.6703125482654286 ) ) ;
#10589=CARTESIAN_POINT ( 'NONE',  ( 26.99999999999999645, -3.464101615137751278, -1.106249998770961307 ) ) ;
#10595=DIRECTION ( 'NONE',  ( 1.000000000000000000, 0.000000000000000000, 0.000000000000000000 ) ) ;
#10598=CARTESIAN_POINT ( 'NONE',  ( 34.07262396933355575, 5.407089921784857367, 163.6023118429445162 ) ) ;
#10599=CARTESIAN_POINT ( 'NONE',  ( 15.24356964374999990, 0.000000000000000000, -5.990624999385463667 ) ) ;
#10602=CARTESIAN_POINT ( 'NONE',  ( 34.31653960987195973, 5.196152422706637353, 167.7876044956290116 ) ) ;
#10606=VECTOR ( 'NONE', #9489, 1000.000000000000000 ) ;
#10610=ORIENTED_EDGE ( 'NONE', *, *, #8355, .T. ) ;
#10611=ADVANCED_BREP_SHAPE_REPRESENTATION ( '', ( #21232, #17215 ), #34722 ) ;
#10614=ADVANCED_FACE ( 'NONE', ( #7535 ), #32927, .T. ) ;
#10615=CARTESIAN_POINT ( 'NONE',  ( 26.75643035624999655, 7.049594010296217766E-16, -3.065624999385479832 ) ) ;
#10618=CARTESIAN_POINT ( 'NONE',  ( 18.00000000000000000, 5.196152422706630247, -10.36874999877096570 ) ) ;
#10626=CARTESIAN_POINT ( 'NONE',  ( 25.08932009880328096, 0.000000000000000000, 165.5834220860826349 ) ) ;
#10628=CARTESIAN_POINT ( 'NONE',  ( 37.37702719191401002, 7.347880794884125653E-16, 168.3479978933117422 ) ) ;
#10638=ORIENTED_EDGE ( 'NONE', *, *, #2939, .T. ) ;
#10650=CARTESIAN_POINT ( 'NONE',  ( 26.99999999999999645, -3.464101615137751278, -8.812499999999992895 ) ) ;
#10656=CARTESIAN_POINT ( 'NONE',  ( 23.87821517812500005, -4.985214923628404016, -7.303124999385484983 ) ) ;
#10659=( GEOMETRIC_REPRESENTATION_CONTEXT ( 3 ) GLOBAL_UNCERTAINTY_ASSIGNED_CONTEXT ( ( #25255 ) ) GLOBAL_UNIT_ASSIGNED_CONTEXT ( ( #1171, #9895, #33018 ) ) REPRESENTATION_CONTEXT ( 'NONE', 'WORKASPACE' ) );
#10663=CARTESIAN_POINT ( 'NONE',  ( 34.49914238540488043, 5.407089921784862696, 168.4774396467310282 ) ) ;
#10670=CARTESIAN_POINT ( 'NONE',  ( 26.99999999999999645, 7.347880794884117764E-16, -6.975000000000008527 ) ) ;
#10671=CARTESIAN_POINT ( 'NONE',  ( 30.81155773992399460, -6.928203230275506996, 162.1466181389027099 ) ) ;
#10686=CARTESIAN_POINT ( 'NONE',  ( 23.99999999999999645, 5.196152422706631135, -5.493749998770947052 ) ) ;
#10698=CARTESIAN_POINT ( 'NONE',  ( 36.97662401522738662, -3.604726614523235284, 160.9767203938538955 ) ) ;
#10701=ORIENTED_EDGE ( 'NONE', *, *, #28626, .F. ) ;
#10705=CARTESIAN_POINT ( 'NONE',  ( 15.00000000000000000, 0.000000000000000000, -5.343749998770963572 ) ) ;
#10706=CARTESIAN_POINT ( 'NONE',  ( 23.87821517812500005, -4.985214923628404016, -3.140624999385472016 ) ) ;
#10712=( BOUNDED_CURVE ( )  B_SPLINE_CURVE ( 2, ( #18515, #13369, #24924, #10337, #13002, #27211, #36477, #10518, #36108, #10151, #35731, #22097, #33647, #24375, #32894, #7686, #30806, #21725, #4828, #16037, #16409, #27955, #13557, #33275, #1615, #12805, #13185, #30054, #9962, #27586, #35919, #24740, #7132, #21354, #6946, #21542, #33089, #13752, #25667, #22466, #11269, #37403, #8059, #30997, #34013, #34570, #8429, #14115, #16778, #28140, #36668, #28323, #8610, #28688, #37034, #7874, #17335, #16962, #5016, #20180, #31728, #2728, #19998, #25298, #19634, #22655, #10894, #5757, #16596, #2548, #37223, #25855, #31542, #19447, #11081, #31180, #5202, #36850, #33836, #2361, #10706, #13935, #19821, #25483, #28879, #14302, #34202, #2170, #2913, #28505, #8247, #25111, #22283, #31357, #5382, #22839, #34387, #5567, #11453, #17152, #23022, #14860, #11633, #625, #3287, #9171, #6129, #23389, #23765, #26594, #29441, #32661, #3477, #14669, #20739, #15046, #3100, #23207, #6702, #26219, #34755, #255, #17522, #31913, #12193, #35306, #8799, #29057, #32282, #9360, #11820, #20935, #20370, #32470, #21122, #20553, #23578, #26408, #34937, #5943, #6326, #8982, #35122, #18274, #26785, #29816, #35500, #15235, #6513, #29629, #14485, #3665, #17897, #9548, #816, #18088, #12387, #32097, #23957, #26039, #67, #17706, #29247, #441, #12006, #24514, #33415, #6893, #27541, #10290, #36063, #15994, #4600, #13138, #21862, #32846, #13323, #1002, #24694, #7454, #27352, #7268, #36246, #1382, #1569, #19029, #21676, #3851, #24883, #30389, #30009, #18844, #15611, #33230, #9916, #21499, #1757, #35686, #16178, #24332, #9739, #18468, #4039, #36430, #30584, #27728, #12954, #12577, #10473, #10106, #4411 ),
 .UNSPECIFIED., .F., .F. ) 
 B_SPLINE_CURVE_WITH_KNOTS ( ( 3, 2, 2, 2, 2, 2, 2, 2, 2, 2, 2, 2, 2, 2, 2, 2, 2, 2, 2, 2, 2, 2, 2, 2, 2, 2, 2, 2, 2, 2, 2, 2, 2, 2, 2, 2, 2, 2, 2, 2, 2, 2, 2, 2, 2, 2, 2, 2, 2, 2, 2, 2, 2, 2, 2, 2, 2, 2, 2, 2, 2, 2, 2, 2, 2, 2, 2, 2, 2, 2, 2, 2, 2, 2, 2, 2, 2, 2, 2, 2, 2, 2, 2, 2, 2, 2, 2, 2, 2, 2, 2, 2, 2, 2, 2, 2, 2, 2, 2, 2, 2, 2, 2, 2, 2, 3 ),
 ( 0.000000000000000000, 0.007246376811594202987, 0.01449275362318840597, 0.02173913043478260809, 0.02898550724637681195, 0.03623188405797101580, 0.04347826086956521618, 0.05072463768115942351, 0.05797101449275362389, 0.06521739130434782428, 0.07246376811594203160, 0.07971014492753622505, 0.08695652173913043237, 0.09420289855072463969, 0.1014492753623188470, 0.1086956521739130266, 0.1159420289855072478, 0.1231884057971014551, 0.1304347826086956486, 0.1376811594202898559, 0.1449275362318840632, 0.1521739130434782705, 0.1594202898550724501, 0.1666666666666666574, 0.1739130434782608647, 0.1811594202898550721, 0.1884057971014492794, 0.1956521739130435145, 0.2028985507246376940, 0.2101449275362318736, 0.2173913043478260532, 0.2246376811594202882, 0.2318840579710144956, 0.2391304347826087029, 0.2463768115942029102, 0.2536231884057971175, 0.2608695652173912971, 0.2681159420289855322, 0.2753623188405797118, 0.2826086956521738913, 0.2898550724637681264, 0.2971014492753623060, 0.3043478260869565410, 0.3115942028985507206, 0.3188405797101449002, 0.3260869565217391353, 0.3333333333333333148, 0.3405797101449275499, 0.3478260869565217295, 0.3550724637681159090, 0.3623188405797101441, 0.3695652173913043237, 0.3768115942028985588, 0.3840579710144927383, 0.3913043478260870289, 0.3985507246376811530, 0.4057971014492753881, 0.4130434782608696231, 0.4202898550724637472, 0.4275362318840579823, 0.4347826086956521063, 0.4420289855072463969, 0.4492753623188405765, 0.4565217391304347561, 0.4637681159420289911, 0.4710144927536232262, 0.4782608695652174058, 0.4855072463768115854, 0.4927536231884058204, 0.5000000000000000000, 0.5072463768115942351, 0.5144927536231883591, 0.5217391304347825942, 0.5289855072463768293, 0.5362318840579710644, 0.5434782608695651884, 0.5507246376811594235, 0.5579710144927536586, 0.5652173913043477826, 0.5724637681159420177, 0.5797101449275362528, 0.5869565217391304879, 0.5942028985507246119, 0.6014492753623188470, 0.6086956521739130821, 0.6159420289855072062, 0.6231884057971014412, 0.6304347826086956763, 0.6376811594202898004, 0.6449275362318840354, 0.6521739130434782705, 0.6594202898550725056, 0.6666666666666666297, 0.6739130434782608647, 0.6811594202898550998, 0.6884057971014492239, 0.6956521739130434590, 0.7028985507246376940, 0.7101449275362318181, 0.7173913043478260532, 0.7246376811594202882, 0.7318840579710144123, 0.7391304347826086474, 0.7463768115942028825, 0.7536231884057971175, 0.7592621468213750502 ),
 .UNSPECIFIED. ) 
 CURVE ( )  GEOMETRIC_REPRESENTATION_ITEM ( )  RATIONAL_B_SPLINE_CURVE ( ( 1.000000000000000000, 0.8660254037844387076, 1.000000000000000000, 0.8660254037844387076, 1.000000000000000000, 0.8660254037844387076, 1.000000000000000000, 0.8660254037844387076, 1.000000000000000000, 0.8660254037844387076, 1.000000000000000000, 0.8660254037844387076, 1.000000000000000000, 0.8660254037844387076, 1.000000000000000000, 0.8660254037844387076, 1.000000000000000000, 0.8660254037844387076, 1.000000000000000000, 0.8660254037844387076, 1.000000000000000000, 0.8660254037844387076, 1.000000000000000000, 0.8660254037844387076, 1.000000000000000000, 0.8660254037844387076, 1.000000000000000000, 0.8660254037844387076, 1.000000000000000000, 0.8660254037844387076, 1.000000000000000000, 0.8660254037844387076, 1.000000000000000000, 0.8660254037844387076, 1.000000000000000000, 0.8660254037844387076, 1.000000000000000000, 0.8660254037844387076, 1.000000000000000000, 0.8660254037844387076, 1.000000000000000000, 0.8660254037844387076, 1.000000000000000000, 0.8660254037844387076, 1.000000000000000000, 0.8660254037844387076, 1.000000000000000000, 0.8660254037844387076, 1.000000000000000000, 0.8660254037844387076, 1.000000000000000000, 0.8660254037844387076, 1.000000000000000000, 0.8660254037844387076, 1.000000000000000000, 0.8660254037844387076, 1.000000000000000000, 0.8660254037844387076, 1.000000000000000000, 0.8660254037844387076, 1.000000000000000000, 0.8660254037844387076, 1.000000000000000000, 0.8660254037844387076, 1.000000000000000000, 0.8660254037844387076, 1.000000000000000000, 0.8660254037844387076, 1.000000000000000000, 0.8660254037844387076, 1.000000000000000000, 0.8660254037844387076, 1.000000000000000000, 0.8660254037844387076, 1.000000000000000000, 0.8660254037844387076, 1.000000000000000000, 0.8660254037844387076, 1.000000000000000000, 0.8660254037844387076, 1.000000000000000000, 0.8660254037844387076, 1.000000000000000000, 0.8660254037844387076, 1.000000000000000000, 0.8660254037844387076, 1.000000000000000000, 0.8660254037844387076, 1.000000000000000000, 0.8660254037844387076, 1.000000000000000000, 0.8660254037844387076, 1.000000000000000000, 0.8660254037844387076, 1.000000000000000000, 0.8660254037844387076, 1.000000000000000000, 0.8660254037844387076, 1.000000000000000000, 0.8660254037844387076, 1.000000000000000000, 0.8660254037844387076, 1.000000000000000000, 0.8660254037844387076, 1.000000000000000000, 0.8660254037844387076, 1.000000000000000000, 0.8660254037844387076, 1.000000000000000000, 0.8660254037844387076, 1.000000000000000000, 0.8660254037844387076, 1.000000000000000000, 0.8660254037844387076, 1.000000000000000000, 0.8660254037844387076, 1.000000000000000000, 0.8660254037844387076, 1.000000000000000000, 0.8660254037844387076, 1.000000000000000000, 0.8660254037844387076, 1.000000000000000000, 0.8660254037844387076, 1.000000000000000000, 0.8660254037844387076, 1.000000000000000000, 0.8660254037844387076, 1.000000000000000000, 0.8660254037844387076, 1.000000000000000000, 0.8660254037844387076, 1.000000000000000000, 0.8660254037844387076, 1.000000000000000000, 0.8660254037844387076, 1.000000000000000000, 0.8660254037844387076, 1.000000000000000000, 0.8660254037844387076, 1.000000000000000000, 0.8660254037844387076, 1.000000000000000000, 0.8660254037844387076, 1.000000000000000000, 0.8660254037844387076, 1.000000000000000000, 0.8660254037844387076, 1.000000000000000000, 0.8660254037844387076, 1.000000000000000000, 0.8660254037844387076, 1.000000000000000000, 0.8660254037844387076, 1.000000000000000000, 0.8660254037844387076, 1.000000000000000000, 0.8660254037844387076, 1.000000000000000000, 0.8660254037844387076, 1.000000000000000000, 0.8660254037844387076, 1.000000000000000000, 0.8660254037844387076, 1.000000000000000000, 0.8660254037844387076, 1.000000000000000000, 0.8660254037844387076, 1.000000000000000000, 0.8660254037844387076, 1.000000000000000000, 0.8660254037844387076, 1.000000000000000000, 0.8660254037844387076, 1.000000000000000000, 0.8660254037844387076, 1.000000000000000000, 0.8660254037844387076, 1.000000000000000000, 0.8660254037844387076, 1.000000000000000000, 0.8660254037844387076, 1.000000000000000000, 0.8660254037844387076, 1.000000000000000000, 0.8660254037844387076, 1.000000000000000000, 0.8660254037844387076, 1.000000000000000000, 0.8660254037844387076, 1.000000000000000000, 0.8660254037844387076, 1.000000000000000000, 0.8660254037844387076, 1.000000000000000000, 0.8660254037844387076, 1.000000000000000000, 0.8660254037844387076, 1.000000000000000000, 0.8660254037844387076, 1.000000000000000000, 0.8660254037844387076, 1.000000000000000000, 0.8660254037844387076, 1.000000000000000000, 0.8660254037844387076, 1.000000000000000000, 0.8660254037844387076, 1.000000000000000000, 0.8957441496011320226, 0.9537471549767242429 ) ) 
 REPRESENTATION_ITEM ( '' )  );
#10717=CARTESIAN_POINT ( 'NONE',  ( 25.02395329184966144, -3.464101615137757051, 164.8362760637381541 ) ) ;
#10721=CARTESIAN_POINT ( 'NONE',  ( 15.24356964374999990, 3.323476615752268604, -2.090624999385484628 ) ) ;
#10730=LINE ( 'NONE', #7897, #11981 ) ;
#10731=( BOUNDED_CURVE ( )  B_SPLINE_CURVE ( 2, ( #2323, #36810, #34160, #13894, #16554, #13011, #22613 ),
 .UNSPECIFIED., .F., .F. ) 
 B_SPLINE_CURVE_WITH_KNOTS ( ( 3, 2, 2, 3 ),
 ( 0.02173913043478229237, 0.02898550724637658296, 0.03623188405797087008, 0.04347826086956516067 ),
 .UNSPECIFIED. ) 
 CURVE ( )  GEOMETRIC_REPRESENTATION_ITEM ( )  RATIONAL_B_SPLINE_CURVE ( ( 1.000000000000005773, 0.8660254037844328234, 1.000000000000000000, 0.8660254037844387076, 1.000000000000000000, 0.8660254037844397068, 0.9999999999999990008 ) ) 
 REPRESENTATION_ITEM ( '' )  );
#10732=CARTESIAN_POINT ( 'NONE',  ( 24.70858993122118363, 3.604726614523240613, 164.0263046051175024 ) ) ;
#10737=CARTESIAN_POINT ( 'NONE',  ( 18.00000000000000355, -5.196152422706632912, -3.525000000000000355 ) ) ;
#10747=CARTESIAN_POINT ( 'NONE',  ( 26.99999999999999645, 3.464101615137755275, -2.887499999999991296 ) ) ;
#10748=CARTESIAN_POINT ( 'NONE',  ( 25.05010001456683710, 0.000000000000000000, 165.1351344719413419 ) ) ;
#10749=CARTESIAN_POINT ( 'NONE',  ( 36.85406125198851157, -3.604726614523238837, 159.5758215996624187 ) ) ;
#10751=CARTESIAN_POINT ( 'NONE',  ( 28.30384396178233075, -5.407089921784859143, 169.3017823552670507 ) ) ;
#10754=EDGE_CURVE ( 'NONE', #22746, #29322, #9500, .T. ) ;
#10757=ORIENTED_EDGE ( 'NONE', *, *, #18561, .T. ) ;
#10762=CARTESIAN_POINT ( 'NONE',  ( 26.75643035624999655, 3.323476615752271712, -8.540624999385476812 ) ) ;
#10771=( BOUNDED_CURVE ( )  B_SPLINE_CURVE ( 2, ( #3403, #26331, #31835, #32212, #9097, #34865, #23501 ),
 .UNSPECIFIED., .F., .F. ) 
 B_SPLINE_CURVE_WITH_KNOTS ( ( 3, 2, 2, 3 ),
 ( 0.8260869565217380250, 0.8333333333333321491, 0.8405797101449260511, 0.8478260869565201752 ),
 .UNSPECIFIED. ) 
 CURVE ( )  GEOMETRIC_REPRESENTATION_ITEM ( )  RATIONAL_B_SPLINE_CURVE ( ( 1.000000000000020428, 0.8660254037844181685, 1.000000000000000000, 0.8660254037844387076, 1.000000000000000000, 0.8660254037844674624, 0.9999999999999712452 ) ) 
 REPRESENTATION_ITEM ( '' )  );
#10774=CARTESIAN_POINT ( 'NONE',  ( 34.04199902021685631, 5.196152422706637353, 164.6495911966399888 ) ) ;
#10775=CARTESIAN_POINT ( 'NONE',  ( 33.79808337967844523, 5.407089921784857367, 160.4642985439555218 ) ) ;
#10778=CARTESIAN_POINT ( 'NONE',  ( 27.61379986294728184, -5.196152422706638241, 160.0172180905011032 ) ) ;
#10787=CARTESIAN_POINT ( 'NONE',  ( 24.83442103481310781, 0.000000000000000000, 165.4645607004874535 ) ) ;
#10789=CARTESIAN_POINT ( 'NONE',  ( 15.24356964374999990, 3.323476615752268604, -6.028124999385455318 ) ) ;
#10791=EDGE_CURVE ( 'NONE', #30939, #33575, #5629, .T. ) ;
#10792=CARTESIAN_POINT ( 'NONE',  ( 19.80074372294634344, 5.630122097104456991, -7.999999999999998224 ) ) ;
#10793=CARTESIAN_POINT ( 'NONE',  ( 25.44556919728430699, -3.464101615137761048, 169.6553679145326328 ) ) ;
#10799=VERTEX_POINT ( 'NONE', #36171 ) ;
#10804=CARTESIAN_POINT ( 'NONE',  ( 15.24356964375000167, -3.323476615752272600, -3.253124999385455407 ) ) ;
#10807=CARTESIAN_POINT ( 'NONE',  ( 18.12178482187500350, -4.985214923628407568, -2.878124999385472726 ) ) ;
#10832=CARTESIAN_POINT ( 'NONE',  ( 24.70692427760507570, 0.000000000000000000, 161.2126178494294493 ) ) ;
#10838=CARTESIAN_POINT ( 'NONE',  ( 23.99999999999999645, 5.196152422706631135, -9.599999999999997868 ) ) ;
#10839=ORIENTED_EDGE ( 'NONE', *, *, #1006, .T. ) ;
#10844=CARTESIAN_POINT ( 'NONE',  ( 26.75643035624999655, -3.323476615752267715, -5.915624999385464378 ) ) ;
#10850=CARTESIAN_POINT ( 'NONE',  ( 37.56329110859752518, 7.646167579472024665E-16, 167.6823559553839971 ) ) ;
#10856=EDGE_CURVE ( 'NONE', #18997, #30939, #13256, .T. ) ;
#10868=CARTESIAN_POINT ( 'NONE',  ( 21.00000000000000355, 0.000000000000000000, 50.00000000000001421 ) ) ;
#10874=CARTESIAN_POINT ( 'NONE',  ( 27.65301994718372569, -5.196152422706638241, 160.4655057046423678 ) ) ;
#10886=CARTESIAN_POINT ( 'NONE',  ( 27.58480908411420529, 5.407089921784856479, 161.0831760960101349 ) ) ;
#10887=CARTESIAN_POINT ( 'NONE',  ( 26.75643035624999655, 3.323476615752271712, -0.4406249993854897129 ) ) ;
#10890=ORIENTED_EDGE ( 'NONE', *, *, #24524, .T. ) ;
#10893=CARTESIAN_POINT ( 'NONE',  ( 21.00000000000000000, 6.928203230275506996, -4.556249998770971921 ) ) ;
#10894=CARTESIAN_POINT ( 'NONE',  ( 26.75643035624999655, 7.049594010296217766E-16, -2.615624999385474325 ) ) ;
#10904=CARTESIAN_POINT ( 'NONE',  ( 37.06980319883564334, -3.464101615137751278, 164.8364115837626400 ) ) ;
#10908=CARTESIAN_POINT ( 'NONE',  ( 26.75643035624999655, -3.323476615752267271, -1.415624999385507232 ) ) ;
#10917=CARTESIAN_POINT ( 'NONE',  ( 37.25279877505902704, 3.604726614523243278, 164.1334123434321270 ) ) ;
#10923=CARTESIAN_POINT ( 'NONE',  ( 36.59262550718515428, 7.347880794884125653E-16, 159.3822456104860237 ) ) ;
#10932=ORIENTED_EDGE ( 'NONE', *, *, #30455, .F. ) ;
#10933=CARTESIAN_POINT ( 'NONE',  ( 15.00000000000000000, 3.464101615137752166, -1.837499999999979927 ) ) ;
#10936=CARTESIAN_POINT ( 'NONE',  ( 30.68654372136677466, 7.209453229046482114, 160.7177013682151596 ) ) ;
#10938=CARTESIAN_POINT ( 'NONE',  ( 31.37779770603408380, -7.209453229046475009, 168.6187705674553285 ) ) ;
#10948=CARTESIAN_POINT ( 'NONE',  ( 15.24356964374999990, 3.323476615752268604, -10.19062499938547184 ) ) ;
#10953=CARTESIAN_POINT ( 'NONE',  ( 25.12527184268644476, 3.464101615137619383, 165.9943523990454821 ) ) ;
#10961=CARTESIAN_POINT ( 'NONE',  ( 24.60236886974748316, -3.604726614523240613, 162.8121923168181695 ) ) ;
#10972=ORIENTED_EDGE ( 'NONE', *, *, #9183, .F. ) ;
#10974=CARTESIAN_POINT ( 'NONE',  ( 30.71105627401454896, -7.209453229046475009, 160.9978811270534891 ) ) ;
#10975=CARTESIAN_POINT ( 'NONE',  ( 18.12178482187500350, -4.985214923628407568, -6.365624999385477878 ) ) ;
#10977=CARTESIAN_POINT ( 'NONE',  ( 34.32918868704696536, -5.407089921784861808, 166.5348599854521296 ) ) ;
#10978=CARTESIAN_POINT ( 'NONE',  ( 28.22824784931821895, 5.196152422706636465, 167.0403907120479232 ) ) ;
#10985=VERTEX_POINT ( 'NONE', #18582 ) ;
#10987=CARTESIAN_POINT ( 'NONE',  ( 17.00000000000000000, 4.898587196589406912E-16, 50.17464377163448574 ) ) ;
#10988=CARTESIAN_POINT ( 'NONE',  ( 21.00000000000000000, -6.646953231504538984, -3.178124999385461003 ) ) ;
#10992=CARTESIAN_POINT ( 'NONE',  ( 18.12178482187500350, -4.985214923628407568, -1.978124999385488803 ) ) ;
#11020=DIRECTION ( 'NONE',  ( 0.000000000000000000, 0.000000000000000000, 1.000000000000000000 ) ) ;
#11021=CARTESIAN_POINT ( 'NONE',  ( 15.02283181144952628, 7.347880794884122694E-16, 50.52293445648592751 ) ) ;
#11025=CARTESIAN_POINT ( 'NONE',  ( 21.00000000000000000, -6.928203230275506996, -8.887499999999988631 ) ) ;
#11030=CARTESIAN_POINT ( 'NONE',  ( 21.00000000000000000, 6.646953231504538984, -8.015624999385487115 ) ) ;
#11037=CARTESIAN_POINT ( 'NONE',  ( 25.17923094205850276, 3.604726614523240613, 169.4057559748129336 ) ) ;
#11045=CARTESIAN_POINT ( 'NONE',  ( 18.00000000000000000, 5.196152422706630247, -1.368749998770957266 ) ) ;
#11053=( BOUNDED_CURVE ( )  B_SPLINE_CURVE ( 2, ( #8373, #26349, #17463, #3042, #16907, #3230, #6067 ),
 .UNSPECIFIED., .F., .F. ) 
 B_SPLINE_CURVE_WITH_KNOTS ( ( 3, 2, 2, 3 ),
 ( 0.4999999999999990008, 0.5072463768115932359, 0.5144927536231874710, 0.5217391304347817060 ),
 .UNSPECIFIED. ) 
 CURVE ( )  GEOMETRIC_REPRESENTATION_ITEM ( )  RATIONAL_B_SPLINE_CURVE ( ( 1.000000000000018430, 0.8660254037844202779, 1.000000000000000000, 0.8660254037844387076, 1.000000000000000000, 0.8660254037844551389, 0.9999999999999835687 ) ) 
 REPRESENTATION_ITEM ( '' )  );
#11060=CARTESIAN_POINT ( 'NONE',  ( 28.27727295472088542, 5.196152422706630247, 167.6007502309489041 ) ) ;
#11067=ORIENTED_EDGE ( 'NONE', *, *, #15675, .F. ) ;
#11073=CARTESIAN_POINT ( 'NONE',  ( 33.90267027097563357, -5.407089921784855591, 161.6597321816656176 ) ) ;
#11080=CARTESIAN_POINT ( 'NONE',  ( 21.00000000000000000, 6.928203230275506996, -4.106249998770976184 ) ) ;
#11081=CARTESIAN_POINT ( 'NONE',  ( 18.12178482187499640, 4.985214923628404904, -2.915624999385468819 ) ) ;
#11083=CARTESIAN_POINT ( 'NONE',  ( 37.37375885156122024, -3.464101615137610057, 168.3106405921332680 ) ) ;
#11084=CARTESIAN_POINT ( 'NONE',  ( 18.12178482187499640, 4.985214923628404904, -10.11562499938548143 ) ) ;
#11093=CARTESIAN_POINT ( 'NONE',  ( 25.02068495149662297, 0.000000000000000000, 164.7989187625597367 ) ) ;
#11097=EDGE_CURVE ( 'NONE', #941, #9824, #31740, .T. ) ;
#11098=CARTESIAN_POINT ( 'NONE',  ( 23.87821517812500005, -4.985214923628404016, -5.053124999385483207 ) ) ;
#11107=CARTESIAN_POINT ( 'NONE',  ( 37.13187018199665346, 7.646167579472024665E-16, 162.7511921998298590 ) ) ;
#11111=LINE ( 'NONE', #17178, #1931 ) ;
#11119=ORIENTED_EDGE ( 'NONE', *, *, #17590, .T. ) ;
#11120=CARTESIAN_POINT ( 'NONE',  ( 18.00000000000000355, -5.196152422706632912, -3.525000000000000355 ) ) ;
#11122=DIRECTION ( 'NONE',  ( 0.08715574274765150453, 0.000000000000000000, 0.9961946980917461003 ) ) ;
#11123=CARTESIAN_POINT ( 'NONE',  ( 27.61912665782109499, 5.407089921784862696, 161.4754277583837734 ) ) ;
#11125=CARTESIAN_POINT ( 'NONE',  ( 28.25155051613373658, 5.407089921784856479, 168.7040655364119743 ) ) ;
#11130=ORIENTED_EDGE ( 'NONE', *, *, #4037, .T. ) ;
#11133=CARTESIAN_POINT ( 'NONE',  ( 27.76741185964712244, 5.196152422706630247, 161.7730112471121799 ) ) ;
#11136=CARTESIAN_POINT ( 'NONE',  ( 15.24356964375000167, -3.323476615752272600, -7.865624999385466332 ) ) ;
#11139=CARTESIAN_POINT ( 'NONE',  ( 37.34761212884377812, 7.347880794884117764E-16, 168.0117821839301087 ) ) ;
#11140=CARTESIAN_POINT ( 'NONE',  ( 27.65834674205753529, 5.407089921784862696, 161.9237153725250664 ) ) ;
#11142=CARTESIAN_POINT ( 'NONE',  ( 25.12854018303972126, 0.000000000000000000, 166.0317097002238995 ) ) ;
#11145=VECTOR ( 'NONE', #1603, 1000.000000000000000 ) ;
#11152=CARTESIAN_POINT ( 'NONE',  ( 33.71964321120555752, 5.407089921784857367, 159.5677233156729642 ) ) ;
#11153=CARTESIAN_POINT ( 'NONE',  ( 31.18414854017020232, 6.928203230275506996, 166.4053504732449369 ) ) ;
#11162=CARTESIAN_POINT ( 'NONE',  ( 33.90267027097563357, -5.407089921784855591, 161.6597321816656176 ) ) ;
#11163=CARTESIAN_POINT ( 'NONE',  ( 26.75643035624999655, 3.323476615752271712, -7.078124999385466687 ) ) ;
#11165=CARTESIAN_POINT ( 'NONE',  ( 37.40967911200478824, 3.604726614523243278, 165.9265627999972992 ) ) ;
#11166=CARTESIAN_POINT ( 'NONE',  ( 31.15473347688575956, -6.928203230275514990, 166.0691347614145741 ) ) ;
#11173=ORIENTED_EDGE ( 'NONE', *, *, #19236, .F. ) ;
#11178=CARTESIAN_POINT ( 'NONE',  ( 15.24356964375000167, -3.323476615752272600, -2.465624999385486404 ) ) ;
#11200=CARTESIAN_POINT ( 'NONE',  ( 25.18740179294109183, 0.000000000000000000, 169.4991492277590339 ) ) ;
#11209=CARTESIAN_POINT ( 'NONE',  ( 15.00000000000000178, -3.464101615137757051, -9.412499999999978328 ) ) ;
#11210=EDGE_LOOP ( 'NONE', ( #8462, #32222, #13790, #13367 ) ) ;
#11215=CARTESIAN_POINT ( 'NONE',  ( 23.87821517812499650, 4.985214923628404904, -9.853124999385482141 ) ) ;
#11221=CARTESIAN_POINT ( 'NONE',  ( 24.90469035240339934, 3.604726614523240613, 166.2677426758239108 ) ) ;
#11226=CARTESIAN_POINT ( 'NONE',  ( 15.00000000000000000, 0.000000000000000000, -6.243749998770947940 ) ) ;
#11229=CARTESIAN_POINT ( 'NONE',  ( 34.54326498017087488, 5.407089921784857367, 168.9817632126399758 ) ) ;
#11231=DIRECTION ( 'NONE',  ( 0.08715574274765150453, 0.000000000000000000, 0.9961946980917461003 ) ) ;
#11232=DIRECTION ( 'NONE',  ( 0.000000000000000000, 0.000000000000000000, 1.000000000000000000 ) ) ;
#11242=EDGE_CURVE ( 'NONE', #16861, #25852, #35610, .T. ) ;
#11245=CARTESIAN_POINT ( 'NONE',  ( 15.24356964374999990, 0.000000000000000000, -0.2531249993854844949 ) ) ;
#11261=CARTESIAN_POINT ( 'NONE',  ( 24.56314878551103575, -3.604726614523240613, 162.3639047026768765 ) ) ;
#11263=CYLINDRICAL_SURFACE ( 'NONE', #8108, 5.999999999999994671 ) ;
#11268=CARTESIAN_POINT ( 'NONE',  ( 24.00000000000000000, -5.196152422706629359, -6.543749998770942433 ) ) ;
#11269=CARTESIAN_POINT ( 'NONE',  ( 23.87821517812499650, 4.985214923628404904, -1.640624999385470462 ) ) ;
#11270=CARTESIAN_POINT ( 'NONE',  ( 24.62848410913218800, 0.000000000000000000, 160.3160426211468348 ) ) ;
#11271=CARTESIAN_POINT ( 'NONE',  ( 34.38190641693269356, -5.196152422706635576, 168.5347505191977859 ) ) ;
#11279=CARTESIAN_POINT ( 'NONE',  ( 31.00765816110621031, -6.928203230275506996, 164.3880562096091182 ) ) ;
#11284=( BOUNDED_CURVE ( )  B_SPLINE_CURVE ( 2, ( #3068, #31325, #11045, #16931, #34719, #20338, #28473 ),
 .UNSPECIFIED., .F., .F. ) 
 B_SPLINE_CURVE_WITH_KNOTS ( ( 3, 2, 2, 3 ),
 ( 0.08695652173913158423, 0.09420289855072500051, 0.1014492753623184029, 0.1086956521739118053 ),
 .UNSPECIFIED. ) 
 CURVE ( )  GEOMETRIC_REPRESENTATION_ITEM ( )  RATIONAL_B_SPLINE_CURVE ( ( 0.9999999999999786837, 0.8660254037844600239, 1.000000000000000000, 0.8660254037844387076, 1.000000000000000000, 0.8660254037844615782, 0.9999999999999771294 ) ) 
 REPRESENTATION_ITEM ( '' )  );
#11285=CARTESIAN_POINT ( 'NONE',  ( 26.75643035624999655, 3.323476615752271268, -4.040624999385488358 ) ) ;
#11286=CARTESIAN_POINT ( 'NONE',  ( 15.00000000000000000, 0.000000000000000000, -1.799999999999996048 ) ) ;
#11294=CARTESIAN_POINT ( 'NONE',  ( 27.78908035617901717, -5.407089921784865361, 163.4180074196626720 ) ) ;
#11303=CARTESIAN_POINT ( 'NONE',  ( 15.00000000000000355, 7.347880794884112834E-16, -8.000000000000000000 ) ) ;
#11307=CARTESIAN_POINT ( 'NONE',  ( 15.00000000000000000, 3.464101615137752166, -4.537499999999986322 ) ) ;
#11309=CARTESIAN_POINT ( 'NONE',  ( 36.81810950810510974, 7.646167579472024665E-16, 159.1648912866995715 ) ) ;
#11311=CARTESIAN_POINT ( 'NONE',  ( 28.21233043189729273, 5.407089921784856479, 168.2557779222707097 ) ) ;
#11321=CARTESIAN_POINT ( 'NONE',  ( 26.75643035624999655, 3.323476615752271712, -8.090624999385481075 ) ) ;
#11326=CARTESIAN_POINT ( 'NONE',  ( 24.55497793462844669, 0.000000000000000000, 162.2705114497308045 ) ) ;
#11329=FILL_AREA_STYLE ('',( #25730 ) ) ;
#11336=CARTESIAN_POINT ( 'NONE',  ( 31.30180879287953388, 6.928203230275506996, 167.7502133156687876 ) ) ;
#11338=CARTESIAN_POINT ( 'NONE',  ( 36.86223210287109708, 7.646167579472015790E-16, 159.6692148526084907 ) ) ;
#11339=CARTESIAN_POINT ( 'NONE',  ( 15.00000000000000000, 0.000000000000000000, -3.543749998770939769 ) ) ;
#11349=CARTESIAN_POINT ( 'NONE',  ( 37.01911243981686539, 7.646167579472015790E-16, 161.4623653091736628 ) ) ;
#11350=CARTESIAN_POINT ( 'NONE',  ( 26.75643035624999655, 7.049594010296217766E-16, -7.565624999385455851 ) ) ;
#11353=CARTESIAN_POINT ( 'NONE',  ( 31.25523494279520165, -7.209453229046482114, 167.2178717732638233 ) ) ;
#11354=CARTESIAN_POINT ( 'NONE',  ( 25.12527184268668634, 3.464101615137757051, 165.9943523990454537 ) ) ;
#11355=DIRECTION ( 'NONE',  ( 0.000000000000000000, 0.000000000000000000, 1.000000000000000000 ) ) ;
#11367=CARTESIAN_POINT ( 'NONE',  ( 23.87821517812500005, -4.985214923628404016, -1.003124999385485161 ) ) ;
#11372=AXIS2_PLACEMENT_3D ( 'NONE', #27366, #12777, #30024 ) ;
#11386=CARTESIAN_POINT ( 'NONE',  ( 31.37779770603408380, -7.209453229046475009, 168.6187705674553285 ) ) ;
#11388=CARTESIAN_POINT ( 'NONE',  ( 26.75643035624999655, 7.049594010296217766E-16, -0.3656249993854721048 ) ) ;
#11390=DIRECTION ( 'NONE',  ( 1.000000000000000000, 0.000000000000000000, 0.000000000000000000 ) ) ;
#11403=CARTESIAN_POINT ( 'NONE',  ( 18.12178482187499640, 4.985214923628404904, -0.2156249993854608693 ) ) ;
#11405=ORIENTED_EDGE ( 'NONE', *, *, #30351, .T. ) ;
#11408=CARTESIAN_POINT ( 'NONE',  ( 24.62848410913218800, 0.000000000000000000, 160.3160426211468348 ) ) ;
#11410=CARTESIAN_POINT ( 'NONE',  ( 28.14206111430700474, -5.407089921784865361, 167.4525959469342524 ) ) ;
#11417=CARTESIAN_POINT ( 'NONE',  ( 34.49097153452227360, -5.407089921784855591, 168.3840463937848995 ) ) ;
#11421=CARTESIAN_POINT ( 'NONE',  ( 26.99999999999952038, -3.464101615138027057, -7.012500000000017941 ) ) ;
#11431=CARTESIAN_POINT ( 'NONE',  ( 37.22014685496823461, 7.347880794884125653E-16, 166.5548474367465985 ) ) ;
#11432=CARTESIAN_POINT ( 'NONE',  ( 36.72009078106068358, 7.347880794884117764E-16, 160.8391803576695622 ) ) ;
#11438=ORIENTED_EDGE ( 'NONE', *, *, #27064, .T. ) ;
#11445=CARTESIAN_POINT ( 'NONE',  ( 24.47817193633207822, 3.604726614523236616, 161.3926148720374556 ) ) ;
#11446=CARTESIAN_POINT ( 'NONE',  ( 21.00000000000000000, 6.646953231504538984, -1.715624999385482852 ) ) ;
#11449=ORIENTED_EDGE ( 'NONE', *, *, #22130, .F. ) ;
#11452=CARTESIAN_POINT ( 'NONE',  ( 26.99999999999999645, -3.464101615137751278, -6.956249998770937637 ) ) ;
#11453=CARTESIAN_POINT ( 'NONE',  ( 18.12178482187499640, 4.985214923628404904, -3.815624999385480720 ) ) ;
#11459=CYLINDRICAL_SURFACE ( 'NONE', #23874, 6.000000000000001776 ) ;
#11462=CARTESIAN_POINT ( 'NONE',  ( 24.90302469878729141, 0.000000000000000000, 163.4540559201358576 ) ) ;
#11466=CARTESIAN_POINT ( 'NONE',  ( 15.24356964375000167, -3.323476615752272600, -4.265624999385501326 ) ) ;
#11471=CARTESIAN_POINT ( 'NONE',  ( 25.13834520420595098, 0.000000000000000000, 166.1437816049835874 ) ) ;
#11475=CARTESIAN_POINT ( 'NONE',  ( 24.67263818733777470, 0.000000000000000000, 163.6153742921546836 ) ) ;
#11477=EDGE_CURVE ( 'NONE', #10799, #31903, #13375, .T. ) ;
#11479=( BOUNDED_CURVE ( )  B_SPLINE_CURVE ( 2, ( #18886, #1423, #12804, #35918, #15469 ),
 .UNSPECIFIED., .F., .F. ) 
 B_SPLINE_CURVE_WITH_KNOTS ( ( 3, 2, 3 ),
 ( 0.9565217391304360328, 0.9637681159420292687, 0.9662082944262200268 ),
 .UNSPECIFIED. ) 
 CURVE ( )  GEOMETRIC_REPRESENTATION_ITEM ( )  RATIONAL_B_SPLINE_CURVE ( ( 0.9999999999999774625, 0.8660254037844612451, 1.000000000000000000, 0.9548847740583508159, 0.9401541683247176540 ) ) 
 REPRESENTATION_ITEM ( '' )  );
#11489=CARTESIAN_POINT ( 'NONE',  ( 21.00000000000000000, 6.928203230275506996, -5.062500000000007994 ) ) ;
#11491=CARTESIAN_POINT ( 'NONE',  ( 27.51453976652391376, -5.407089921784865361, 160.2799941206736776 ) ) ;
#11493=CARTESIAN_POINT ( 'NONE',  ( 25.22662187717753568, 0.000000000000000000, 169.9474368419002985 ) ) ;
#11495=CARTESIAN_POINT ( 'NONE',  ( 21.00000000000000355, 0.000000000000000000, 50.00000000000001421 ) ) ;
#11499=CARTESIAN_POINT ( 'NONE',  ( 36.60243052835136268, 7.347880794884117764E-16, 159.4943175152456831 ) ) ;
#11502=VECTOR ( 'NONE', #29211, 1000.000000000000000 ) ;
#11504=CARTESIAN_POINT ( 'NONE',  ( 37.02077809343345649, -3.464101615137479495, 164.2760520648616875 ) ) ;
#11508=CARTESIAN_POINT ( 'NONE',  ( 30.70615376348499836, -7.209453229046482114, 160.9418451752858346 ) ) ;
#11520=CARTESIAN_POINT ( 'NONE',  ( 25.18576762276457259, -3.604726614523244610, 169.4804705771697968 ) ) ;
#11521=CARTESIAN_POINT ( 'NONE',  ( 26.99999999999999645, 7.347880794884117764E-16, -2.418749998770952647 ) ) ;
#11524=AXIS2_PLACEMENT_3D ( 'NONE', #32416, #6460, #15556 ) ;
#11531=CARTESIAN_POINT ( 'NONE',  ( 33.87652354815133293, 5.407089921784857367, 161.3608737722381079 ) ) ;
#11532=CARTESIAN_POINT ( 'NONE',  ( 23.87821517812499650, 4.985214923628404904, -7.490624999385464555 ) ) ;
#11534=CARTESIAN_POINT ( 'NONE',  ( 37.44563085588819717, 7.646167579472024665E-16, 166.3374931129601464 ) ) ;
#11535=CARTESIAN_POINT ( 'NONE',  ( 37.06653485837549766, 3.464101615137759271, 164.7990542813598722 ) ) ;
#11536=CARTESIAN_POINT ( 'NONE',  ( 18.00000000000000000, 5.196152422706630247, -0.07499999999999173994 ) ) ;
#11547=CARTESIAN_POINT ( 'NONE',  ( 23.87821517812499650, 4.985214923628404904, -1.753124999385485827 ) ) ;
#11558=EDGE_CURVE ( 'NONE', #34009, #23156, #36778, .T. ) ;
#11561=VECTOR ( 'NONE', #3207, 1000.000000000000000 ) ;
#11568=CARTESIAN_POINT ( 'NONE',  ( 27.00000000000007816, 3.464101615137709533, -4.631249998770966769 ) ) ;
#11570=VERTEX_POINT ( 'NONE', #23456 ) ;
#11572=CARTESIAN_POINT ( 'NONE',  ( 21.00000000000000000, 6.646953231504538984, -0.7031249993854685743 ) ) ;
#11573=CARTESIAN_POINT ( 'NONE',  ( 15.00000000000047606, 3.464101615138028389, -4.987500000000019362 ) ) ;
#11577=CARTESIAN_POINT ( 'NONE',  ( 34.23809944139907202, 5.196152422706637353, 166.8910292673464539 ) ) ;
#11581=VERTEX_POINT ( 'NONE', #694 ) ;
#11585=CARTESIAN_POINT ( 'NONE',  ( 26.75643035624999655, -3.323476615752267715, -8.615624999385470772 ) ) ;
#11590=CARTESIAN_POINT ( 'NONE',  ( 37.40641077165175687, 7.646167579472024665E-16, 165.8892054988188534 ) ) ;
#11597=CARTESIAN_POINT ( 'NONE',  ( 34.45175145028584041, -5.407089921784855591, 167.9357587796436064 ) ) ;
#11600=CARTESIAN_POINT ( 'NONE',  ( 27.00000000000013500, 3.464101615137676227, -0.5812499987709733862 ) ) ;
#11611=DIRECTION ( 'NONE',  ( 0.08715574274765143514, 0.000000000000000000, 0.9961946980917462113 ) ) ;
#11617=CARTESIAN_POINT ( 'NONE',  ( 15.00000000000000355, 7.347880794884112834E-16, -8.000000000000000000 ) ) ;
#11626=CARTESIAN_POINT ( 'NONE',  ( 21.00000000000000000, -6.646953231504538984, -1.940624999385496929 ) ) ;
#11629=ORIENTED_EDGE ( 'NONE', *, *, #18769, .F. ) ;
#11632=CARTESIAN_POINT ( 'NONE',  ( 18.00000000000000355, -5.196152422706632912, -7.968749998770952025 ) ) ;
#11633=CARTESIAN_POINT ( 'NONE',  ( 26.75643035624999655, 7.049594010296217766E-16, -3.965624999385464200 ) ) ;
#11640=CARTESIAN_POINT ( 'NONE',  ( 36.71682244070765933, -3.464101615137751278, 160.8018230564910880 ) ) ;
#11644=CARTESIAN_POINT ( 'NONE',  ( 15.24356964374999990, 3.323476615752268604, -3.890624999385467575 ) ) ;
#11645=CARTESIAN_POINT ( 'NONE',  ( 23.99999999999999645, 5.196152422706631135, -0.5999999999999894307 ) ) ;
#11648=ORIENTED_EDGE ( 'NONE', *, *, #33263, .F. ) ;
#11652=CARTESIAN_POINT ( 'NONE',  ( 20.99999999999999645, 0.000000000000000000, -8.000000000000000000 ) ) ;
#11653=CARTESIAN_POINT ( 'NONE',  ( 30.84342405831255007, 7.209453229046482114, 162.5108518247803318 ) ) ;
#11657=CYLINDRICAL_SURFACE ( 'NONE', #37013, 5.999999999999994671 ) ;
#11664=CARTESIAN_POINT ( 'NONE',  ( 25.00000000000004263, 0.000000000000000000, 49.82535622836640954 ) ) ;
#11668=CARTESIAN_POINT ( 'NONE',  ( 18.00000000000000000, 5.196152422706630247, -5.475000000000007638 ) ) ;
#11673=CARTESIAN_POINT ( 'NONE',  ( 25.07300988058480229, -3.604726614523240613, 168.1916436865136291 ) ) ;
#11679=ORIENTED_EDGE ( 'NONE', *, *, #33263, .T. ) ;
#11681=CARTESIAN_POINT ( 'NONE',  ( 33.60730975337005333, -5.196152422706629359, 159.6810701411317552 ) ) ;
#11684=CARTESIAN_POINT ( 'NONE',  ( 18.12178482187499640, 4.985214923628404904, -5.615624999385476990 ) ) ;
#11691=CARTESIAN_POINT ( 'NONE',  ( 24.43731768191911513, 0.000000000000000000, 160.9256486073069539 ) ) ;
#11698=EDGE_LOOP ( 'NONE', ( #11770, #12025, #9170, #298 ) ) ;
#11702=CARTESIAN_POINT ( 'NONE',  ( 25.47963170482115913, 3.634172111495134416, -8.000000000000000000 ) ) ;
#11703=CARTESIAN_POINT ( 'NONE',  ( 31.37289519550453321, -7.209453229046482114, 168.5627346156876740 ) ) ;
#11704=CARTESIAN_POINT ( 'NONE',  ( 18.00000000000000000, 5.196152422706630247, -2.718749998770947585 ) ) ;
#11714=CARTESIAN_POINT ( 'NONE',  ( 24.55661210480496592, 3.604726614523236616, 162.2891901003200132 ) ) ;
#11715=CARTESIAN_POINT ( 'NONE',  ( 15.24356964374999990, 0.000000000000000000, -8.240624999385465443 ) ) ;
#11718=CARTESIAN_POINT ( 'NONE',  ( 24.98639886122932197, 0.000000000000000000, 167.2016752052849426 ) ) ;
#11719=CARTESIAN_POINT ( 'NONE',  ( 37.26263527955770627, 3.464101615137759271, 167.0404923520662805 ) ) ;
#11720=CYLINDRICAL_SURFACE ( 'NONE', #32586, 5.999999999999994671 ) ;
#11723=EDGE_CURVE ( 'NONE', #4359, #7912, #13024, .T. ) ;
#11731=EDGE_CURVE ( 'NONE', #30158, #31903, #24580, .T. ) ;
#11733=CARTESIAN_POINT ( 'NONE',  ( 18.12178482187500350, -4.985214923628407568, -3.328124999385479121 ) ) ;
#11751=CARTESIAN_POINT ( 'NONE',  ( 24.97165984609394940, 0.000000000000000000, 164.2385592436587558 ) ) ;
#11754=CARTESIAN_POINT ( 'NONE',  ( 36.83775103377001869, 7.347880794884117764E-16, 162.1840432000934129 ) ) ;
#11757=CARTESIAN_POINT ( 'NONE',  ( 25.22335353682449721, 3.604726614523236616, 169.9100795407219096 ) ) ;
#11758=AXIS2_PLACEMENT_3D ( 'NONE', #14330, #19479, #25884 ) ;
#11760=( BOUNDED_CURVE ( )  B_SPLINE_CURVE ( 2, ( #25328, #36877, #22498, #5234, #16810, #280, #11846 ),
 .UNSPECIFIED., .F., .F. ) 
 B_SPLINE_CURVE_WITH_KNOTS ( ( 3, 2, 2, 3 ),
 ( 0.8043478260869549867, 0.8115942028985493328, 0.8188405797101435679, 0.8260869565217379140 ),
 .UNSPECIFIED. ) 
 CURVE ( )  GEOMETRIC_REPRESENTATION_ITEM ( )  RATIONAL_B_SPLINE_CURVE ( ( 1.000000000000028644, 0.8660254037844099528, 1.000000000000000000, 0.8660254037844387076, 1.000000000000000000, 0.8660254037844612451, 0.9999999999999774625 ) ) 
 REPRESENTATION_ITEM ( '' )  );
#11762=CARTESIAN_POINT ( 'NONE',  ( 20.99999999999999645, 0.000000000000000000, -8.000000000000000000 ) ) ;
#11767=CARTESIAN_POINT ( 'NONE',  ( 28.26746793355466281, 5.196152422706636465, 167.4886783261892162 ) ) ;
#11769=CARTESIAN_POINT ( 'NONE',  ( 28.16288104225748512, -5.196152422706638241, 166.2932446884790920 ) ) ;
#11770=ORIENTED_EDGE ( 'NONE', *, *, #6322, .F. ) ;
#11775=CARTESIAN_POINT ( 'NONE',  ( 20.00041297495057080, 5.668978411116884608, -10.25260147226209995 ) ) ;
#11780=CARTESIAN_POINT ( 'NONE',  ( 28.12898775289485442, 5.407089921784862696, 167.3031667422204691 ) ) ;
#11786=CARTESIAN_POINT ( 'NONE',  ( 37.64663378759995283, 7.646167579472015790E-16, 168.6349671354342092 ) ) ;
#11800=CARTESIAN_POINT ( 'NONE',  ( 34.27405118538959528, -5.196152422706629359, 167.3019595815335947 ) ) ;
#11801=CARTESIAN_POINT ( 'NONE',  ( 14.99999999999965539, 3.464101615137553658, -4.031249998770945808 ) ) ;
#11802=EDGE_CURVE ( 'NONE', #11864, #15590, #3920, .T. ) ;
#11803=CARTESIAN_POINT ( 'NONE',  ( 37.19400013225076407, 3.464101615137916035, 166.2559890285434392 ) ) ;
#11807=VERTEX_POINT ( 'NONE', #15684 ) ;
#11813=CARTESIAN_POINT ( 'NONE',  ( 26.75643035624999655, 7.049594010296217766E-16, -2.728124999385489247 ) ) ;
#11817=VECTOR ( 'NONE', #33679, 1000.000000000000000 ) ;
#11820=CARTESIAN_POINT ( 'NONE',  ( 18.12178482187500350, -4.985214923628407568, -5.015624999385459581 ) ) ;
#11827=CARTESIAN_POINT ( 'NONE',  ( 24.89975635843425650, 3.464101615137752166, 163.4166986189574402 ) ) ;
#11831=CARTESIAN_POINT ( 'NONE',  ( 26.75643035624999655, 3.323476615752271268, -5.390624999385473792 ) ) ;
#11835=AXIS2_PLACEMENT_3D ( 'NONE', #13973, #11122, #24273 ) ;
#11841=CARTESIAN_POINT ( 'NONE',  ( 15.00000000000000000, 0.000000000000000000, -5.793749998770941545 ) ) ;
#11846=CARTESIAN_POINT ( 'NONE',  ( 24.70692427760507570, 0.000000000000000000, 161.2126178494294493 ) ) ;
#11855=CARTESIAN_POINT ( 'NONE',  ( 26.99999999999999645, 7.347880794884117764E-16, -3.824999999999994849 ) ) ;
#11856=CARTESIAN_POINT ( 'NONE',  ( 28.20210112649392542, -5.196152422706638241, 166.7415323026203851 ) ) ;
#11859=CARTESIAN_POINT ( 'NONE',  ( 24.99130137175887612, 0.000000000000000000, 167.2577111570525972 ) ) ;
#11864=VERTEX_POINT ( 'NONE', #27235 ) ;
#11867=CARTESIAN_POINT ( 'NONE',  ( 21.00000000000000355, 0.000000000000000000, 50.00000000000001421 ) ) ;
#11868=CARTESIAN_POINT ( 'NONE',  ( 21.00000000000000000, 6.646953231504538984, -6.103124999385481253 ) ) ;
#11875=CARTESIAN_POINT ( 'NONE',  ( 37.30512370425429935, -3.464101615137751278, 167.5261372686103982 ) ) ;
#11887=CARTESIAN_POINT ( 'NONE',  ( 37.33780710767756972, 7.347880794884125653E-16, 167.8997102791704492 ) ) ;
#11889=CARTESIAN_POINT ( 'NONE',  ( 24.40300010821222898, 0.000000000000000000, 160.5333969449332869 ) ) ;
#11890=CARTESIAN_POINT ( 'NONE',  ( 21.00000000000000000, -6.928203230275506996, -1.631249998770951004 ) ) ;
#11897=EDGE_CURVE ( 'NONE', #14950, #25042, #32959, .T. ) ;
#11899=FACE_OUTER_BOUND ( 'NONE', #36746, .T. ) ;
#11902=CARTESIAN_POINT ( 'NONE',  ( 36.86550044322413555, 3.604726614523238837, 159.7065721537869365 ) ) ;
#11903=CARTESIAN_POINT ( 'NONE',  ( 26.75643035624999655, -3.323476615752267715, -7.603124999385488358 ) ) ;
#11905=CARTESIAN_POINT ( 'NONE',  ( 27.98518077736123288, -5.407089921784865361, 165.6594454903691087 ) ) ;
#11906=CARTESIAN_POINT ( 'NONE',  ( 30.97824309782176044, 6.928203230275514990, 164.0518404977788407 ) ) ;
#11919=CARTESIAN_POINT ( 'NONE',  ( 23.87821517812499650, 4.985214923628404904, -3.103124999385475924 ) ) ;
#11930=DIRECTION ( 'NONE',  ( 0.9961946980917459893, 0.000000000000000000, -0.08715574274765348906 ) ) ;
#11931=CARTESIAN_POINT ( 'NONE',  ( 30.97824309782176755, 6.928203230275514990, 164.0518404977788123 ) ) ;
#11936=ADVANCED_FACE ( 'NONE', ( #13774 ), #30830, .T. ) ;
#11947=CARTESIAN_POINT ( 'NONE',  ( 26.75643035624999655, -3.323476615752267715, -1.303124999385484095 ) ) ;
#11955=ORIENTED_EDGE ( 'NONE', *, *, #28642, .T. ) ;
#11958=CARTESIAN_POINT ( 'NONE',  ( 18.12178482187499640, 4.985214923628404904, -8.878124999385478944 ) ) ;
#11960=EDGE_CURVE ( 'NONE', #29322, #23945, #4853, .T. ) ;
#11961=CARTESIAN_POINT ( 'NONE',  ( 25.40634911304790577, -3.464101615137787693, 169.2070803003913397 ) ) ;
#11965=CARTESIAN_POINT ( 'NONE',  ( 28.18128119854344860, -5.407089921784865361, 167.9008835610755455 ) ) ;
#11971=FACE_OUTER_BOUND ( 'NONE', #8079, .T. ) ;
#11972=EDGE_LOOP ( 'NONE', ( #31033, #31886, #961, #11119 ) ) ;
#11976=( BOUNDED_CURVE ( )  B_SPLINE_CURVE ( 2, ( #33401, #33215, #33024, #28079, #19012, #24867, #1368 ),
 .UNSPECIFIED., .F., .F. ) 
 B_SPLINE_CURVE_WITH_KNOTS ( ( 3, 2, 2, 3 ),
 ( 0.1956521739130434034, 0.2028985507246377218, 0.2101449275362319846, 0.2173913043478263030 ),
 .UNSPECIFIED. ) 
 CURVE ( )  GEOMETRIC_REPRESENTATION_ITEM ( )  RATIONAL_B_SPLINE_CURVE ( ( 1.000000000000001554, 0.8660254037844372643, 1.000000000000000000, 0.8660254037844387076, 1.000000000000000000, 0.8660254037844345998, 1.000000000000003997 ) ) 
 REPRESENTATION_ITEM ( '' )  );
#11977=PRODUCT ( 'extension pipe', 'extension pipe', '', ( #34626 ) ) ;
#11981=VECTOR ( 'NONE', #22304, 1000.000000000000000 ) ;
#11990=CARTESIAN_POINT ( 'NONE',  ( 28.43415329166666083, 5.196152422706630247, 169.3939006875140194 ) ) ;
#12000=CARTESIAN_POINT ( 'NONE',  ( 24.36051168362275021, 3.604726614523236616, 160.0477520296136049 ) ) ;
#12001=CARTESIAN_POINT ( 'NONE',  ( 21.00000000000000000, -6.646953231504538984, -3.290624999385483918 ) ) ;
#12006=CARTESIAN_POINT ( 'NONE',  ( 23.87821517812500005, -4.985214923628404016, -6.290624999385458160 ) ) ;
#12010=EDGE_CURVE ( 'NONE', #18510, #34425, #34225, .T. ) ;
#12015=CARTESIAN_POINT ( 'NONE',  ( 24.74614436184151955, 0.000000000000000000, 161.6609054635707423 ) ) ;
#12021=CARTESIAN_POINT ( 'NONE',  ( 15.24356964374999990, 0.000000000000000000, -7.003124999385490490 ) ) ;
#12025=ORIENTED_EDGE ( 'NONE', *, *, #22570, .T. ) ;
#12026=CARTESIAN_POINT ( 'NONE',  ( 37.15151170766156952, 7.347880794884117764E-16, 165.7703441132237003 ) ) ;
#12030=CARTESIAN_POINT ( 'NONE',  ( 30.62771359501211066, -7.209453229046482114, 160.0452699470032485 ) ) ;
#12038=CARTESIAN_POINT ( 'NONE',  ( 26.99999999999999645, 7.347880794884117764E-16, -7.818749998770941012 ) ) ;
#12042=CARTESIAN_POINT ( 'NONE',  ( 26.99999999999999645, 7.347880794884117764E-16, -6.975000000000008527 ) ) ;
#12046=CARTESIAN_POINT ( 'NONE',  ( 34.41253136604939300, -5.407089921784855591, 167.4874711655023418 ) ) ;
#12053=CARTESIAN_POINT ( 'NONE',  ( 26.99999999999946354, -3.464101615138058143, -3.356249998770978848 ) ) ;
#12055=CARTESIAN_POINT ( 'NONE',  ( 26.75643035624999655, 7.049594010296217766E-16, -5.765624999385460470 ) ) ;
#12058=CARTESIAN_POINT ( 'NONE',  ( 18.00000000000000355, -5.196152422706632912, -5.268749998770943854 ) ) ;
#12061=CYLINDRICAL_SURFACE ( 'NONE', #21000, 6.000000000000001776 ) ;
#12062=CARTESIAN_POINT ( 'NONE',  ( 25.41288579386105440, 0.000000000000000000, 169.2817949039725818 ) ) ;
#12074=CARTESIAN_POINT ( 'NONE',  ( 24.69183098274843502, 4.432317000257220307, -7.999999999999998224 ) ) ;
#12075=CARTESIAN_POINT ( 'NONE',  ( 25.06810737005524459, -3.604726614523244610, 168.1356077347459461 ) ) ;
#12076=CARTESIAN_POINT ( 'NONE',  ( 21.00000000000000000, -6.928203230275506996, -2.081249998770946963 ) ) ;
#12080=CARTESIAN_POINT ( 'NONE',  ( 21.00000000000000355, 0.000000000000000000, 50.00000000000001421 ) ) ;
#12087=CARTESIAN_POINT ( 'NONE',  ( 26.99999999999999645, -3.464101615137751278, -0.2625000000000108913 ) ) ;
#12089=CARTESIAN_POINT ( 'NONE',  ( 27.90674060888834518, -5.407089921784865361, 164.7628702620865226 ) ) ;
#12090=CARTESIAN_POINT ( 'NONE',  ( 36.86716609684025059, 7.347880794884125653E-16, 162.5202589094750181 ) ) ;
#12096=ORIENTED_EDGE ( 'NONE', *, *, #8355, .F. ) ;
#12101=CARTESIAN_POINT ( 'NONE',  ( 23.87821517812499650, 4.985214923628404904, -4.003124999385487826 ) ) ;
#12110=PLANE ( 'NONE',  #1878 ) ;
#12111=AXIS2_PLACEMENT_3D ( 'NONE', #5142, #4400, #16723 ) ;
#12115=CARTESIAN_POINT ( 'NONE',  ( 26.99999999999999645, 7.347880794884117764E-16, -7.368749998770962151 ) ) ;
#12116=CARTESIAN_POINT ( 'NONE',  ( 24.75598086634022010, 0.000000000000000000, 164.5679854722048958 ) ) ;
#12128=CARTESIAN_POINT ( 'NONE',  ( 37.48648511030115316, -3.604726614523235284, 166.8044593776906481 ) ) ;
#12129=CARTESIAN_POINT ( 'NONE',  ( 18.12178482187499640, 4.985214923628404904, -3.365624999385474769 ) ) ;
#12138=ORIENTED_EDGE ( 'NONE', *, *, #9024, .T. ) ;
#12141=CARTESIAN_POINT ( 'NONE',  ( 15.24356964375000167, -3.323476615752272600, -0.5531249993854806535 ) ) ;
#12144=EDGE_CURVE ( 'NONE', #972, #4178, #1954, .T. ) ;
#12145=CARTESIAN_POINT ( 'NONE',  ( 31.27239372959508756, -6.928203230275514990, 167.4139976038384532 ) ) ;
#12146=ORIENTED_EDGE ( 'NONE', *, *, #13809, .T. ) ;
#12149=CARTESIAN_POINT ( 'NONE',  ( 27.93288733171263516, 5.407089921784862696, 165.0617286715140608 ) ) ;
#12154=EDGE_CURVE ( 'NONE', #10052, #16958, #21360, .T. ) ;
#12155=CARTESIAN_POINT ( 'NONE',  ( 15.00000000000000355, 7.347880794884112834E-16, 50.26196565745150480 ) ) ;
#12157=CARTESIAN_POINT ( 'NONE',  ( 28.05502581071438328, -5.196152422706632912, 165.0604537508149008 ) ) ;
#12158=CARTESIAN_POINT ( 'NONE',  ( 24.87690945940258302, -3.604726614523240613, 165.9502056158071355 ) ) ;
#12160=( BOUNDED_CURVE ( )  B_SPLINE_CURVE ( 2, ( #31960, #6747, #35732, #9217, #17754, #15091, #20788 ),
 .UNSPECIFIED., .F., .F. ) 
 B_SPLINE_CURVE_WITH_KNOTS ( ( 3, 2, 2, 3 ),
 ( 0.9347826086956532166, 0.9420289855072474516, 0.9492753623188416867, 0.9565217391304360328 ),
 .UNSPECIFIED. ) 
 CURVE ( )  GEOMETRIC_REPRESENTATION_ITEM ( )  RATIONAL_B_SPLINE_CURVE ( ( 0.9999999999999815703, 0.8660254037844571373, 1.000000000000000000, 0.8660254037844387076, 1.000000000000000000, 0.8660254037844161701, 1.000000000000022649 ) ) 
 REPRESENTATION_ITEM ( '' )  );
#12177=CARTESIAN_POINT ( 'NONE',  ( 36.64165061258780298, 7.347880794884117764E-16, 159.9426051293869477 ) ) ;
#12185=EDGE_CURVE ( 'NONE', #6022, #28136, #10730, .T. ) ;
#12188=CARTESIAN_POINT ( 'NONE',  ( 21.00000000000000000, 6.646953231504538984, -2.615624999385474325 ) ) ;
#12193=CARTESIAN_POINT ( 'NONE',  ( 23.87821517812499650, 4.985214923628404904, -4.790624999385456384 ) ) ;
#12202=CARTESIAN_POINT ( 'NONE',  ( 24.78863278643100188, -3.464101615137757051, 162.1465503788904243 ) ) ;
#12207=CARTESIAN_POINT ( 'NONE',  ( 20.99999999999999645, 6.646953231504538984, -6.665624999385467930 ) ) ;
#12212=CARTESIAN_POINT ( 'NONE',  ( 15.00000000000000000, 0.000000000000000000, -0.8437499987709595750 ) ) ;
#12217=CARTESIAN_POINT ( 'NONE',  ( 24.35887751344623098, 0.000000000000000000, 160.0290733790243962 ) ) ;
#12228=ORIENTED_EDGE ( 'NONE', *, *, #24193, .F. ) ;
#12229=CARTESIAN_POINT ( 'NONE',  ( 15.00000000000000178, -3.464101615137757051, -8.062499999999991118 ) ) ;
#12230=CARTESIAN_POINT ( 'NONE',  ( 14.99999999999936229, 3.464101615137384904, -3.187499999999991118 ) ) ;
#12234=CARTESIAN_POINT ( 'NONE',  ( 31.14247720061542424, -7.209453229046475009, 165.9290448826076272 ) ) ;
#12239=ORIENTED_EDGE ( 'NONE', *, *, #29268, .T. ) ;
#12244=CARTESIAN_POINT ( 'NONE',  ( 26.75643035624999655, 7.049594010296217766E-16, -5.315624999385482496 ) ) ;
#12248=EDGE_CURVE ( 'NONE', #8427, #15760, #7075, .T. ) ;
#12251=CARTESIAN_POINT ( 'NONE',  ( 21.00000000000000355, 0.000000000000000000, 50.00000000000001421 ) ) ;
#12252=CARTESIAN_POINT ( 'NONE',  ( 36.81484116775207127, -3.604726614523238837, 159.1275339855211257 ) ) ;
#12258=CARTESIAN_POINT ( 'NONE',  ( 15.24356964374999990, 0.000000000000000000, -0.7031249993854904456 ) ) ;
#12262=ORIENTED_EDGE ( 'NONE', *, *, #8908, .F. ) ;
#12266=CARTESIAN_POINT ( 'NONE',  ( 20.53679726638638314, 5.749653476603932667, -8.000000000000005329 ) ) ;
#12267=CARTESIAN_POINT ( 'NONE',  ( 24.94391043663983965, 3.604726614523240613, 166.7160302899652322 ) ) ;
#12272=ADVANCED_FACE ( 'NONE', ( #34959 ), #3122, .T. ) ;
#12278=CARTESIAN_POINT ( 'NONE',  ( 30.63261610554166126, -7.209453229046475009, 160.1013058987709314 ) ) ;
#12279=CARTESIAN_POINT ( 'NONE',  ( 23.87821517812500005, -4.985214923628404016, -8.990624999385465443 ) ) ;
#12281=CARTESIAN_POINT ( 'NONE',  ( 37.36719068741531657, 7.646167579472024665E-16, 165.4409178846775603 ) ) ;
#12283=CARTESIAN_POINT ( 'NONE',  ( 37.02731477413906447, 3.464101615137759271, 164.3507666672186076 ) ) ;
#12284=DIRECTION ( 'NONE',  ( 0.000000000000000000, 0.000000000000000000, 1.000000000000000000 ) ) ;
#12287=ADVANCED_FACE ( 'NONE', ( #9004 ), #26616, .T. ) ;
#12294=CARTESIAN_POINT ( 'NONE',  ( 21.00000000000000000, 6.646953231504538984, -4.865624999385484983 ) ) ;
#12309=CARTESIAN_POINT ( 'NONE',  ( 24.71676078210377625, 0.000000000000000000, 164.1196978580636028 ) ) ;
#12322=CARTESIAN_POINT ( 'NONE',  ( 25.03052145599531997, 0.000000000000000000, 167.7059987711938902 ) ) ;
#12323=CARTESIAN_POINT ( 'NONE',  ( 23.87821517812500005, -4.985214923628404016, -2.240624999385460114 ) ) ;
#12334=CARTESIAN_POINT ( 'NONE',  ( 18.12178482187500350, -4.985214923628407568, -2.315624999385479388 ) ) ;
#12337=CARTESIAN_POINT ( 'NONE',  ( 26.99999999999999645, -3.464101615137751278, -7.856249998770961085 ) ) ;
#12343=CARTESIAN_POINT ( 'NONE',  ( 31.00030439525832193, 7.209453229046482114, 164.3040022813455039 ) ) ;
#12351=CARTESIAN_POINT ( 'NONE',  ( 34.33409119757650529, -5.407089921784855591, 166.5908959372197558 ) ) ;
#12355=VECTOR ( 'NONE', #9951, 1000.000000000000000 ) ;
#12358=AXIS2_PLACEMENT_3D ( 'NONE', #24560, #37225, #36852 ) ;
#12369=( BOUNDED_CURVE ( )  B_SPLINE_CURVE ( 3, ( #17173, #28900, #5965, #22862 ),
 .UNSPECIFIED., .F., .F. ) 
 B_SPLINE_CURVE_WITH_KNOTS ( ( 4, 4 ),
 ( 4.712388980384729642, 6.283185307179586232 ),
 .UNSPECIFIED. ) 
 CURVE ( )  GEOMETRIC_REPRESENTATION_ITEM ( )  RATIONAL_B_SPLINE_CURVE ( ( 1.000000000000000000, 0.8047378541243743744, 0.8047378541243743744, 1.000000000000000000 ) ) 
 REPRESENTATION_ITEM ( '' )  );
#12371=CARTESIAN_POINT ( 'NONE',  ( 15.59980547062007616, -2.577807756931967287, -7.999999999999994671 ) ) ;
#12373=CARTESIAN_POINT ( 'NONE',  ( 24.99999999999999289, 0.000000000000000000, 50.00000000000000000 ) ) ;
#12375=DIRECTION ( 'NONE',  ( 0.08715574274765150453, 0.000000000000000000, 0.9961946980917461003 ) ) ;
#12381=CARTESIAN_POINT ( 'NONE',  ( 26.75643035624999655, -3.323476615752267715, -4.565624999385477167 ) ) ;
#12384=ADVANCED_FACE ( 'NONE', ( #8633 ), #8819, .T. ) ;
#12387=CARTESIAN_POINT ( 'NONE',  ( 15.24356964374999990, 0.000000000000000000, -5.990624999385463667 ) ) ;
#12393=CARTESIAN_POINT ( 'NONE',  ( 30.67428744509644289, 6.928203230275506996, 160.5776114894082127 ) ) ;
#12397=CARTESIAN_POINT ( 'NONE',  ( 15.24356964374999990, 3.323476615752268604, -6.140624999385478233 ) ) ;
#12402=CARTESIAN_POINT ( 'NONE',  ( 30.85077782416043490, -6.928203230275506996, 162.5949057530440029 ) ) ;
#12406=CARTESIAN_POINT ( 'NONE',  ( 30.68654372136677821, 7.209453229046482114, 160.7177013682151596 ) ) ;
#12409=EDGE_CURVE ( 'NONE', #10799, #24633, #12369, .T. ) ;
#12421=CARTESIAN_POINT ( 'NONE',  ( 24.00000000000000000, -5.196152422706629359, -7.050000000000000711 ) ) ;
#12426=CARTESIAN_POINT ( 'NONE',  ( 34.26872439051576436, 5.407089921784857367, 165.8437499136509814 ) ) ;
#12427=DIRECTION ( 'NONE',  ( -0.9810603962227041341, -0.1736474146266793750, 0.08583166290373737961 ) ) ;
#12430=ORIENTED_EDGE ( 'NONE', *, *, #20852, .F. ) ;
#12436=CARTESIAN_POINT ( 'NONE',  ( 23.87821517812499650, 4.985214923628404904, -7.490624999385464555 ) ) ;
#12445=CARTESIAN_POINT ( 'NONE',  ( 24.35560917309319251, 3.604726614523240613, 159.9917160778459220 ) ) ;
#12458=CARTESIAN_POINT ( 'NONE',  ( 31.23562490067698150, 7.209453229046482114, 166.9937279661931768 ) ) ;
#12466=CARTESIAN_POINT ( 'NONE',  ( 24.69385091608528526, 3.464101615137450185, 161.0631886434913440 ) ) ;
#12469=CARTESIAN_POINT ( 'NONE',  ( 24.36704836432882004, -3.604726614523240613, 160.1224666319704681 ) ) ;
#12471=CARTESIAN_POINT ( 'NONE',  ( 15.24356964374999990, 3.323476615752268604, -9.178124999385456562 ) ) ;
#12473=CARTESIAN_POINT ( 'NONE',  ( 34.26382187998621731, 5.407089921784862696, 165.7877139618832985 ) ) ;
#12474=CARTESIAN_POINT ( 'NONE',  ( 25.08605175845023894, 3.464101615137757051, 165.5460647849041607 ) ) ;
#12481=ORIENTED_EDGE ( 'NONE', *, *, #26262, .T. ) ;
#12486=CARTESIAN_POINT ( 'NONE',  ( 23.87821517812500005, -4.985214923628404016, -7.753124999385491378 ) ) ;
#12489=AXIS2_PLACEMENT_3D ( 'NONE', #13296, #1728, #15962 ) ;
#12503=CARTESIAN_POINT ( 'NONE',  ( 15.00000000000000000, 0.000000000000000000, -1.743749998770943721 ) ) ;
#12504=CARTESIAN_POINT ( 'NONE',  ( 27.95086320365434318, -5.407089921784859143, 165.2671938279954702 ) ) ;
#12507=FACE_OUTER_BOUND ( 'NONE', #13544, .T. ) ;
#12516=CARTESIAN_POINT ( 'NONE',  ( 28.09467017918796472, 5.407089921784856479, 166.9109150798468306 ) ) ;
#12517=CARTESIAN_POINT ( 'NONE',  ( 23.87821517812499650, 4.985214923628404904, -2.090624999385476634 ) ) ;
#12518=AXIS2_PLACEMENT_3D ( 'NONE', #12251, #29874, #23821 ) ;
#12526=ORIENTED_EDGE ( 'NONE', *, *, #26608, .T. ) ;
#12527=ORIENTED_EDGE ( 'NONE', *, *, #20519, .T. ) ;
#12530=CARTESIAN_POINT ( 'NONE',  ( 23.87821517812499650, 4.985214923628404904, -2.540624999385482141 ) ) ;
#12532=CARTESIAN_POINT ( 'NONE',  ( 26.99999999999999645, 3.464101615137755275, -8.231249998770962861 ) ) ;
#12540=CARTESIAN_POINT ( 'NONE',  ( 37.12860184164360788, -3.604726614523238837, 162.7138348986514131 ) ) ;
#12547=CARTESIAN_POINT ( 'NONE',  ( 24.90959286293295349, 3.604726614523236616, 166.3237786275915937 ) ) ;
#12562=FACE_OUTER_BOUND ( 'NONE', #7893, .T. ) ;
#12566=DIRECTION ( 'NONE',  ( 1.000000000000000000, 0.000000000000000000, 0.000000000000000000 ) ) ;
#12568=CARTESIAN_POINT ( 'NONE',  ( 28.04195244930222586, 5.196152422706630247, 164.9110245461011743 ) ) ;
#12574=CARTESIAN_POINT ( 'NONE',  ( 23.87821517812499650, 4.985214923628404904, -4.903124999385472194 ) ) ;
#12577=CARTESIAN_POINT ( 'NONE',  ( 20.99999999999999645, 6.646953231504538984, -7.903124999385464200 ) ) ;
#12583=CARTESIAN_POINT ( 'NONE',  ( 36.60569886870439404, 3.464101615137755275, 159.5316748164241574 ) ) ;
#12587=CARTESIAN_POINT ( 'NONE',  ( 18.12178482187499640, 4.985214923628404904, -7.528124999385488181 ) ) ;
#12596=CARTESIAN_POINT ( 'NONE',  ( 27.51453976652391376, -5.407089921784865361, 160.2799941206736776 ) ) ;
#12597=ORIENTED_EDGE ( 'NONE', *, *, #36966, .T. ) ;
#12608=VERTEX_POINT ( 'NONE', #21141 ) ;
#12609=CARTESIAN_POINT ( 'NONE',  ( 26.99999999999999645, -3.464101615137751278, -7.462500000000007461 ) ) ;
#12610=CARTESIAN_POINT ( 'NONE',  ( 24.00000000000000000, -5.196152422706629359, -4.349999999999992539 ) ) ;
#12613=CARTESIAN_POINT ( 'NONE',  ( 37.14004103287923186, 3.604726614523238837, 162.8445854527759309 ) ) ;
#12619=VECTOR ( 'NONE', #16804, 1000.000000000000000 ) ;
#12623=CARTESIAN_POINT ( 'NONE',  ( 37.22995187613445012, 7.347880794884117764E-16, 166.6669193415062580 ) ) ;
#12625=CARTESIAN_POINT ( 'NONE',  ( 26.75643035624999655, -3.323476615752267715, -9.403124999385470417 ) ) ;
#12632=CARTESIAN_POINT ( 'NONE',  ( 31.16453849805197862, -6.928203230275506996, 166.1812066661742904 ) ) ;
#12641=EDGE_CURVE ( 'NONE', #26027, #15426, #16012, .T. ) ;
#12642=EDGE_LOOP ( 'NONE', ( #17704, #14999, #30614, #8493 ) ) ;
#12646=CARTESIAN_POINT ( 'NONE',  ( 37.44563085588819717, 7.646167579472024665E-16, 166.3374931129601464 ) ) ;
#12655=CARTESIAN_POINT ( 'NONE',  ( 15.00000000000000000, 0.000000000000000000, -4.500000000000003553 ) ) ;
#12658=ORIENTED_EDGE ( 'NONE', *, *, #14057, .F. ) ;
#12660=CARTESIAN_POINT ( 'NONE',  ( 15.24356964374999990, 0.000000000000000000, -9.590624999385454430 ) ) ;
#12661=CARTESIAN_POINT ( 'NONE',  ( 37.01094158893428698, -3.604726614523238837, 161.3689720562275909 ) ) ;
#12662=CARTESIAN_POINT ( 'NONE',  ( 37.02077809343298753, -3.464101615137755275, 164.2760520648617160 ) ) ;
#12669=B_SPLINE_CURVE_WITH_KNOTS ( 'NONE', 3,
 ( #5244, #12701, #36889, #16639, #32977, #30847, #25154, #30141, #13604, #15553, #9858, #15741, #31035, #19676, #2399, #7914, #2211, #31215, #16451, #13793, #22321, #1133, #25340, #22509, #5057, #8102 ),
 .UNSPECIFIED., .F., .F.,
 ( 4, 2, 2, 2, 2, 2, 2, 2, 2, 2, 2, 2, 4 ),
 ( 0.000000000000000000, 0.001454664733950383586, 0.002181997100925580149, 0.002909329467900777580, 0.004363994201851170707, 0.005091326568826366403, 0.005818658935801563833, 0.006545991302776761264, 0.007273323669751959562, 0.008727988403702353556, 0.01018265313765274842, 0.01090998550462794758, 0.01163731787160314328 ),
 .UNSPECIFIED. ) ;
#12673=CARTESIAN_POINT ( 'NONE',  ( 26.75643035624999655, 7.049594010296217766E-16, -6.328124999385481786 ) ) ;
#12682=CARTESIAN_POINT ( 'NONE',  ( 15.00000000000000355, 7.347880794884112834E-16, -8.000000000000000000 ) ) ;
#12686=CARTESIAN_POINT ( 'NONE',  ( 27.87242303518145548, -5.407089921784859143, 164.3706185997128841 ) ) ;
#12688=CARTESIAN_POINT ( 'NONE',  ( 24.69711925643884598, 0.000000000000000000, 161.1005459446697614 ) ) ;
#12691=DIRECTION ( 'NONE',  ( 0.9961946980917462113, 0.000000000000000000, -0.08715574274765118534 ) ) ;
#12696=EDGE_LOOP ( 'NONE', ( #64, #26312, #16210, #12096 ) ) ;
#12697=CARTESIAN_POINT ( 'NONE',  ( 25.03378979634835488, -3.604726614523240613, 167.7433560723723076 ) ) ;
#12698=CARTESIAN_POINT ( 'NONE',  ( 21.00000000000000000, -6.646953231504538984, -3.178124999385461003 ) ) ;
#12699=DIRECTION ( 'NONE',  ( 1.000000000000000000, 0.000000000000000000, 0.000000000000000000 ) ) ;
#12701=CARTESIAN_POINT ( 'NONE',  ( 20.48038928096284650, -5.986770049455423681, -7.999999999999998224 ) ) ;
#12703=CARTESIAN_POINT ( 'NONE',  ( 37.11229162342512211, 7.347880794884117764E-16, 165.3220564990824073 ) ) ;
#12708=VERTEX_POINT ( 'NONE', #18108 ) ;
#12713=CARTESIAN_POINT ( 'NONE',  ( 26.75643035624999655, 7.049594010296217766E-16, -1.265624999385456251 ) ) ;
#12716=CARTESIAN_POINT ( 'NONE',  ( 18.00000000000000355, -5.196152422706632912, -9.768749998770948295 ) ) ;
#12724=CARTESIAN_POINT ( 'NONE',  ( 37.20704201011650269, -3.604726614523238837, 163.6104101269339424 ) ) ;
#12726=( BOUNDED_CURVE ( )  B_SPLINE_CURVE ( 2, ( #2343, #31160, #11060, #27935, #37200, #16757, #10497 ),
 .UNSPECIFIED., .F., .F. ) 
 B_SPLINE_CURVE_WITH_KNOTS ( ( 3, 2, 2, 3 ),
 ( 0.1739130434782606149, 0.1811594202898547112, 0.1884057971014488075, 0.1956521739130429038 ),
 .UNSPECIFIED. ) 
 CURVE ( )  GEOMETRIC_REPRESENTATION_ITEM ( )  RATIONAL_B_SPLINE_CURVE ( ( 1.000000000000004663, 0.8660254037844340447, 1.000000000000000000, 0.8660254037844387076, 1.000000000000000000, 0.8660254037844494768, 0.9999999999999892308 ) ) 
 REPRESENTATION_ITEM ( '' )  );
#12730=LINE ( 'NONE', #24482, #7330 ) ;
#12733=CARTESIAN_POINT ( 'NONE',  ( 34.37331128181295270, -5.407089921784855591, 167.0391835513610488 ) ) ;
#12749=CARTESIAN_POINT ( 'NONE',  ( 18.00000000000000000, 5.196152422706630247, -1.425000000000009592 ) ) ;
#12751=CYLINDRICAL_SURFACE ( 'NONE', #19872, 6.000000000000001776 ) ;
#12753=CARTESIAN_POINT ( 'NONE',  ( 27.83604700695378398, 5.196152422706636465, 162.5575145706350781 ) ) ;
#12755=VERTEX_POINT ( 'NONE', #21145 ) ;
#12760=CARTESIAN_POINT ( 'NONE',  ( 21.00000000000000000, -6.646953231504538984, -4.190624999385508254 ) ) ;
#12763=EDGE_LOOP ( 'NONE', ( #518, #35136, #5399, #17789 ) ) ;
#12773=CARTESIAN_POINT ( 'NONE',  ( 20.99999999999999645, 6.646953231504538984, -7.115624999385463667 ) ) ;
#12774=FACE_OUTER_BOUND ( 'NONE', #21343, .T. ) ;
#12777=DIRECTION ( 'NONE',  ( 0.08715574274765150453, 0.000000000000000000, 0.9961946980917461003 ) ) ;
#12788=DIRECTION ( 'NONE',  ( 0.08715574274765150453, 0.000000000000000000, 0.9961946980917461003 ) ) ;
#12794=ORIENTED_EDGE ( 'NONE', *, *, #20123, .T. ) ;
#12798=CARTESIAN_POINT ( 'NONE',  ( 34.15106413780644345, 5.407089921784857367, 164.4988870712271023 ) ) ;
#12804=CARTESIAN_POINT ( 'NONE',  ( 27.57131143846490673, 5.196152422706630247, 159.5315731764057716 ) ) ;
#12805=CARTESIAN_POINT ( 'NONE',  ( 15.24356964374999990, 3.323476615752268604, -1.078124999385470462 ) ) ;
#12807=CARTESIAN_POINT ( 'NONE',  ( 24.77555942491173369, 0.000000000000000000, 161.9971211729523475 ) ) ;
#12808=CARTESIAN_POINT ( 'NONE',  ( 26.75643035624999655, 3.323476615752271712, -9.778124999385472194 ) ) ;
#12816=CARTESIAN_POINT ( 'NONE',  ( 37.27244030072392889, 3.464101615137755275, 167.1525642568259968 ) ) ;
#12829=CARTESIAN_POINT ( 'NONE',  ( 37.41624727615045742, 7.347880794884125653E-16, 168.7962855074530069 ) ) ;
#12830=CARTESIAN_POINT ( 'NONE',  ( 31.33367511126808935, -7.209453229046482114, 168.1144470015464378 ) ) ;
#12832=AXIS2_PLACEMENT_3D ( 'NONE', #22915, #17038, #20256 ) ;
#12836=DIRECTION ( 'NONE',  ( 0.000000000000000000, 0.000000000000000000, 1.000000000000000000 ) ) ;
#12844=DIRECTION ( 'NONE',  ( 0.08715574274765150453, 0.000000000000000000, 0.9961946980917461003 ) ) ;
#12846=CARTESIAN_POINT ( 'NONE',  ( 15.24356964374999990, 0.000000000000000000, -9.140624999385476457 ) ) ;
#12848=CARTESIAN_POINT ( 'NONE',  ( 33.93698784468253393, -5.407089921784861808, 162.0519838440392562 ) ) ;
#12849=CARTESIAN_POINT ( 'NONE',  ( 33.80667851479820030, 5.196152422706637353, 161.9598655117922874 ) ) ;
#12861=CARTESIAN_POINT ( 'NONE',  ( 26.75643035624999655, 3.323476615752271712, -5.840624999385470417 ) ) ;
#12874=CARTESIAN_POINT ( 'NONE',  ( 27.79398286670857132, -5.407089921784859143, 163.4740433714303265 ) ) ;
#12879=CARTESIAN_POINT ( 'NONE',  ( 31.35083389806797527, -6.928203230275514990, 168.3105728321210393 ) ) ;
#12887=CARTESIAN_POINT ( 'NONE',  ( 37.48975345065418452, 7.646167579472015790E-16, 166.8418166788690655 ) ) ;
#12888=CARTESIAN_POINT ( 'NONE',  ( 15.24356964375000167, -3.323476615752272600, -3.703124999385450700 ) ) ;
#12892=CARTESIAN_POINT ( 'NONE',  ( 28.39820154767614468, -5.196152422706638241, 168.9829703733268218 ) ) ;
#12893=CARTESIAN_POINT ( 'NONE',  ( 25.13834520420595098, 0.000000000000000000, 166.1437816049835874 ) ) ;
#12899=B_SPLINE_CURVE_WITH_KNOTS ( 'NONE', 3,
 ( #10792, #25004, #7582, #18454, #19159, #7770, #16303, #30708, #6688, #29996, #35674, #3836, #1178, #29802, #15599, #21108, #27155, #32834, #4727, #22365, #25198, #27850, #12371, #15414, #18073, #13645 ),
 .UNSPECIFIED., .F., .F.,
 ( 4, 2, 2, 2, 2, 2, 2, 2, 2, 2, 2, 2, 4 ),
 ( 0.000000000000000000, 0.001456441005936622663, 0.002184661508904929550, 0.002912882011873236653, 0.004369323017809840018, 0.005097543520778138014, 0.005825764023746436877, 0.007282205029683033737, 0.008010425532651330865, 0.008738646035619629729, 0.01019508704155622919, 0.01092330754452452632, 0.01165152804749282692 ),
 .UNSPECIFIED. ) ;
#12905=CARTESIAN_POINT ( 'NONE',  ( 18.12178482187500350, -4.985214923628407568, -1.865624999385473437 ) ) ;
#12907=CARTESIAN_POINT ( 'NONE',  ( 26.75643035624999655, -3.323476615752267715, -0.5156249993854836733 ) ) ;
#12908=VERTEX_POINT ( 'NONE', #24165 ) ;
#12915=CARTESIAN_POINT ( 'NONE',  ( 24.75107835581066240, 0.000000000000000000, 164.5119495204372413 ) ) ;
#12922=CARTESIAN_POINT ( 'NONE',  ( 24.99130137175887612, 0.000000000000000000, 167.2577111570525972 ) ) ;
#12939=DIRECTION ( 'NONE',  ( 0.000000000000000000, 0.000000000000000000, 1.000000000000000000 ) ) ;
#12941=DIRECTION ( 'NONE',  ( 0.08715574274765150453, 0.000000000000000000, 0.9961946980917461003 ) ) ;
#12950=CARTESIAN_POINT ( 'NONE',  ( 26.75643035624999655, -3.323476615752267715, -4.115624999385481431 ) ) ;
#12954=CARTESIAN_POINT ( 'NONE',  ( 18.12178482187499640, 4.985214923628404904, -7.865624999385478766 ) ) ;
#12961=CARTESIAN_POINT ( 'NONE',  ( 36.60243052835136268, 7.347880794884117764E-16, 159.4943175152456831 ) ) ;
#12967=CARTESIAN_POINT ( 'NONE',  ( 20.99999999999999645, 0.000000000000000000, -8.000000000000000000 ) ) ;
#12969=EDGE_CURVE ( 'NONE', #33229, #37335, #13608, .T. ) ;
#12971=CARTESIAN_POINT ( 'NONE',  ( 26.99999999999999645, 7.347880794884117764E-16, -3.768749998770942966 ) ) ;
#12975=CARTESIAN_POINT ( 'NONE',  ( 15.02283181144952628, 7.347880794884122694E-16, 50.52293445648592751 ) ) ;
#12977=ORIENTED_EDGE ( 'NONE', *, *, #10396, .T. ) ;
#12981=CARTESIAN_POINT ( 'NONE',  ( 25.13180852339300486, -3.464101615137899159, 166.0690670014023738 ) ) ;
#12991=LINE ( 'NONE', #1223, #12355 ) ;
#12994=CARTESIAN_POINT ( 'NONE',  ( 37.25443294523552851, 7.646167579472015790E-16, 164.1520909940213642 ) ) ;
#12995=CARTESIAN_POINT ( 'NONE',  ( 37.38029553226678559, 3.464101615137904933, 168.3853551944901596 ) ) ;
#13002=CARTESIAN_POINT ( 'NONE',  ( 23.87821517812499650, 4.985214923628404904, -0.2906249993854803648 ) ) ;
#13004=CARTESIAN_POINT ( 'NONE',  ( 30.79194769780577445, 6.928203230275506996, 161.9224743318320634 ) ) ;
#13005=CARTESIAN_POINT ( 'NONE',  ( 21.00000000000000000, -6.646953231504538984, -9.928124999385461891 ) ) ;
#13008=DIRECTION ( 'NONE',  ( 0.000000000000000000, 0.000000000000000000, 1.000000000000000000 ) ) ;
#13011=CARTESIAN_POINT ( 'NONE',  ( 25.41615413421412129, -3.464101615137772594, 169.3191522051510276 ) ) ;
#13012=CARTESIAN_POINT ( 'NONE',  ( 25.33117728503513177, 3.464101615137752166, 168.3478623745115499 ) ) ;
#13021=ORIENTED_EDGE ( 'NONE', *, *, #11477, .F. ) ;
#13024=LINE ( 'NONE', #32916, #7194 ) ;
#13025=CARTESIAN_POINT ( 'NONE',  ( 27.81522707900330715, 5.407089921784862696, 163.7168658290902101 ) ) ;
#13030=CARTESIAN_POINT ( 'NONE',  ( 24.00000000000000000, -5.196152422706629359, -3.450000000000008615 ) ) ;
#13039=CARTESIAN_POINT ( 'NONE',  ( 20.99999999999999645, 0.000000000000000000, -8.000000000000000000 ) ) ;
#13041=CARTESIAN_POINT ( 'NONE',  ( 21.00000000000000000, -6.928203230275506996, -2.587499999999983480 ) ) ;
#13043=CARTESIAN_POINT ( 'NONE',  ( 37.08938175740716758, -3.604726614523238837, 162.2655472845101201 ) ) ;
#13044=CARTESIAN_POINT ( 'NONE',  ( 36.82467767225077182, -3.464101615137755275, 162.0346139941553076 ) ) ;
#13049=ORIENTED_EDGE ( 'NONE', *, *, #27983, .T. ) ;
#13050=VERTEX_POINT ( 'NONE', #6264 ) ;
#13055=CARTESIAN_POINT ( 'NONE',  ( 26.75643035624999655, -3.323476615752267715, -6.365624999385492089 ) ) ;
#13068=CARTESIAN_POINT ( 'NONE',  ( 30.86793661096031727, -7.209453229046475009, 162.7910315836186328 ) ) ;
#13075=ADVANCED_FACE ( 'NONE', ( #34690 ), #8920, .T. ) ;
#13077=CARTESIAN_POINT ( 'NONE',  ( 15.00000000000000000, 0.000000000000000000, 0.000000000000000000 ) ) ;
#13080=CARTESIAN_POINT ( 'NONE',  ( 34.03340388509710834, 5.407089921784857367, 163.1540242288032232 ) ) ;
#13081=CARTESIAN_POINT ( 'NONE',  ( 26.75643035624999655, 3.323476615752271712, -4.828124999385488003 ) ) ;
#13092=CARTESIAN_POINT ( 'NONE',  ( 15.24356964375000167, -3.323476615752272600, -3.703124999385450700 ) ) ;
#13094=CARTESIAN_POINT ( 'NONE',  ( 15.00000000000000178, -3.464101615137757051, -9.356249998770968190 ) ) ;
#13101=CARTESIAN_POINT ( 'NONE',  ( 27.57990657358465114, 5.407089921784862696, 161.0271401442424803 ) ) ;
#13109=ORIENTED_EDGE ( 'NONE', *, *, #17603, .T. ) ;
#13110=CARTESIAN_POINT ( 'NONE',  ( 26.99999999999999645, 7.347880794884117764E-16, -5.175000000000013145 ) ) ;
#13116=CARTESIAN_POINT ( 'NONE',  ( 20.99999999999999645, -6.928203230275506996, -2.531249998770942256 ) ) ;
#13135=CARTESIAN_POINT ( 'NONE',  ( 26.75643035624999655, -3.323476615752267715, -5.465624999385500615 ) ) ;
#13137=ORIENTED_EDGE ( 'NONE', *, *, #4364, .F. ) ;
#13138=CARTESIAN_POINT ( 'NONE',  ( 26.75643035624999655, 3.323476615752271268, -6.628124999385470062 ) ) ;
#13143=CARTESIAN_POINT ( 'NONE',  ( 37.52080268400803931, -3.604726614523238837, 167.1967110400642866 ) ) ;
#13146=CARTESIAN_POINT ( 'NONE',  ( 26.99999999999999645, 7.347880794884117764E-16, -7.424999999999987388 ) ) ;
#13149=( BOUNDED_CURVE ( )  B_SPLINE_CURVE ( 2, ( #5496, #17079, #28618, #12879, #32967, #9664, #32780 ),
 .UNSPECIFIED., .F., .F. ) 
 B_SPLINE_CURVE_WITH_KNOTS ( ( 3, 2, 2, 3 ),
 ( 0.1086956521739124576, 0.1159420289855068037, 0.1231884057971011498, 0.1304347826086954820 ),
 .UNSPECIFIED. ) 
 CURVE ( )  GEOMETRIC_REPRESENTATION_ITEM ( )  RATIONAL_B_SPLINE_CURVE ( ( 1.000000000000010658, 0.8660254037844279384, 1.000000000000000000, 0.8660254037844387076, 1.000000000000000000, 0.8660254037844418162, 0.9999999999999968914 ) ) 
 REPRESENTATION_ITEM ( '' )  );
#13151=CARTESIAN_POINT ( 'NONE',  ( 24.00000000000000000, -5.196152422706629359, -2.943749998770950338 ) ) ;
#13159=ORIENTED_EDGE ( 'NONE', *, *, #19130, .F. ) ;
#13163=CARTESIAN_POINT ( 'NONE',  ( 20.99999999999999645, 0.000000000000000000, -8.000000000000000000 ) ) ;
#13165=CARTESIAN_POINT ( 'NONE',  ( 34.07795076420737246, -5.196152422706629359, 165.0605215108271864 ) ) ;
#13166=( BOUNDED_CURVE ( )  B_SPLINE_CURVE ( 2, ( #30498, #36726, #2415, #1673, #7741, #4519, #19134 ),
 .UNSPECIFIED., .F., .F. ) 
 B_SPLINE_CURVE_WITH_KNOTS ( ( 3, 2, 2, 3 ),
 ( 0.000000000000000000, 0.007246376811594042525, 0.01449275362318808505, 0.02173913043478212584 ),
 .UNSPECIFIED. ) 
 CURVE ( )  GEOMETRIC_REPRESENTATION_ITEM ( )  RATIONAL_B_SPLINE_CURVE ( ( 1.000000000000000000, 0.8660254037844387076, 1.000000000000000000, 0.8660254037844387076, 1.000000000000000000, 0.8660254037844475894, 0.9999999999999911182 ) ) 
 REPRESENTATION_ITEM ( '' )  );
#13171=CARTESIAN_POINT ( 'NONE',  ( 21.00000000000000355, 0.000000000000000000, 50.00000000000001421 ) ) ;
#13174=ADVANCED_FACE ( 'NONE', ( #37162 ), #15552, .T. ) ;
#13176=CARTESIAN_POINT ( 'NONE',  ( 24.87690945940258302, -3.604726614523240613, 165.9502056158071355 ) ) ;
#13183=ORIENTED_EDGE ( 'NONE', *, *, #15057, .T. ) ;
#13184=CARTESIAN_POINT ( 'NONE',  ( 21.00000000000000000, 6.928203230275506996, -5.456249998770962506 ) ) ;
#13185=CARTESIAN_POINT ( 'NONE',  ( 18.12178482187499640, 4.985214923628404904, -1.115624999385472771 ) ) ;
#13188=CARTESIAN_POINT ( 'NONE',  ( 21.00000000000000000, 6.646953231504538984, -9.703124999385480010 ) ) ;
#13198=CARTESIAN_POINT ( 'NONE',  ( 37.22668353578141875, -3.464101615137751278, 166.6295620403278406 ) ) ;
#13204=CARTESIAN_POINT ( 'NONE',  ( 26.75643035624999655, -3.323476615752267271, -2.765624999385494664 ) ) ;
#13208=VERTEX_POINT ( 'NONE', #36004 ) ;
#13209=CARTESIAN_POINT ( 'NONE',  ( 37.22995187613445012, 7.347880794884117764E-16, 166.6669193415062580 ) ) ;
#13213=CARTESIAN_POINT ( 'NONE',  ( 27.93288733171263516, 5.407089921784862696, 165.0617286715140608 ) ) ;
#13215=( BOUNDED_CURVE ( )  B_SPLINE_CURVE ( 2, ( #33306, #36697, #30470, #10367, #19297, #30836, #36508 ),
 .UNSPECIFIED., .F., .F. ) 
 B_SPLINE_CURVE_WITH_KNOTS ( ( 3, 2, 2, 3 ),
 ( 0.2173913043478263030, 0.2246376811594205936, 0.2318840579710149119, 0.2391304347826092025 ),
 .UNSPECIFIED. ) 
 CURVE ( )  GEOMETRIC_REPRESENTATION_ITEM ( )  RATIONAL_B_SPLINE_CURVE ( ( 0.9999999999999958922, 0.8660254037844428154, 1.000000000000000000, 0.8660254037844387076, 1.000000000000000000, 0.8660254037844294928, 1.000000000000009326 ) ) 
 REPRESENTATION_ITEM ( '' )  );
#13225=AXIS2_PLACEMENT_3D ( 'NONE', #3416, #18787, #12699 ) ;
#13231=CARTESIAN_POINT ( 'NONE',  ( 23.99999999999999645, 5.196152422706631135, -3.299999999999997158 ) ) ;
#13232=CARTESIAN_POINT ( 'NONE',  ( 34.02850137456756130, 5.407089921784862696, 163.0979882770355971 ) ) ;
#13233=CARTESIAN_POINT ( 'NONE',  ( 36.83121435295684165, 3.464101615137759271, 162.1093285965121709 ) ) ;
#13235=DIRECTION ( 'NONE',  ( 0.9961946980917462113, 0.000000000000000000, -0.08715574274765118534 ) ) ;
#13244=CARTESIAN_POINT ( 'NONE',  ( 23.87821517812499650, 4.985214923628404904, -7.603124999385480365 ) ) ;
#13252=CARTESIAN_POINT ( 'NONE',  ( 24.97165984609394940, 0.000000000000000000, 164.2385592436587558 ) ) ;
#13256=LINE ( 'NONE', #9843, #29820 ) ;
#13257=CARTESIAN_POINT ( 'NONE',  ( 27.67632261399923976, -5.407089921784859143, 162.1291805290064474 ) ) ;
#13266=CARTESIAN_POINT ( 'NONE',  ( 27.89856975800574546, 5.407089921784856479, 164.6694770091404223 ) ) ;
#13267=CARTESIAN_POINT ( 'NONE',  ( 15.24356964374999990, 3.323476615752268604, -5.128124999385462957 ) ) ;
#13274=VERTEX_POINT ( 'NONE', #26721 ) ;
#13278=CARTESIAN_POINT ( 'NONE',  ( 18.12178482187499640, 4.985214923628404904, -4.265624999385458693 ) ) ;
#13281=CARTESIAN_POINT ( 'NONE',  ( 15.00000000000000000, 3.464101615137752166, -8.531249998770938703 ) ) ;
#13283=ORIENTED_EDGE ( 'NONE', *, *, #12010, .T. ) ;
#13287=CARTESIAN_POINT ( 'NONE',  ( 36.93576976081443775, 7.646167579472024665E-16, 160.5097541291234506 ) ) ;
#13290=SHAPE_REPRESENTATION_RELATIONSHIP ( 'NONE' , 'NONE' ,  #29986, #10611 ) ;
#13296=CARTESIAN_POINT ( 'NONE',  ( 21.00000000000000355, 0.000000000000000000, 50.00000000000001421 ) ) ;
#13304=DIRECTION ( 'NONE',  ( 0.08715574274765150453, 0.000000000000000000, 0.9961946980917461003 ) ) ;
#13310=CARTESIAN_POINT ( 'NONE',  ( 18.00000000000000355, -5.196152422706632912, -1.668749998770951981 ) ) ;
#13314=CARTESIAN_POINT ( 'NONE',  ( 21.00000000000000000, 6.928203230275506996, -9.562499999999998224 ) ) ;
#13315=ORIENTED_EDGE ( 'NONE', *, *, #12010, .F. ) ;
#13320=CARTESIAN_POINT ( 'NONE',  ( 23.87821517812499650, 4.985214923628404904, -7.603124999385480365 ) ) ;
#13323=CARTESIAN_POINT ( 'NONE',  ( 23.87821517812500005, -4.985214923628404016, -6.740624999385463667 ) ) ;
#13327=AXIS2_PLACEMENT_3D ( 'NONE', #28258, #25414, #27703 ) ;
#13334=CARTESIAN_POINT ( 'NONE',  ( 20.99999999999999645, 0.000000000000000000, -8.000000000000000000 ) ) ;
#13335=CARTESIAN_POINT ( 'NONE',  ( 14.99999999999960387, -3.464101615137527457, -3.056249998770969256 ) ) ;
#13343=CARTESIAN_POINT ( 'NONE',  ( 26.97716818855048260, 0.000000000000000000, 49.47706554351410801 ) ) ;
#13349=CARTESIAN_POINT ( 'NONE',  ( 34.10736582727759725, -5.196152422706635576, 165.3967372202087915 ) ) ;
#13361=CARTESIAN_POINT ( 'NONE',  ( 24.71349244175073778, 3.604726614523236616, 164.0823405568851570 ) ) ;
#13367=ORIENTED_EDGE ( 'NONE', *, *, #31820, .F. ) ;
#13368=CARTESIAN_POINT ( 'NONE',  ( 23.99999999999999645, 5.196152422706631135, -3.693749998770950782 ) ) ;
#13369=CARTESIAN_POINT ( 'NONE',  ( 15.24356964374999990, 3.323476615752268604, -0.1781249993854788494 ) ) ;
#13371=CARTESIAN_POINT ( 'NONE',  ( 18.00000000000000000, 5.196152422706630247, -5.925000000000013145 ) ) ;
#13372=CARTESIAN_POINT ( 'NONE',  ( 15.24356964375000167, -3.323476615752272600, -7.753124999385476279 ) ) ;
#13375=( BOUNDED_CURVE ( )  B_SPLINE_CURVE ( 3, ( #323, #6204, #35192, #14928 ),
 .UNSPECIFIED., .F., .F. ) 
 B_SPLINE_CURVE_WITH_KNOTS ( ( 4, 4 ),
 ( 1.570796326794937858, 3.141592653589793116 ),
 .UNSPECIFIED. ) 
 CURVE ( )  GEOMETRIC_REPRESENTATION_ITEM ( )  RATIONAL_B_SPLINE_CURVE ( ( 1.000000000000000000, 0.8047378541243747074, 0.8047378541243747074, 1.000000000000000000 ) ) 
 REPRESENTATION_ITEM ( '' )  );
#13380=CARTESIAN_POINT ( 'NONE',  ( 31.12531841381553477, -6.928203230275506996, 165.7329190520329973 ) ) ;
#13384=VECTOR ( 'NONE', #486, 1000.000000000000000 ) ;
#13385=CARTESIAN_POINT ( 'NONE',  ( 15.24356964375000167, -3.323476615752272600, -1.565624999385463179 ) ) ;
#13389=ORIENTED_EDGE ( 'NONE', *, *, #30081, .F. ) ;
#13390=CARTESIAN_POINT ( 'NONE',  ( 25.28542051998549667, 0.000000000000000000, 167.8248601567890432 ) ) ;
#13393=CARTESIAN_POINT ( 'NONE',  ( 37.07307153918868181, 7.347880794884117764E-16, 164.8737688849411143 ) ) ;
#13395=CARTESIAN_POINT ( 'NONE',  ( 37.32797060317886917, 7.646167579472024665E-16, 164.9926302705362957 ) ) ;
#13403=CARTESIAN_POINT ( 'NONE',  ( 24.73960768102886121, -3.464101615138067469, 161.5861908599895003 ) ) ;
#13405=CARTESIAN_POINT ( 'NONE',  ( 26.99999999999999289, 0.000000000000000000, -8.000000000000000000 ) ) ;
#13412=CARTESIAN_POINT ( 'NONE',  ( 24.00000000000000000, -5.196152422706629359, -1.650000000000012568 ) ) ;
#13413=CARTESIAN_POINT ( 'NONE',  ( 34.01542801315541453, -5.407089921784861808, 162.9485590723218422 ) ) ;
#13414=CARTESIAN_POINT ( 'NONE',  ( 27.87526709119022783, 5.196152422706636465, 163.0058021847763712 ) ) ;
#13420=EDGE_LOOP ( 'NONE', ( #5611, #9108, #9613, #31690 ) ) ;
#13422=CARTESIAN_POINT ( 'NONE',  ( 25.24946877610227958, -3.464101615137868073, 167.4139298438261676 ) ) ;
#13424=CARTESIAN_POINT ( 'NONE',  ( 21.00000000000000000, -6.646953231504538984, -9.590624999385488181 ) ) ;
#13433=( BOUNDED_CURVE ( )  B_SPLINE_CURVE ( 2, ( #3730, #9798, #21189, #9615, #21376, #15492, #18155 ),
 .UNSPECIFIED., .F., .F. ) 
 B_SPLINE_CURVE_WITH_KNOTS ( ( 3, 2, 2, 3 ),
 ( 0.7391304347826078702, 0.7463768115942021053, 0.7536231884057964514, 0.7608695652173906865 ),
 .UNSPECIFIED. ) 
 CURVE ( )  GEOMETRIC_REPRESENTATION_ITEM ( )  RATIONAL_B_SPLINE_CURVE ( ( 1.000000000000014433, 0.8660254037844243857, 1.000000000000000000, 0.8660254037844387076, 1.000000000000000000, 0.8660254037844510311, 0.9999999999999876765 ) ) 
 REPRESENTATION_ITEM ( '' )  );
#13437=CARTESIAN_POINT ( 'NONE',  ( 37.02731477413858130, 3.464101615138035051, 164.3507666672186929 ) ) ;
#13438=CARTESIAN_POINT ( 'NONE',  ( 27.63710252976279591, -5.407089921784859143, 161.6808929148651828 ) ) ;
#13439=CARTESIAN_POINT ( 'NONE',  ( 26.99999999999999645, 3.464101615137755275, -1.031249998770967347 ) ) ;
#13443=LINE ( 'NONE', #33717, #3014 ) ;
#13451=CARTESIAN_POINT ( 'NONE',  ( 24.79193261022362549, 3.604726614523236616, 164.9789157851677146 ) ) ;
#13452=CARTESIAN_POINT ( 'NONE',  ( 26.75643035624999655, 7.049594010296217766E-16, -5.315624999385482496 ) ) ;
#13455=CARTESIAN_POINT ( 'NONE',  ( 31.31161381383153497, -6.928203230275514990, 167.8622852179797462 ) ) ;
#13458=CARTESIAN_POINT ( 'NONE',  ( 29.49486714975617474, 6.148716665048037378, 159.5363409456820136 ) ) ;
#13465=CARTESIAN_POINT ( 'NONE',  ( 23.87821517812500005, -4.985214923628404016, -4.040624999385455496 ) ) ;
#13468=CARTESIAN_POINT ( 'NONE',  ( 15.00000000000000178, -3.464101615137757051, -10.25624999877095966 ) ) ;
#13494=CARTESIAN_POINT ( 'NONE',  ( 15.00000000000000000, 0.000000000000000000, -1.743749998770943721 ) ) ;
#13495=DIRECTION ( 'NONE',  ( 0.08715574274765150453, 0.000000000000000000, 0.9961946980917461003 ) ) ;
#13504=CARTESIAN_POINT ( 'NONE',  ( 15.24356964374999990, 3.323476615752268604, -7.040624999385501681 ) ) ;
#13512=CARTESIAN_POINT ( 'NONE',  ( 31.41211527974097706, -7.209453229046482114, 169.0110222298289671 ) ) ;
#13519=CARTESIAN_POINT ( 'NONE',  ( 23.99999999999999645, 5.196152422706631135, -6.899999999999989697 ) ) ;
#13525=CARTESIAN_POINT ( 'NONE',  ( 21.00000000000000355, 0.000000000000000000, 50.00000000000001421 ) ) ;
#13538=EDGE_CURVE ( 'NONE', #24506, #17676, #20131, .T. ) ;
#13544=EDGE_LOOP ( 'NONE', ( #34434, #13183, #23862, #5719 ) ) ;
#13549=CARTESIAN_POINT ( 'NONE',  ( 33.99418380086066804, 5.407089921784857367, 162.7057366146619586 ) ) ;
#13550=CARTESIAN_POINT ( 'NONE',  ( 26.75643035624999655, -3.323476615752267715, -0.5156249993854836733 ) ) ;
#13556=CARTESIAN_POINT ( 'NONE',  ( 26.99999999999999645, 3.464101615137755275, -4.181249998770937282 ) ) ;
#13557=CARTESIAN_POINT ( 'NONE',  ( 18.12178482187500350, -4.985214923628407568, -0.9656249993854615354 ) ) ;
#13569=CARTESIAN_POINT ( 'NONE',  ( 27.92429219659289785, 5.196152422706630247, 163.5661617036773237 ) ) ;
#13571=EDGE_CURVE ( 'NONE', #8055, #26185, #28847, .T. ) ;
#13574=CARTESIAN_POINT ( 'NONE',  ( 20.99999999999999645, -6.646953231504538984, -1.040624999385473481 ) ) ;
#13584=CARTESIAN_POINT ( 'NONE',  ( 24.71512661192725702, -3.604726614523244610, 164.1010192074743657 ) ) ;
#13593=CARTESIAN_POINT ( 'NONE',  ( 27.00000000000047251, -3.464101615137475942, -3.412500000000007194 ) ) ;
#13602=ORIENTED_EDGE ( 'NONE', *, *, #17246, .F. ) ;
#13603=CARTESIAN_POINT ( 'NONE',  ( 26.99999999999999645, 7.347880794884117764E-16, -1.124999999999987121 ) ) ;
#13604=CARTESIAN_POINT ( 'NONE',  ( 23.73600959472706506, -5.270316205469181448, -7.999999999999998224 ) ) ;
#13605=CARTESIAN_POINT ( 'NONE',  ( 24.43731768191911513, 0.000000000000000000, 160.9256486073069539 ) ) ;
#13607=CARTESIAN_POINT ( 'NONE',  ( 27.84912036836594140, -5.196152422706638241, 162.7069437753488046 ) ) ;
#13608=( BOUNDED_CURVE ( )  B_SPLINE_CURVE ( 2, ( #22962, #11573, #31480, #34509, #14241, #17089, #5505 ),
 .UNSPECIFIED., .F., .F. ) 
 B_SPLINE_CURVE_WITH_KNOTS ( ( 3, 2, 2, 3 ),
 ( 0.4782608695652184050, 0.4855072463768126956, 0.4927536231884070417, 0.5000000000000013323 ),
 .UNSPECIFIED. ) 
 CURVE ( )  GEOMETRIC_REPRESENTATION_ITEM ( )  RATIONAL_B_SPLINE_CURVE ( ( 0.9999999999999815703, 0.8660254037844571373, 1.000000000000000000, 0.8660254037844387076, 1.000000000000000000, 0.8660254037844140607, 1.000000000000024647 ) ) 
 REPRESENTATION_ITEM ( '' )  );
#13614=EDGE_LOOP ( 'NONE', ( #20061, #17519, #32892, #4125 ) ) ;
#13615=VERTEX_POINT ( 'NONE', #29526 ) ;
#13619=CARTESIAN_POINT ( 'NONE',  ( 23.87821517812499650, 4.985214923628404904, -9.853124999385482141 ) ) ;
#13633=CARTESIAN_POINT ( 'NONE',  ( 37.09428426793671463, -3.604726614523235284, 162.3215832362777746 ) ) ;
#13637=CARTESIAN_POINT ( 'NONE',  ( 24.74287602148785581, 3.464101615137384904, 161.6235481623923249 ) ) ;
#13642=CARTESIAN_POINT ( 'NONE',  ( 34.13799077639428958, -5.407089921784855591, 164.3494578665133474 ) ) ;
#13643=CARTESIAN_POINT ( 'NONE',  ( 18.12178482187499640, 4.985214923628404904, -5.615624999385476990 ) ) ;
#13645=CARTESIAN_POINT ( 'NONE',  ( 16.07192114941521766, -3.422577806627481234, -8.000000000000001776 ) ) ;
#13646=CARTESIAN_POINT ( 'NONE',  ( 28.42434827050043467, 5.196152422706636465, 169.2818287827543600 ) ) ;
#13658=CARTESIAN_POINT ( 'NONE',  ( 18.12178482187499640, 4.985214923628404904, -4.715624999385465088 ) ) ;
#13661=CARTESIAN_POINT ( 'NONE',  ( 24.85399959338462139, 0.000000000000000000, 162.8936964012349051 ) ) ;
#13662=CARTESIAN_POINT ( 'NONE',  ( 21.00000000000000000, 6.646953231504538984, -2.165624999385510563 ) ) ;
#13665=ORIENTED_EDGE ( 'NONE', *, *, #9024, .F. ) ;
#13681=CARTESIAN_POINT ( 'NONE',  ( 21.00000000000000355, 0.000000000000000000, 50.00000000000001421 ) ) ;
#13686=ORIENTED_EDGE ( 'NONE', *, *, #22429, .T. ) ;
#13690=CARTESIAN_POINT ( 'NONE',  ( 27.00000000000052580, 3.464101615137448409, -2.887499999999997513 ) ) ;
#13694=CARTESIAN_POINT ( 'NONE',  ( 26.99999999999999645, 7.347880794884117764E-16, -8.775000000000005684 ) ) ;
#13700=CARTESIAN_POINT ( 'NONE',  ( 23.87821517812499650, 4.985214923628404904, -5.803124999385484095 ) ) ;
#13703=ORIENTED_EDGE ( 'NONE', *, *, #4266, .F. ) ;
#13705=CARTESIAN_POINT ( 'NONE',  ( 24.86380461455084756, 0.000000000000000000, 163.0057683059945930 ) ) ;
#13706=( BOUNDED_CURVE ( )  B_SPLINE_CURVE ( 2, ( #28027, #13637, #2060, #25187, #25370, #22353, #36740 ),
 .UNSPECIFIED., .F., .T. ) 
 B_SPLINE_CURVE_WITH_KNOTS ( ( 3, 2, 2, 3 ),
 ( 0.7826086956521726146, 0.7898550724637666276, 0.7971014492753608627, 0.8043478260869549867 ),
 .UNSPECIFIED. ) 
 CURVE ( )  GEOMETRIC_REPRESENTATION_ITEM ( )  RATIONAL_B_SPLINE_CURVE ( ( 1.000000000000024647, 0.8660254037844140607, 1.000000000000000000, 0.8660254037844387076, 1.000000000000000000, 0.8660254037844674624, 0.9999999999999712452 ) ) 
 REPRESENTATION_ITEM ( '' )  );
#13707=CARTESIAN_POINT ( 'NONE',  ( 25.22171936664797798, 0.000000000000000000, 169.8914008901326724 ) ) ;
#13718=CARTESIAN_POINT ( 'NONE',  ( 20.99999999999999645, -6.928203230275506996, -2.981249998770937992 ) ) ;
#13726=FACE_OUTER_BOUND ( 'NONE', #5340, .T. ) ;
#13727=ORIENTED_EDGE ( 'NONE', *, *, #33000, .T. ) ;
#13738=ORIENTED_EDGE ( 'NONE', *, *, #7478, .T. ) ;
#13745=CARTESIAN_POINT ( 'NONE',  ( 27.62402916835064559, 5.407089921784856479, 161.5314637101514279 ) ) ;
#13746=CARTESIAN_POINT ( 'NONE',  ( 21.00000000000000000, -6.646953231504538984, -0.5906249993854776337 ) ) ;
#13751=CARTESIAN_POINT ( 'NONE',  ( 26.99999999999999645, 3.464101615137755275, -3.731249998770941545 ) ) ;
#13752=CARTESIAN_POINT ( 'NONE',  ( 15.24356964374999990, 3.323476615752268604, -1.528124999385497729 ) ) ;
#13760=AXIS2_PLACEMENT_3D ( 'NONE', #10868, #21798, #12691 ) ;
#13761=CARTESIAN_POINT ( 'NONE',  ( 28.09424589495082714, -5.196152422706632912, 165.5087413649561938 ) ) ;
#13765=CARTESIAN_POINT ( 'NONE',  ( 26.75643035624999655, 7.049594010296217766E-16, -0.9281249993854934210 ) ) ;
#13774=FACE_OUTER_BOUND ( 'NONE', #12696, .T. ) ;
#13775=CARTESIAN_POINT ( 'NONE',  ( 37.21357869082257253, 3.604726614523243278, 163.6851247292908909 ) ) ;
#13782=EDGE_CURVE ( 'NONE', #36867, #12908, #3815, .T. ) ;
#13783=CARTESIAN_POINT ( 'NONE',  ( 15.00000000000000000, 0.000000000000000000, -5.793749998770941545 ) ) ;
#13786=LINE ( 'NONE', #11303, #18417 ) ;
#13790=ORIENTED_EDGE ( 'NONE', *, *, #7799, .T. ) ;
#13791=CARTESIAN_POINT ( 'NONE',  ( 26.99999999999999645, -3.464101615137751278, -3.412500000000012967 ) ) ;
#13793=CARTESIAN_POINT ( 'NONE',  ( 26.72225775819230975, -1.093967549749166102, -8.000000000000003553 ) ) ;
#13794=CARTESIAN_POINT ( 'NONE',  ( 33.85854767620964623, -5.407089921784861808, 161.1554086157566985 ) ) ;
#13796=CARTESIAN_POINT ( 'NONE',  ( 36.62857725106855611, -3.464101615137755275, 159.7931759234488425 ) ) ;
#13803=CARTESIAN_POINT ( 'NONE',  ( 15.00000000000000000, 0.000000000000000000, -0.9000000000000119016 ) ) ;
#13805=CARTESIAN_POINT ( 'NONE',  ( 18.12178482187499640, 4.985214923628404904, -9.778124999385489957 ) ) ;
#13809=EDGE_CURVE ( 'NONE', #19565, #32257, #32735, .T. ) ;
#13819=CARTESIAN_POINT ( 'NONE',  ( 27.74168942105997360, 5.407089921784856479, 162.8763265525752786 ) ) ;
#13822=DIRECTION ( 'NONE',  ( 0.000000000000000000, 0.000000000000000000, 1.000000000000000000 ) ) ;
#13830=CARTESIAN_POINT ( 'NONE',  ( 37.21521286099908110, 7.646167579472015790E-16, 163.7038033798800711 ) ) ;
#13832=CARTESIAN_POINT ( 'NONE',  ( 23.87821517812499650, 4.985214923628404904, -4.790624999385456384 ) ) ;
#13834=CARTESIAN_POINT ( 'NONE',  ( 37.44889919624123564, 3.604726614523243278, 166.3748504141385638 ) ) ;
#13835=CARTESIAN_POINT ( 'NONE',  ( 25.24946877610209128, -3.464101615137761048, 167.4139298438261960 ) ) ;
#13838=CARTESIAN_POINT ( 'NONE',  ( 15.02283181144952628, 7.347880794884122694E-16, 50.52293445648592751 ) ) ;
#13844=CARTESIAN_POINT ( 'NONE',  ( 26.99999999999999645, 7.347880794884117764E-16, -1.518749998770940746 ) ) ;
#13845=CARTESIAN_POINT ( 'NONE',  ( 15.24356964375000167, -3.323476615752272600, -4.603124999385474148 ) ) ;
#13848=CARTESIAN_POINT ( 'NONE',  ( 15.24356964374999990, 0.000000000000000000, -2.953124999385492444 ) ) ;
#13870=LINE ( 'NONE', #1736, #17950 ) ;
#13875=CARTESIAN_POINT ( 'NONE',  ( 15.00000000000039613, 3.464101615137982204, -2.737500000000008260 ) ) ;
#13881=CARTESIAN_POINT ( 'NONE',  ( 15.00000000000000000, 3.464101615137752166, -9.037500000000006750 ) ) ;
#13886=CARTESIAN_POINT ( 'NONE',  ( 15.24356964375000167, -3.323476615752272600, -6.965624999385507721 ) ) ;
#13892=CARTESIAN_POINT ( 'NONE',  ( 34.42070221693199272, 5.407089921784862696, 167.5808644184484706 ) ) ;
#13894=CARTESIAN_POINT ( 'NONE',  ( 31.39985900347063819, -6.928203230275506996, 168.8709323510219917 ) ) ;
#13908=DIRECTION ( 'NONE',  ( 0.000000000000000000, 0.000000000000000000, 1.000000000000000000 ) ) ;
#13916=CARTESIAN_POINT ( 'NONE',  ( 37.06980319883601283, -3.464101615137536783, 164.8364115837626684 ) ) ;
#13926=CARTESIAN_POINT ( 'NONE',  ( 24.67427235751429393, 3.604726614523236616, 163.6340529427438639 ) ) ;
#13931=VERTEX_POINT ( 'NONE', #21645 ) ;
#13934=CARTESIAN_POINT ( 'NONE',  ( 15.00000000000000178, -3.464101615137757051, -5.306249998770942611 ) ) ;
#13935=CARTESIAN_POINT ( 'NONE',  ( 20.99999999999999645, -6.646953231504538984, -3.178124999385461003 ) ) ;
#13944=CARTESIAN_POINT ( 'NONE',  ( 24.98146486726017912, 0.000000000000000000, 164.3506311484184437 ) ) ;
#13949=CARTESIAN_POINT ( 'NONE',  ( 23.87821517812500005, -4.985214923628404016, -1.453124999385491112 ) ) ;
#13953=VERTEX_POINT ( 'NONE', #10628 ) ;
#13957=CARTESIAN_POINT ( 'NONE',  ( 36.97498984505087805, 7.646167579472024665E-16, 160.9580417432647153 ) ) ;
#13971=VERTEX_POINT ( 'NONE', #19185 ) ;
#13972=CARTESIAN_POINT ( 'NONE',  ( 21.00000000000000000, -6.928203230275506996, -4.387499999999998401 ) ) ;
#13973=CARTESIAN_POINT ( 'NONE',  ( 21.00000000000000355, 0.000000000000000000, 50.00000000000001421 ) ) ;
#13974=CARTESIAN_POINT ( 'NONE',  ( 33.81932759197320593, -5.407089921784861808, 160.7071210016154055 ) ) ;
#13976=CARTESIAN_POINT ( 'NONE',  ( 37.64336544724691436, -3.604726614523235284, 168.5976098342557918 ) ) ;
#13984=CARTESIAN_POINT ( 'NONE',  ( 26.75643035624999655, 7.049594010296217766E-16, -8.578124999385483562 ) ) ;
#13989=CARTESIAN_POINT ( 'NONE',  ( 37.05016167317072728, -3.604726614523238837, 161.8172596703688555 ) ) ;
#13998=CARTESIAN_POINT ( 'NONE',  ( 26.99999999999967670, 3.464101615137938683, -1.931249998770954823 ) ) ;
#13999=CARTESIAN_POINT ( 'NONE',  ( 24.44222019244867283, 0.000000000000000000, 160.9816845590745800 ) ) ;
#14000=CARTESIAN_POINT ( 'NONE',  ( 21.00000000000000000, 6.928203230275506996, -0.5062499987709455640 ) ) ;
#14011=CARTESIAN_POINT ( 'NONE',  ( 24.48470861703815515, -3.604726614523240613, 161.4673294743943188 ) ) ;
#14012=CARTESIAN_POINT ( 'NONE',  ( 18.12178482187499640, 4.985214923628404904, -8.765624999385462246 ) ) ;
#14015=CARTESIAN_POINT ( 'NONE',  ( 31.33367511126808935, -7.209453229046482114, 168.1144470015463810 ) ) ;
#14016=CARTESIAN_POINT ( 'NONE',  ( 37.09921826190588234, -3.464101615137755275, 165.1726272931442452 ) ) ;
#14024=VERTEX_POINT ( 'NONE', #33818 ) ;
#14026=DIRECTION ( 'NONE',  ( 0.000000000000000000, 0.000000000000000000, 1.000000000000000000 ) ) ;
#14029=CARTESIAN_POINT ( 'NONE',  ( 26.75643035624999655, 7.049594010296217766E-16, -1.828124999385477567 ) ) ;
#14051=CARTESIAN_POINT ( 'NONE',  ( 24.90302469878729141, 0.000000000000000000, 163.4540559201358576 ) ) ;
#14057=EDGE_CURVE ( 'NONE', #4178, #5932, #18711, .T. ) ;
#14063=CARTESIAN_POINT ( 'NONE',  ( 26.99999999999999645, -3.464101615137751278, -9.712500000000016342 ) ) ;
#14068=CARTESIAN_POINT ( 'NONE',  ( 26.75643035624999655, 3.323476615752271712, -8.990624999385502747 ) ) ;
#14073=CARTESIAN_POINT ( 'NONE',  ( 28.02440086159767674, -5.407089921784865361, 166.1077331045103733 ) ) ;
#14080=CARTESIAN_POINT ( 'NONE',  ( 34.50404489593442747, 5.407089921784857367, 168.5334755984986828 ) ) ;
#14082=DIRECTION ( 'NONE',  ( 0.08715574274765150453, 0.000000000000000000, 0.9961946980917461003 ) ) ;
#14083=CARTESIAN_POINT ( 'NONE',  ( 14.99999999999941380, -3.464101615137419543, -7.162500000000004974 ) ) ;
#14108=CARTESIAN_POINT ( 'NONE',  ( 37.05833252405330569, 7.646167579472015790E-16, 161.9106529233149274 ) ) ;
#14109=CARTESIAN_POINT ( 'NONE',  ( 18.12178482187499640, 4.985214923628404904, -0.3281249993854762348 ) ) ;
#14113=EDGE_LOOP ( 'NONE', ( #34477, #29010, #3098, #16351 ) ) ;
#14114=CARTESIAN_POINT ( 'NONE',  ( 18.00000000000000355, -5.196152422706632912, -8.418749998770957532 ) ) ;
#14115=CARTESIAN_POINT ( 'NONE',  ( 15.24356964375000167, -3.323476615752272600, -1.903124999385467753 ) ) ;
#14117=CARTESIAN_POINT ( 'NONE',  ( 25.28868886033866659, -3.464101615137837431, 167.8622174579674606 ) ) ;
#14125=CARTESIAN_POINT ( 'NONE',  ( 36.91619120224290640, 7.347880794884117764E-16, 163.0806184283759706 ) ) ;
#14130=CARTESIAN_POINT ( 'NONE',  ( 18.12178482187499640, 4.985214923628404904, -3.928124999385496086 ) ) ;
#14140=CARTESIAN_POINT ( 'NONE',  ( 30.78459393195788607, -7.209453229046482114, 161.8384204035683922 ) ) ;
#14145=CARTESIAN_POINT ( 'NONE',  ( 20.99999999999999645, 6.928203230275506996, -4.162500000000016520 ) ) ;
#14152=ORIENTED_EDGE ( 'NONE', *, *, #23212, .F. ) ;
#14153=CARTESIAN_POINT ( 'NONE',  ( 15.00000000000000178, -3.464101615137757051, -4.912499999999988098 ) ) ;
#14154=DIRECTION ( 'NONE',  ( 0.9961946980917462113, 0.000000000000000000, -0.08715574274765118534 ) ) ;
#14155=CARTESIAN_POINT ( 'NONE',  ( 36.97172150469784668, -3.604726614523238837, 160.9206844420862694 ) ) ;
#14157=CARTESIAN_POINT ( 'NONE',  ( 28.22540379330944660, -5.407089921784859143, 168.4052071269844930 ) ) ;
#14159=CYLINDRICAL_SURFACE ( 'NONE', #4547, 5.999999999999994671 ) ;
#14162=VERTEX_POINT ( 'NONE', #20538 ) ;
#14167=CARTESIAN_POINT ( 'NONE',  ( 18.12178482187499640, 4.985214923628404904, -8.878124999385478944 ) ) ;
#14169=( BOUNDED_CURVE ( )  B_SPLINE_CURVE ( 2, ( #30619, #8052, #34381, #31174, #24917, #1978, #10510 ),
 .UNSPECIFIED., .F., .F. ) 
 B_SPLINE_CURVE_WITH_KNOTS ( ( 3, 2, 2, 3 ),
 ( 0.5869565217391291556, 0.5942028985507233907, 0.6014492753623178478, 0.6086956521739121939 ),
 .UNSPECIFIED. ) 
 CURVE ( )  GEOMETRIC_REPRESENTATION_ITEM ( )  RATIONAL_B_SPLINE_CURVE ( ( 1.000000000000024647, 0.8660254037844140607, 1.000000000000000000, 0.8660254037844387076, 1.000000000000000000, 0.8660254037844551389, 0.9999999999999835687 ) ) 
 REPRESENTATION_ITEM ( '' )  );
#14171=DIRECTION ( 'NONE',  ( 0.9961946980917462113, 0.000000000000000000, -0.08715574274765118534 ) ) ;
#14172=CARTESIAN_POINT ( 'NONE',  ( 37.01420992928731835, 7.646167579472024665E-16, 161.4063293574060083 ) ) ;
#14174=SURFACE_STYLE_FILL_AREA ( #11329 ) ;
#14175=CARTESIAN_POINT ( 'NONE',  ( 23.35209618661503583, 3.999999999999908962, 50.00000000000000000 ) ) ;
#14180=ORIENTED_EDGE ( 'NONE', *, *, #4835, .F. ) ;
#14182=CARTESIAN_POINT ( 'NONE',  ( 28.31649303895732928, 5.196152422706630247, 168.0490378450901687 ) ) ;
#14184=ADVANCED_FACE ( 'NONE', ( #14282 ), #37381, .T. ) ;
#14186=CARTESIAN_POINT ( 'NONE',  ( 25.14654753852813229, -3.604726614523244610, 169.0321829630285322 ) ) ;
#14187=CARTESIAN_POINT ( 'NONE',  ( 26.99999999999999645, -3.464101615137751278, -1.556249998770957044 ) ) ;
#14196=CARTESIAN_POINT ( 'NONE',  ( 37.01584409946383403, -3.604726614523235284, 161.4250080079951886 ) ) ;
#14197=CARTESIAN_POINT ( 'NONE',  ( 23.87821517812500005, -4.985214923628404016, -7.190624999385470062 ) ) ;
#14199=CARTESIAN_POINT ( 'NONE',  ( 25.14327919817509027, 0.000000000000000000, 168.9948256618500864 ) ) ;
#14200=CARTESIAN_POINT ( 'NONE',  ( 34.14658591151403755, -5.196152422706635576, 165.8450248343500562 ) ) ;
#14210=( BOUNDED_CURVE ( )  B_SPLINE_CURVE ( 2, ( #2943, #35333, #31756, #9389, #20963, #29276, #32496 ),
 .UNSPECIFIED., .F., .F. ) 
 B_SPLINE_CURVE_WITH_KNOTS ( ( 3, 2, 2, 3 ),
 ( 0.08695652173913033522, 0.09420289855072437601, 0.1014492753623184307, 0.1086956521739124576 ),
 .UNSPECIFIED. ) 
 CURVE ( )  GEOMETRIC_REPRESENTATION_ITEM ( )  RATIONAL_B_SPLINE_CURVE ( ( 1.000000000000001776, 0.8660254037844368202, 1.000000000000000000, 0.8660254037844387076, 1.000000000000000000, 0.8660254037844494768, 0.9999999999999892308 ) ) 
 REPRESENTATION_ITEM ( '' )  );
#14212=CARTESIAN_POINT ( 'NONE',  ( 18.00000000000000355, -5.196152422706632912, -2.624999999999988454 ) ) ;
#14215=CARTESIAN_POINT ( 'NONE',  ( 18.12178482187500350, -4.985214923628407568, -1.078124999385476901 ) ) ;
#14220=CARTESIAN_POINT ( 'NONE',  ( 26.99999999999946354, -3.464101615138058143, -2.962500000000024336 ) ) ;
#14227=CARTESIAN_POINT ( 'NONE',  ( 23.34314575050772333, 3.999999999999902744, 49.89769604716121876 ) ) ;
#14237=CARTESIAN_POINT ( 'NONE',  ( 34.49097153452227360, -5.407089921784855591, 168.3840463937848995 ) ) ;
#14240=CARTESIAN_POINT ( 'NONE',  ( 23.87821517812499650, 4.985214923628404904, -0.7406249993854585600 ) ) ;
#14241=CARTESIAN_POINT ( 'NONE',  ( 23.99999999999999645, 5.196152422706631135, -5.099999999999993427 ) ) ;
#14244=EDGE_CURVE ( 'NONE', #11807, #23273, #15811, .T. ) ;
#14249=ORIENTED_EDGE ( 'NONE', *, *, #12641, .F. ) ;
#14253=CARTESIAN_POINT ( 'NONE',  ( 21.00000000000000000, 6.646953231504538984, -8.465624999385484628 ) ) ;
#14255=ORIENTED_EDGE ( 'NONE', *, *, #18908, .F. ) ;
#14259=CARTESIAN_POINT ( 'NONE',  ( 37.32470226282583781, -3.604726614523238837, 164.9552729693578215 ) ) ;
#14263=EDGE_CURVE ( 'NONE', #8199, #17429, #34401, .T. ) ;
#14267=CARTESIAN_POINT ( 'NONE',  ( 28.30384396178233075, -5.407089921784859143, 169.3017823552670507 ) ) ;
#14270=CARTESIAN_POINT ( 'NONE',  ( 25.32137226386879902, 3.464101615137695767, 168.2357904697519473 ) ) ;
#14280=CYLINDRICAL_SURFACE ( 'NONE', #18049, 6.000000000000001776 ) ;
#14282=FACE_OUTER_BOUND ( 'NONE', #24556, .T. ) ;
#14294=CARTESIAN_POINT ( 'NONE',  ( 33.94189035521207387, -5.407089921784855591, 162.1080197958069107 ) ) ;
#14295=CARTESIAN_POINT ( 'NONE',  ( 15.24356964374999990, 0.000000000000000000, -2.953124999385492444 ) ) ;
#14301=CARTESIAN_POINT ( 'NONE',  ( 18.00000000000000000, 5.196152422706630247, -6.768749998770945631 ) ) ;
#14302=CARTESIAN_POINT ( 'NONE',  ( 15.24356964374999990, 3.323476615752268604, -3.328124999385480898 ) ) ;
#14303=CARTESIAN_POINT ( 'NONE',  ( 26.99999999999999645, 7.347880794884117764E-16, -6.525000000000003020 ) ) ;
#14310=CARTESIAN_POINT ( 'NONE',  ( 33.77726345172796840, 5.196152422706631135, 161.6236498024106822 ) ) ;
#14315=CARTESIAN_POINT ( 'NONE',  ( 15.24356964375000167, -3.323476615752272600, -4.715624999385497063 ) ) ;
#14320=CARTESIAN_POINT ( 'NONE',  ( 24.94224478302373527, 0.000000000000000000, 163.9023435342771506 ) ) ;
#14323=DIRECTION ( 'NONE',  ( 0.000000000000000000, 0.000000000000000000, 1.000000000000000000 ) ) ;
#14324=CARTESIAN_POINT ( 'NONE',  ( 24.63341810310133084, 0.000000000000000000, 163.1670866780133906 ) ) ;
#14330=CARTESIAN_POINT ( 'NONE',  ( 20.99999999999999645, 0.000000000000000000, 50.00000000000000000 ) ) ;
#14333=CARTESIAN_POINT ( 'NONE',  ( 15.00000000000000000, 0.000000000000000000, -3.543749998770939769 ) ) ;
#14337=CARTESIAN_POINT ( 'NONE',  ( 15.00000000000000000, 0.000000000000000000, -4.950000000000009948 ) ) ;
#14338=DIRECTION ( 'NONE',  ( 1.000000000000000000, 0.000000000000000000, 0.000000000000000000 ) ) ;
#14340=CARTESIAN_POINT ( 'NONE',  ( 27.55375985076035761, -5.407089921784865361, 160.7282817348149706 ) ) ;
#14342=CARTESIAN_POINT ( 'NONE',  ( 28.51246584124881167, 5.725134610794655465, 159.7765254813093350 ) ) ;
#14345=EDGE_CURVE ( 'NONE', #30675, #37490, #733, .T. ) ;
#14351=DIRECTION ( 'NONE',  ( 0.08715574274764675833, 0.000000000000000000, 0.9961946980917465444 ) ) ;
#14354=DIRECTION ( 'NONE',  ( 0.9961946980917462113, 0.000000000000000000, -0.08715574274765118534 ) ) ;
#14359=CARTESIAN_POINT ( 'NONE',  ( 33.83240095338533848, 5.407089921784862696, 160.8565502063291603 ) ) ;
#14365=VERTEX_POINT ( 'NONE', #12373 ) ;
#14370=CARTESIAN_POINT ( 'NONE',  ( 25.14327919817509027, 0.000000000000000000, 168.9948256618500864 ) ) ;
#14371=CARTESIAN_POINT ( 'NONE',  ( 23.99999999999999645, 5.196152422706631135, -2.343749998770960907 ) ) ;
#14376=DIRECTION ( 'NONE',  ( 0.08715574274765150453, 0.000000000000000000, 0.9961946980917461003 ) ) ;
#14378=ORIENTED_EDGE ( 'NONE', *, *, #12185, .F. ) ;
#14379=CARTESIAN_POINT ( 'NONE',  ( 27.79398286670857132, -5.407089921784859143, 163.4740433714303265 ) ) ;
#14380=CARTESIAN_POINT ( 'NONE',  ( 21.00000000000000000, 6.646953231504538984, -7.003124999385472726 ) ) ;
#14382=CARTESIAN_POINT ( 'NONE',  ( 37.48485094012463748, 7.646167579472024665E-16, 166.7857807271014394 ) ) ;
#14383=CARTESIAN_POINT ( 'NONE',  ( 37.14497502684837826, 3.464101615137759271, 165.6956295096424299 ) ) ;
#14391=VERTEX_POINT ( 'NONE', #30188 ) ;
#14394=CARTESIAN_POINT ( 'NONE',  ( 26.99999999999976197, -3.464101615137889834, -2.512499999999992628 ) ) ;
#14396=CARTESIAN_POINT ( 'NONE',  ( 23.87821517812500005, -4.985214923628404016, -2.353124999385475036 ) ) ;
#14410=AXIS2_PLACEMENT_3D ( 'NONE', #29801, #3835, #24130 ) ;
#14413=DIRECTION ( 'NONE',  ( 0.08715574274765150453, 0.000000000000000000, 0.9961946980917461003 ) ) ;
#14416=CARTESIAN_POINT ( 'NONE',  ( 33.85570362020085611, 5.196152422706631135, 162.5202250306932399 ) ) ;
#14418=CARTESIAN_POINT ( 'NONE',  ( 37.57146195948011069, 3.604726614523238837, 167.7757492083300690 ) ) ;
#14420=( BOUNDED_CURVE ( )  B_SPLINE_CURVE ( 2, ( #15080, #29665, #12610, #27383, #23993, #21156, #15460 ),
 .UNSPECIFIED., .F., .F. ) 
 B_SPLINE_CURVE_WITH_KNOTS ( ( 3, 2, 2, 3 ),
 ( 0.4130434782608697342, 0.4202898550724640248, 0.4275362318840583153, 0.4347826086956526059 ),
 .UNSPECIFIED. ) 
 CURVE ( )  GEOMETRIC_REPRESENTATION_ITEM ( )  RATIONAL_B_SPLINE_CURVE ( ( 0.9999999999999968914, 0.8660254037844418162, 1.000000000000000000, 0.8660254037844387076, 1.000000000000000000, 0.8660254037844304920, 1.000000000000008216 ) ) 
 REPRESENTATION_ITEM ( '' )  );
#14421=CARTESIAN_POINT ( 'NONE',  ( 21.00000000000000355, 0.000000000000000000, 50.00000000000001421 ) ) ;
#14427=CLOSED_SHELL ( 'NONE', ( #2736, #20332, #27945, #1359, #30209, #16354, #31709, #15672, #5903, #20150, #14665, #2887, #27519, #1763, #4292, #33464, #3539, #6864, #6608, #6935, #16660, #14464, #14927, #27932, #29080, #26315, #18772, #36037, #28781, #29607, #27662, #3415, #18545, #25118, #2519, #35997, #36575, #23162, #10614, #33764, #22857, #7558, #14184, #33048, #15222, #1718, #6153, #29167, #16117, #21757, #14509, #35067, #12384, #12287, #23127, #5981, #32600, #7066, #21420, #13174, #5488, #20307, #31352, #29870, #13075, #4542, #30497, #12272, #26735, #6172, #17476, #14730, #36725, #33751, #17858, #22061, #9835, #37139, #23624, #14447, #27559, #35329, #2474, #25240, #14689, #30892, #21074, #24201, #3519, #17262, #7878, #19922, #11936, #36997, #20346, #32790, #15404, #5625, #20608, #32521, #2404, #24785, #15966 ) ) ;
#14435=CARTESIAN_POINT ( 'NONE',  ( 26.75643035624999655, 7.049594010296217766E-16, -0.3656249993854721048 ) ) ;
#14437=EDGE_LOOP ( 'NONE', ( #4581, #34907, #16592, #12146 ) ) ;
#14440=CARTESIAN_POINT ( 'NONE',  ( 34.28996860281051795, -5.407089921784861808, 166.0865723713108366 ) ) ;
#14447=ADVANCED_FACE ( 'NONE', ( #26770 ), #18074, .T. ) ;
#14448=CARTESIAN_POINT ( 'NONE',  ( 31.41701779027052766, -7.209453229046475009, 169.0670581815966216 ) ) ;
#14450=CARTESIAN_POINT ( 'NONE',  ( 15.00000000000000000, 3.464101615137752610, -0.4312499987709516591 ) ) ;
#14456=EDGE_CURVE ( 'NONE', #7551, #22746, #4612, .T. ) ;
#14461=CARTESIAN_POINT ( 'NONE',  ( 37.26917196037089042, 7.347880794884117764E-16, 167.1152069556475510 ) ) ;
#14463=CARTESIAN_POINT ( 'NONE',  ( 15.02283181144952628, 7.347880794884122694E-16, 50.52293445648592751 ) ) ;
#14464=ADVANCED_FACE ( 'NONE', ( #17881 ), #29616, .T. ) ;
#14471=CARTESIAN_POINT ( 'NONE',  ( 37.11229162342512211, 7.347880794884117764E-16, 165.3220564990824073 ) ) ;
#14477=CARTESIAN_POINT ( 'NONE',  ( 27.54558899987776144, 5.407089921784856479, 160.6348884818688418 ) ) ;
#14478=CARTESIAN_POINT ( 'NONE',  ( 15.24356964374999990, 0.000000000000000000, -1.153124999385496396 ) ) ;
#14484=CARTESIAN_POINT ( 'NONE',  ( 15.00000000000000178, -3.464101615137757051, -7.106249998770957532 ) ) ;
#14485=CARTESIAN_POINT ( 'NONE',  ( 26.75643035624999655, 7.049594010296217766E-16, -5.765624999385460470 ) ) ;
#14491=CARTESIAN_POINT ( 'NONE',  ( 33.88185034302515675, -5.196152422706629359, 162.8190834401207496 ) ) ;
#14495=CARTESIAN_POINT ( 'NONE',  ( 20.99999999999999645, -6.646953231504538984, -3.740624999385479654 ) ) ;
#14496=LINE ( 'NONE', #23591, #8329 ) ;
#14506=CARTESIAN_POINT ( 'NONE',  ( 30.72576380560321851, 7.209453229046482114, 161.1659889823564811 ) ) ;
#14509=ADVANCED_FACE ( 'NONE', ( #35485 ), #15600, .T. ) ;
#14516=CARTESIAN_POINT ( 'NONE',  ( 20.99999999999999645, 6.928203230275506996, -3.656249998770947585 ) ) ;
#14520=CARTESIAN_POINT ( 'NONE',  ( 18.00000000000000355, -5.196152422706632912, -5.324999999999996625 ) ) ;
#14522=CARTESIAN_POINT ( 'NONE',  ( 36.88023945835897166, 3.464101615138061696, 162.6696881154131802 ) ) ;
#14524=CARTESIAN_POINT ( 'NONE',  ( 34.34716455898865206, 5.407089921784857367, 166.7403251419335390 ) ) ;
#14526=CARTESIAN_POINT ( 'NONE',  ( 15.00000000000000000, 0.000000000000000000, -0.8437499987709595750 ) ) ;
#14530=CARTESIAN_POINT ( 'NONE',  ( 36.59916218799779841, -3.464101615138058143, 159.4569602140672657 ) ) ;
#14532=CARTESIAN_POINT ( 'NONE',  ( 36.74623750377856624, -3.464101615137356927, 161.1380387658726931 ) ) ;
#14533=CARTESIAN_POINT ( 'NONE',  ( 15.24356964374999990, 3.323476615752268604, -6.928124999385478766 ) ) ;
#14537=CARTESIAN_POINT ( 'NONE',  ( 26.99999999999999645, 7.347880794884117764E-16, -4.218749998770948473 ) ) ;
#14538=CARTESIAN_POINT ( 'NONE',  ( 25.20371201115935733, 3.464101615137634038, 166.8909276273280398 ) ) ;
#14540=DIRECTION ( 'NONE',  ( 0.08715574274765150453, 0.000000000000000000, 0.9961946980917461003 ) ) ;
#14541=CARTESIAN_POINT ( 'NONE',  ( 25.44883753774445978, 3.464101615137752166, 169.6927252169354290 ) ) ;
#14554=CARTESIAN_POINT ( 'NONE',  ( 27.48022219281702405, -5.407089921784859143, 159.8877424583000391 ) ) ;
#14555=CARTESIAN_POINT ( 'NONE',  ( 21.00000000000000000, 6.928203230275506996, -2.306249998770960374 ) ) ;
#14560=CYLINDRICAL_SURFACE ( 'NONE', #12832, 6.000000000000001776 ) ;
#14561=CARTESIAN_POINT ( 'NONE',  ( 27.47391033735120303, 4.898587196589416773E-16, 169.8919867420001992 ) ) ;
#14566=CARTESIAN_POINT ( 'NONE',  ( 33.83730346391489263, 5.407089921784857367, 160.9125861580968149 ) ) ;
#14567=CARTESIAN_POINT ( 'NONE',  ( 21.00000000000000000, -6.646953231504538984, -7.228124999385454608 ) ) ;
#14569=CARTESIAN_POINT ( 'NONE',  ( 34.48606902399273366, -5.407089921784861808, 168.3280104420172449 ) ) ;
#14570=CARTESIAN_POINT ( 'NONE',  ( 34.15965927292618431, 5.196152422706637353, 165.9944540390638679 ) ) ;
#14582=CARTESIAN_POINT ( 'NONE',  ( 18.12178482187499640, 4.985214923628404904, -3.028124999385484184 ) ) ;
#14587=( BOUNDED_CURVE ( )  B_SPLINE_CURVE ( 2, ( #6878, #30887, #21487, #33027, #33729, #9533, #16491, #28039, #2071, #6499, #29615, #15220, #26769, #23941, #5843, #31077, #5651, #25940, #28961, #16865, #14569, #31442, #31623, #17234, #14199, #33913, #17421, #22924, #22548, #37303, #8147, #25750, #2441, #14015, #31806, #28226, #8693, #28402, #2255, #31259, #2999, #20079, #20267, #19530, #5465, #5100, #34287, #37117, #28772, #36930, #7955, #34097, #17047, #34469, #14382, #8512, #16679, #11353, #28585, #5285, #2623, #2812, #23105, #37483, #8331, #13834, #11534, #22738, #10977, #34649, #19901, #26121, #11718, #153, #25381, #19719, #25565, #11165, #17793, #32370, #27068, #6220, #15320, #24041, #35393, #29712, #3937, #35587, #12473, #23292, #12281, #9632, #20455, #29336, #29142, #32186, #902, #31997, #18359, #20639, #21209, #522, #3374, #34837, #18172, #9442, #11905, #6026, #21020, #32748, #9256, #32556, #3566, #6597, #3746, #14943, #6785, #35025, #29908, #26679, #20829, #9069, #6409, #26303, #23855, #26490, #26872, #15512, #17612, #23472, #12089, #1092, #23663, #8877, #35207, #3183, #14759, #17983, #340, #29527, #15129, #710, #10563, #24229, #4313, #22140, #16265, #24598, #32935, #4873, #4502, #30099, #33686, #19310, #18746, #1658, #16452, #27996, #10378, #24961, #13232, #4131, #27628, #24781, #13413, #19116, #6989, #36148, #35964, #7173, #27815, #1277, #1469, #16079, #21953, #13043, #36332, #30288, #1843, #30848, #33499, #18557, #36519, #10002, #15703, #7544, #30666, #27254, #12848, #30482, #4684, #24416, #21583, #10191, #33130, #15892, #7727, #27437, #21767, #12661, #35773, #7357, #9817, #33317, #21394, #18929, #22877, #20218, #2028, #2212, #37442, #14155, #13794, #25524, #31216, #36890, #34244, #25341, #11123, #16640, #22700, #8649, #8103, #8286, #13974, #5058, #33874, #19859, #28543, #37077, #22322, #10936, #22510, #31581, #2767, #25709, #8465, #31764, #14340, #28729, #13605, #25894, #36710, #34057, #7916, #19677, #17189, #10749, #34606, #5245, #11491, #31402, #5421, #5604, #28181, #37262, #20035, #17002, #11309, #23060, #34428, #5795, #2585, #17375, #25155, #16822, #19490, #28364, #31036 ),
 .UNSPECIFIED., .F., .F. ) 
 B_SPLINE_CURVE_WITH_KNOTS ( ( 3, 2, 2, 2, 2, 2, 2, 2, 2, 2, 2, 2, 2, 2, 2, 2, 2, 2, 2, 2, 2, 2, 2, 2, 2, 2, 2, 2, 2, 2, 2, 2, 2, 2, 2, 2, 2, 2, 2, 2, 2, 2, 2, 2, 2, 2, 2, 2, 2, 2, 2, 2, 2, 2, 2, 2, 2, 2, 2, 2, 2, 2, 2, 2, 2, 2, 2, 2, 2, 2, 2, 2, 2, 2, 2, 2, 2, 2, 2, 2, 2, 2, 2, 2, 2, 2, 2, 2, 2, 2, 2, 2, 2, 2, 2, 2, 2, 2, 2, 2, 2, 2, 2, 2, 2, 2, 2, 2, 2, 2, 2, 2, 2, 2, 2, 2, 2, 2, 2, 2, 2, 2, 2, 2, 2, 2, 2, 2, 2, 2, 2, 2, 2, 2, 3 ),
 ( 0.000000000000000000, 0.007246376811594202987, 0.01449275362318840597, 0.02173913043478260809, 0.02898550724637681195, 0.03623188405797101580, 0.04347826086956521618, 0.05072463768115942351, 0.05797101449275362389, 0.06521739130434782428, 0.07246376811594203160, 0.07971014492753622505, 0.08695652173913043237, 0.09420289855072463969, 0.1014492753623188470, 0.1086956521739130405, 0.1159420289855072478, 0.1231884057971014551, 0.1304347826086956486, 0.1376811594202898559, 0.1449275362318840632, 0.1521739130434782705, 0.1594202898550724501, 0.1666666666666666574, 0.1739130434782608647, 0.1811594202898550721, 0.1884057971014492794, 0.1956521739130434867, 0.2028985507246376940, 0.2101449275362318736, 0.2173913043478260809, 0.2246376811594202882, 0.2318840579710144956, 0.2391304347826087029, 0.2463768115942029102, 0.2536231884057971175, 0.2608695652173912971, 0.2681159420289855322, 0.2753623188405797118, 0.2826086956521738913, 0.2898550724637681264, 0.2971014492753623060, 0.3043478260869565410, 0.3115942028985507206, 0.3188405797101449002, 0.3260869565217391353, 0.3333333333333333148, 0.3405797101449275499, 0.3478260869565217295, 0.3550724637681159646, 0.3623188405797101441, 0.3695652173913043237, 0.3768115942028985588, 0.3840579710144927383, 0.3913043478260869734, 0.3985507246376811530, 0.4057971014492753881, 0.4130434782608695676, 0.4202898550724637472, 0.4275362318840579823, 0.4347826086956521618, 0.4420289855072463969, 0.4492753623188405765, 0.4565217391304347561, 0.4637681159420289911, 0.4710144927536231707, 0.4782608695652174058, 0.4855072463768115854, 0.4927536231884058204, 0.5000000000000000000, 0.5072463768115942351, 0.5144927536231883591, 0.5217391304347825942, 0.5289855072463768293, 0.5362318840579710644, 0.5434782608695651884, 0.5507246376811594235, 0.5579710144927536586, 0.5652173913043477826, 0.5724637681159420177, 0.5797101449275362528, 0.5869565217391304879, 0.5942028985507246119, 0.6014492753623188470, 0.6086956521739130821, 0.6159420289855072062, 0.6231884057971014412, 0.6304347826086956763, 0.6376811594202898004, 0.6449275362318840354, 0.6521739130434782705, 0.6594202898550725056, 0.6666666666666666297, 0.6739130434782608647, 0.6811594202898550998, 0.6884057971014492239, 0.6956521739130434590, 0.7028985507246376940, 0.7101449275362319291, 0.7173913043478260532, 0.7246376811594202882, 0.7318840579710145233, 0.7391304347826086474, 0.7463768115942028825, 0.7536231884057971175, 0.7608695652173913526, 0.7681159420289854767, 0.7753623188405797118, 0.7826086956521739468, 0.7898550724637680709, 0.7971014492753623060, 0.8043478260869565410, 0.8115942028985507761, 0.8188405797101449002, 0.8260869565217391353, 0.8333333333333333703, 0.8405797101449274944, 0.8478260869565217295, 0.8550724637681159646, 0.8623188405797101996, 0.8695652173913043237, 0.8768115942028985588, 0.8840579710144927938, 0.8913043478260869179, 0.8985507246376811530, 0.9057971014492753881, 0.9130434782608695121, 0.9202898550724637472, 0.9275362318840579823, 0.9347826086956522174, 0.9420289855072463414, 0.9492753623188405765, 0.9565217391304348116, 0.9637681159420289356, 0.9662082893573751274 ),
 .UNSPECIFIED. ) 
 CURVE ( )  GEOMETRIC_REPRESENTATION_ITEM ( )  RATIONAL_B_SPLINE_CURVE ( ( 1.000000000000000000, 0.8660254037844387076, 1.000000000000000000, 0.8660254037844387076, 1.000000000000000000, 0.8660254037844387076, 1.000000000000000000, 0.8660254037844387076, 1.000000000000000000, 0.8660254037844387076, 1.000000000000000000, 0.8660254037844387076, 1.000000000000000000, 0.8660254037844387076, 1.000000000000000000, 0.8660254037844387076, 1.000000000000000000, 0.8660254037844387076, 1.000000000000000000, 0.8660254037844387076, 1.000000000000000000, 0.8660254037844387076, 1.000000000000000000, 0.8660254037844387076, 1.000000000000000000, 0.8660254037844387076, 1.000000000000000000, 0.8660254037844387076, 1.000000000000000000, 0.8660254037844387076, 1.000000000000000000, 0.8660254037844387076, 1.000000000000000000, 0.8660254037844387076, 1.000000000000000000, 0.8660254037844387076, 1.000000000000000000, 0.8660254037844387076, 1.000000000000000000, 0.8660254037844387076, 1.000000000000000000, 0.8660254037844387076, 1.000000000000000000, 0.8660254037844387076, 1.000000000000000000, 0.8660254037844387076, 1.000000000000000000, 0.8660254037844387076, 1.000000000000000000, 0.8660254037844387076, 1.000000000000000000, 0.8660254037844387076, 1.000000000000000000, 0.8660254037844387076, 1.000000000000000000, 0.8660254037844387076, 1.000000000000000000, 0.8660254037844387076, 1.000000000000000000, 0.8660254037844387076, 1.000000000000000000, 0.8660254037844387076, 1.000000000000000000, 0.8660254037844387076, 1.000000000000000000, 0.8660254037844387076, 1.000000000000000000, 0.8660254037844387076, 1.000000000000000000, 0.8660254037844387076, 1.000000000000000000, 0.8660254037844387076, 1.000000000000000000, 0.8660254037844387076, 1.000000000000000000, 0.8660254037844387076, 1.000000000000000000, 0.8660254037844387076, 1.000000000000000000, 0.8660254037844387076, 1.000000000000000000, 0.8660254037844387076, 1.000000000000000000, 0.8660254037844387076, 1.000000000000000000, 0.8660254037844387076, 1.000000000000000000, 0.8660254037844387076, 1.000000000000000000, 0.8660254037844387076, 1.000000000000000000, 0.8660254037844387076, 1.000000000000000000, 0.8660254037844387076, 1.000000000000000000, 0.8660254037844387076, 1.000000000000000000, 0.8660254037844387076, 1.000000000000000000, 0.8660254037844387076, 1.000000000000000000, 0.8660254037844387076, 1.000000000000000000, 0.8660254037844387076, 1.000000000000000000, 0.8660254037844387076, 1.000000000000000000, 0.8660254037844387076, 1.000000000000000000, 0.8660254037844387076, 1.000000000000000000, 0.8660254037844387076, 1.000000000000000000, 0.8660254037844387076, 1.000000000000000000, 0.8660254037844387076, 1.000000000000000000, 0.8660254037844387076, 1.000000000000000000, 0.8660254037844387076, 1.000000000000000000, 0.8660254037844387076, 1.000000000000000000, 0.8660254037844387076, 1.000000000000000000, 0.8660254037844387076, 1.000000000000000000, 0.8660254037844387076, 1.000000000000000000, 0.8660254037844387076, 1.000000000000000000, 0.8660254037844387076, 1.000000000000000000, 0.8660254037844387076, 1.000000000000000000, 0.8660254037844387076, 1.000000000000000000, 0.8660254037844387076, 1.000000000000000000, 0.8660254037844387076, 1.000000000000000000, 0.8660254037844387076, 1.000000000000000000, 0.8660254037844387076, 1.000000000000000000, 0.8660254037844387076, 1.000000000000000000, 0.8660254037844387076, 1.000000000000000000, 0.8660254037844387076, 1.000000000000000000, 0.8660254037844387076, 1.000000000000000000, 0.8660254037844387076, 1.000000000000000000, 0.8660254037844387076, 1.000000000000000000, 0.8660254037844387076, 1.000000000000000000, 0.8660254037844387076, 1.000000000000000000, 0.8660254037844387076, 1.000000000000000000, 0.8660254037844387076, 1.000000000000000000, 0.8660254037844387076, 1.000000000000000000, 0.8660254037844387076, 1.000000000000000000, 0.8660254037844387076, 1.000000000000000000, 0.8660254037844387076, 1.000000000000000000, 0.8660254037844387076, 1.000000000000000000, 0.8660254037844387076, 1.000000000000000000, 0.8660254037844387076, 1.000000000000000000, 0.8660254037844387076, 1.000000000000000000, 0.8660254037844387076, 1.000000000000000000, 0.8660254037844387076, 1.000000000000000000, 0.8660254037844387076, 1.000000000000000000, 0.8660254037844387076, 1.000000000000000000, 0.8660254037844387076, 1.000000000000000000, 0.8660254037844387076, 1.000000000000000000, 0.8660254037844387076, 1.000000000000000000, 0.8660254037844387076, 1.000000000000000000, 0.8660254037844387076, 1.000000000000000000, 0.8660254037844387076, 1.000000000000000000, 0.8660254037844387076, 1.000000000000000000, 0.8660254037844387076, 1.000000000000000000, 0.8660254037844387076, 1.000000000000000000, 0.8660254037844387076, 1.000000000000000000, 0.8660254037844387076, 1.000000000000000000, 0.8660254037844387076, 1.000000000000000000, 0.8660254037844387076, 1.000000000000000000, 0.8660254037844387076, 1.000000000000000000, 0.8660254037844387076, 1.000000000000000000, 0.8660254037844387076, 1.000000000000000000, 0.8660254037844387076, 1.000000000000000000, 0.8660254037844387076, 1.000000000000000000, 0.8660254037844387076, 1.000000000000000000, 0.8660254037844387076, 1.000000000000000000, 0.8660254037844387076, 1.000000000000000000, 0.8660254037844387076, 1.000000000000000000, 0.8660254037844387076, 1.000000000000000000, 0.8660254037844387076, 1.000000000000000000, 0.8660254037844387076, 1.000000000000000000, 0.8660254037844387076, 1.000000000000000000, 0.8660254037844387076, 1.000000000000000000, 0.8660254037844387076, 1.000000000000000000, 0.8660254037844387076, 1.000000000000000000, 0.8660254037844387076, 1.000000000000000000, 0.8660254037844387076, 1.000000000000000000, 0.8660254037844387076, 1.000000000000000000, 0.8660254037844387076, 1.000000000000000000, 0.8660254037844387076, 1.000000000000000000, 0.8660254037844387076, 1.000000000000000000, 0.8660254037844387076, 1.000000000000000000, 0.8660254037844387076, 1.000000000000000000, 0.8660254037844387076, 1.000000000000000000, 0.8660254037844387076, 1.000000000000000000, 0.9548848677736607726, 0.9401542295229587953 ) ) 
 REPRESENTATION_ITEM ( '' )  );
#14588=EDGE_CURVE ( 'NONE', #17802, #4869, #3956, .T. ) ;
#14598=CARTESIAN_POINT ( 'NONE',  ( 33.96355885174396860, 5.196152422706637353, 163.7530159683574311 ) ) ;
#14601=CYLINDRICAL_SURFACE ( 'NONE', #35176, 6.000000000000001776 ) ;
#14609=CARTESIAN_POINT ( 'NONE',  ( 23.87821517812500005, -4.985214923628404016, -1.340624999385475746 ) ) ;
#14622=CARTESIAN_POINT ( 'NONE',  ( 23.87821517812499650, 4.985214923628404904, -8.503124999385491378 ) ) ;
#14627=CARTESIAN_POINT ( 'NONE',  ( 34.34226204845910502, 5.407089921784862696, 166.6842891901658845 ) ) ;
#14640=AXIS2_PLACEMENT_3D ( 'NONE', #5278, #19340, #2062 ) ;
#14662=CARTESIAN_POINT ( 'NONE',  ( 18.12178482187500350, -4.985214923628407568, -1.978124999385488803 ) ) ;
#14665=ADVANCED_FACE ( 'NONE', ( #27715 ), #30936, .T. ) ;
#14669=CARTESIAN_POINT ( 'NONE',  ( 26.75643035624999655, 3.323476615752271268, -4.378124999385460292 ) ) ;
#14674=DIRECTION ( 'NONE',  ( 0.9961946980917462113, 0.000000000000000000, -0.08715574274765118534 ) ) ;
#14676=CARTESIAN_POINT ( 'NONE',  ( 36.79853094953357129, 7.347880794884117764E-16, 161.7357555859521199 ) ) ;
#14681=CARTESIAN_POINT ( 'NONE',  ( 26.75643035624999655, 3.323476615752271268, -4.940624999385510918 ) ) ;
#14685=ORIENTED_EDGE ( 'NONE', *, *, #7983, .T. ) ;
#14689=ADVANCED_FACE ( 'NONE', ( #4953, #1556 ), #33219, .F. ) ;
#14690=CARTESIAN_POINT ( 'NONE',  ( 20.99999999999999645, 0.000000000000000000, -8.000000000000000000 ) ) ;
#14691=CARTESIAN_POINT ( 'NONE',  ( 27.73678691053042300, 5.407089921784862696, 162.8202906008076241 ) ) ;
#14701=CARTESIAN_POINT ( 'NONE',  ( 24.98146486726017912, 0.000000000000000000, 164.3506311484184437 ) ) ;
#14704=ORIENTED_EDGE ( 'NONE', *, *, #15765, .F. ) ;
#14705=CARTESIAN_POINT ( 'NONE',  ( 15.00000000000000000, 0.000000000000000000, -5.849999999999994316 ) ) ;
#14707=CARTESIAN_POINT ( 'NONE',  ( 21.00000000000000355, 0.000000000000000000, 50.00000000000001421 ) ) ;
#14708=CARTESIAN_POINT ( 'NONE',  ( 27.92429219659289785, 5.196152422706630247, 163.5661617036773237 ) ) ;
#14710=CARTESIAN_POINT ( 'NONE',  ( 28.17311034766084887, 5.407089921784856479, 167.8074903081294167 ) ) ;
#14713=( BOUNDED_CURVE ( )  B_SPLINE_CURVE ( 2, ( #26388, #11801, #19978, #31520, #6107, #3270, #5921 ),
 .UNSPECIFIED., .F., .F. ) 
 B_SPLINE_CURVE_WITH_KNOTS ( ( 3, 2, 2, 3 ),
 ( 0.3478260869565210078, 0.3550724637681153539, 0.3623188405797096445, 0.3695652173913039351 ),
 .UNSPECIFIED. ) 
 CURVE ( )  GEOMETRIC_REPRESENTATION_ITEM ( )  RATIONAL_B_SPLINE_CURVE ( ( 1.000000000000013323, 0.8660254037844252739, 1.000000000000000000, 0.8660254037844387076, 1.000000000000000000, 0.8660254037844459241, 0.9999999999999927836 ) ) 
 REPRESENTATION_ITEM ( '' )  );
#14716=ORIENTED_EDGE ( 'NONE', *, *, #24095, .F. ) ;
#14718=FACE_OUTER_BOUND ( 'NONE', #21541, .T. ) ;
#14721=CARTESIAN_POINT ( 'NONE',  ( 23.87821517812500005, -4.985214923628404016, -5.840624999385479299 ) ) ;
#14724=CARTESIAN_POINT ( 'NONE',  ( 34.02892565880470954, -5.196152422706635576, 164.5001619919262055 ) ) ;
#14727=LINE ( 'NONE', #26276, #8302 ) ;
#14728=CARTESIAN_POINT ( 'NONE',  ( 34.36556471527461554, 5.196152422706631135, 168.3479640145299641 ) ) ;
#14730=ADVANCED_FACE ( 'NONE', ( #7443 ), #7258, .T. ) ;
#14741=CARTESIAN_POINT ( 'NONE',  ( 21.64885123950055501, 5.731983593561799317, -8.000000000000000000 ) ) ;
#14742=CARTESIAN_POINT ( 'NONE',  ( 31.35328515338631306, 7.209453229046482114, 168.3385908086170559 ) ) ;
#14743=CARTESIAN_POINT ( 'NONE',  ( 21.00000000000000000, 6.928203230275506996, -1.856249998770964860 ) ) ;
#14744=STYLED_ITEM ( 'NONE', ( #24481 ), #10611 ) ;
#14753=CARTESIAN_POINT ( 'NONE',  ( 25.02068495149662297, 0.000000000000000000, 164.7989187625597367 ) ) ;
#14755=ORIENTED_EDGE ( 'NONE', *, *, #25649, .F. ) ;
#14756=CARTESIAN_POINT ( 'NONE',  ( 30.65222614765987785, 7.209453229046475009, 160.3254497058415495 ) ) ;
#14757=CARTESIAN_POINT ( 'NONE',  ( 26.75643035624999655, 7.049594010296217766E-16, -7.115624999385477878 ) ) ;
#14759=CARTESIAN_POINT ( 'NONE',  ( 34.10694154304044901, 5.407089921784862696, 163.9945635053181547 ) ) ;
#14760=CARTESIAN_POINT ( 'NONE',  ( 28.04522078954815356, -5.196152422706638241, 164.9483818460552413 ) ) ;
#14767=ORIENTED_EDGE ( 'NONE', *, *, #31372, .F. ) ;
#14772=CARTESIAN_POINT ( 'NONE',  ( 26.75643035624999655, 3.323476615752271712, -5.390624999385475569 ) ) ;
#14799=CARTESIAN_POINT ( 'NONE',  ( 21.00000000000000000, -6.646953231504538984, -0.9281249993854503444 ) ) ;
#14802=CARTESIAN_POINT ( 'NONE',  ( 26.99999999999991118, -3.464101615137797463, -4.706249998770959841 ) ) ;
#14803=CARTESIAN_POINT ( 'NONE',  ( 25.24620043574905282, 0.000000000000000000, 167.3765725426477502 ) ) ;
#14811=CARTESIAN_POINT ( 'NONE',  ( 26.75643035624999655, 3.323476615752271712, -9.890624999385464022 ) ) ;
#14820=CARTESIAN_POINT ( 'NONE',  ( 34.30304196422265761, 5.407089921784862696, 166.2360015760246199 ) ) ;
#14826=CARTESIAN_POINT ( 'NONE',  ( 34.03873067997093216, -5.196152422706629359, 164.6122338966858933 ) ) ;
#14827=CARTESIAN_POINT ( 'NONE',  ( 25.19067013329413385, -3.604726614523240613, 169.5365065289374797 ) ) ;
#14828=ORIENTED_EDGE ( 'NONE', *, *, #16506, .F. ) ;
#14844=CARTESIAN_POINT ( 'NONE',  ( 25.45210587809749825, 0.000000000000000000, 169.7300825181138748 ) ) ;
#14853=CARTESIAN_POINT ( 'NONE',  ( 30.65222614765988141, 7.209453229046475009, 160.3254497058415495 ) ) ;
#14854=CARTESIAN_POINT ( 'NONE',  ( 26.75643035624999655, 3.323476615752271712, -1.790624999385476812 ) ) ;
#14859=ORIENTED_EDGE ( 'NONE', *, *, #36496, .F. ) ;
#14860=CARTESIAN_POINT ( 'NONE',  ( 26.75643035624999655, 3.323476615752271268, -3.928124999385464999 ) ) ;
#14867=CARTESIAN_POINT ( 'NONE',  ( 30.85077782416043135, -6.928203230275506996, 162.5949057530440029 ) ) ;
#14871=CARTESIAN_POINT ( 'NONE',  ( 20.99999999999999645, 6.646953231504538984, -5.765624999385476457 ) ) ;
#14881=CARTESIAN_POINT ( 'NONE',  ( 27.54068648934820729, 5.407089921784862696, 160.5788525301012157 ) ) ;
#14885=CARTESIAN_POINT ( 'NONE',  ( 26.99999999999999645, 7.347880794884117764E-16, -1.968749998770946696 ) ) ;
#14894=CARTESIAN_POINT ( 'NONE',  ( 18.00000000000000000, 5.196152422706630247, -6.824999999999997513 ) ) ;
#14898=CARTESIAN_POINT ( 'NONE',  ( 37.33287311370841621, 7.646167579472015790E-16, 165.0486662223039218 ) ) ;
#14903=ORIENTED_EDGE ( 'NONE', *, *, #12409, .F. ) ;
#14904=CYLINDRICAL_SURFACE ( 'NONE', #16706, 6.000000000000001776 ) ;
#14905=CARTESIAN_POINT ( 'NONE',  ( 18.12178482187500350, -4.985214923628407568, -5.915624999385471483 ) ) ;
#14913=CARTESIAN_POINT ( 'NONE',  ( 34.40478479951106294, 5.196152422706631135, 168.7962516286712571 ) ) ;
#14924=ORIENTED_EDGE ( 'NONE', *, *, #4375, .F. ) ;
#14927=ADVANCED_FACE ( 'NONE', ( #16908 ), #5886, .T. ) ;
#14928=CARTESIAN_POINT ( 'NONE',  ( 25.00000000000004263, 0.000000000000000000, 49.82535622836640954 ) ) ;
#14929=CARTESIAN_POINT ( 'NONE',  ( 31.17679477432231394, -7.209453229046482114, 166.3212965449812657 ) ) ;
#14930=CARTESIAN_POINT ( 'NONE',  ( 23.99999999999999645, 5.196152422706631135, -3.243749998770945275 ) ) ;
#14940=CARTESIAN_POINT ( 'NONE',  ( 36.86223210287109708, 7.646167579472015790E-16, 159.6692148526084907 ) ) ;
#14941=CARTESIAN_POINT ( 'NONE',  ( 15.00000000000000178, -3.464101615137757051, -0.4124999999999987566 ) ) ;
#14943=CARTESIAN_POINT ( 'NONE',  ( 37.28548217858939040, -3.604726614523238837, 164.5069853552165284 ) ) ;
#14944=CARTESIAN_POINT ( 'NONE',  ( 33.91126540609537443, -5.196152422706635576, 163.1552991495023548 ) ) ;
#14950=VERTEX_POINT ( 'NONE', #25794 ) ;
#14954=CARTESIAN_POINT ( 'NONE',  ( 33.93414378867374381, 5.196152422706631135, 163.4168002589758260 ) ) ;
#14958=CARTESIAN_POINT ( 'NONE',  ( 23.87821517812500005, -4.985214923628404016, -4.603124999385476812 ) ) ;
#14966=CARTESIAN_POINT ( 'NONE',  ( 20.99999999999999645, -6.928203230275506996, -3.037500000000010747 ) ) ;
#14977=FACE_OUTER_BOUND ( 'NONE', #28481, .T. ) ;
#14982=CARTESIAN_POINT ( 'NONE',  ( 31.12286715849720764, 7.209453229046475009, 165.7049010755369807 ) ) ;
#14983=DIRECTION ( 'NONE',  ( 1.000000000000000000, 0.000000000000000000, 0.000000000000000000 ) ) ;
#14994=CARTESIAN_POINT ( 'NONE',  ( 23.87821517812499650, 4.985214923628404904, -1.190624999385464511 ) ) ;
#14999=ORIENTED_EDGE ( 'NONE', *, *, #22340, .T. ) ;
#15001=CARTESIAN_POINT ( 'NONE',  ( 33.98928129033111389, 5.407089921784862696, 162.6497006628943041 ) ) ;
#15004=VECTOR ( 'NONE', #36234, 1000.000000000000000 ) ;
#15009=CARTESIAN_POINT ( 'NONE',  ( 37.40804494182826545, -3.604726614523235284, 165.9078841494080336 ) ) ;
#15010=EDGE_LOOP ( 'NONE', ( #36665, #103, #7453, #27382, #26530, #9981, #19537, #1412, #7684, #15844, #34846, #36276, #29753, #7312, #31878, #25900, #41, #4592, #31725, #32352, #3727, #348, #27010, #8520, #15191, #6060, #17511, #36617, #37083, #20214, #25245, #22986, #10839, #16828, #11405, #3475, #34657, #19796, #28783 ) ) ;
#15016=EDGE_CURVE ( 'NONE', #590, #33506, #19476, .T. ) ;
#15040=CARTESIAN_POINT ( 'NONE',  ( 24.44548853280170775, -3.604726614523240613, 161.0190418602530258 ) ) ;
#15041=CARTESIAN_POINT ( 'NONE',  ( 23.87821517812499650, 4.985214923628404904, -1.753124999385485827 ) ) ;
#15044=ORIENTED_EDGE ( 'NONE', *, *, #2979, .F. ) ;
#15046=CARTESIAN_POINT ( 'NONE',  ( 26.75643035624999655, -3.323476615752267271, -4.453124999385455141 ) ) ;
#15054=CARTESIAN_POINT ( 'NONE',  ( 36.68413903717728175, 3.464101615137755275, 160.4282500447066866 ) ) ;
#15057=EDGE_CURVE ( 'NONE', #15757, #8199, #3043, .T. ) ;
#15059=CARTESIAN_POINT ( 'NONE',  ( 20.99999999999999645, 6.646953231504538984, -7.565624999385492266 ) ) ;
#15060=CARTESIAN_POINT ( 'NONE',  ( 24.98477879236699195, 0.000000000000000000, 49.65137702900941008 ) ) ;
#15063=CARTESIAN_POINT ( 'NONE',  ( 14.99999999999972466, -3.464101615137598067, -0.8062499987709568217 ) ) ;
#15067=CARTESIAN_POINT ( 'NONE',  ( 24.39809759768267128, 0.000000000000000000, 160.4773609931656608 ) ) ;
#15079=CARTESIAN_POINT ( 'NONE',  ( 15.00000000000000000, 3.464101615137752166, -8.137499999999985079 ) ) ;
#15080=CARTESIAN_POINT ( 'NONE',  ( 26.99999999999999645, 7.347880794884117764E-16, -4.275000000000001243 ) ) ;
#15083=CARTESIAN_POINT ( 'NONE',  ( 37.48648511030114605, -3.604726614523235284, 166.8044593776906197 ) ) ;
#15085=CARTESIAN_POINT ( 'NONE',  ( 30.63506736085999904, 6.928203230275506996, 160.1293238752668913 ) ) ;
#15089=CARTESIAN_POINT ( 'NONE',  ( 36.94560626531313829, 7.347880794884125653E-16, 163.4168341377576041 ) ) ;
#15091=CARTESIAN_POINT ( 'NONE',  ( 24.59253236524820352, -3.464101615137419543, 159.9051123081840444 ) ) ;
#15092=( BOUNDED_CURVE ( )  B_SPLINE_CURVE ( 2, ( #13209, #10171, #10358, #4479, #1638, #19288, #30827 ),
 .UNSPECIFIED., .F., .F. ) 
 B_SPLINE_CURVE_WITH_KNOTS ( ( 3, 2, 2, 3 ),
 ( 0.1956521739130429038, 0.2028985507246371944, 0.2101449275362314850, 0.2173913043478257756 ),
 .UNSPECIFIED. ) 
 CURVE ( )  GEOMETRIC_REPRESENTATION_ITEM ( )  RATIONAL_B_SPLINE_CURVE ( ( 1.000000000000010658, 0.8660254037844279384, 1.000000000000000000, 0.8660254037844387076, 1.000000000000000000, 0.8660254037844443697, 0.9999999999999943379 ) ) 
 REPRESENTATION_ITEM ( '' )  );
#15093=CARTESIAN_POINT ( 'NONE',  ( 30.76253263452132813, -6.928203230275514990, 161.5862586200017574 ) ) ;
#15094=CARTESIAN_POINT ( 'NONE',  ( 15.24356964375000167, -3.323476615752272600, -7.303124999385448568 ) ) ;
#15097=CARTESIAN_POINT ( 'NONE',  ( 26.99999999999962341, -3.464101615137965773, -5.156249998770960019 ) ) ;
#15101=CARTESIAN_POINT ( 'NONE',  ( 36.86059793269458140, 3.604726614523243278, 159.6505362020193104 ) ) ;
#15110=ORIENTED_EDGE ( 'NONE', *, *, #9600, .F. ) ;
#15114=CARTESIAN_POINT ( 'NONE',  ( 31.27484498491342180, 7.209453229046482114, 167.4420155803344699 ) ) ;
#15125=CARTESIAN_POINT ( 'NONE',  ( 30.67183618977810156, -7.209453229046475009, 160.5495935129122245 ) ) ;
#15126=CARTESIAN_POINT ( 'NONE',  ( 26.99999999999999645, 7.347880794884117764E-16, -0.2250000000000029754 ) ) ;
#15129=CARTESIAN_POINT ( 'NONE',  ( 34.09386818162830224, -5.407089921784861808, 163.8451343006043999 ) ) ;
#15130=CARTESIAN_POINT ( 'NONE',  ( 33.87204532185894124, -5.196152422706635576, 162.7070115353610618 ) ) ;
#15139=( BOUNDED_CURVE ( )  B_SPLINE_CURVE ( 2, ( #22042, #27899, #1929, #18033, #11769, #37345, #2855 ),
 .UNSPECIFIED., .F., .F. ) 
 B_SPLINE_CURVE_WITH_KNOTS ( ( 3, 2, 2, 3 ),
 ( 0.3260869565217382471, 0.3333333333333325932, 0.3405797101449269948, 0.3478260869565213409 ),
 .UNSPECIFIED. ) 
 CURVE ( )  GEOMETRIC_REPRESENTATION_ITEM ( )  RATIONAL_B_SPLINE_CURVE ( ( 1.000000000000016431, 0.8660254037844222763, 1.000000000000000000, 0.8660254037844387076, 1.000000000000000000, 0.8660254037844459241, 0.9999999999999927836 ) ) 
 REPRESENTATION_ITEM ( '' )  );
#15141=CARTESIAN_POINT ( 'NONE',  ( 15.24356964374999990, 3.323476615752268604, -4.790624999385491023 ) ) ;
#15145=CARTESIAN_POINT ( 'NONE',  ( 26.99999999999999645, 7.347880794884117764E-16, -6.468749998770951137 ) ) ;
#15158=CARTESIAN_POINT ( 'NONE',  ( 34.19028422204287665, 5.407089921784857367, 164.9471746853683669 ) ) ;
#15172=CARTESIAN_POINT ( 'NONE',  ( 28.05545009495152087, 5.407089921784856479, 166.4626274657055660 ) ) ;
#15173=CARTESIAN_POINT ( 'NONE',  ( 26.75643035624999655, 3.323476615752271712, -3.478124999385468819 ) ) ;
#15177=CARTESIAN_POINT ( 'NONE',  ( 37.06326651802246630, 7.347880794884125653E-16, 164.7616969801814548 ) ) ;
#15182=VERTEX_POINT ( 'NONE', #30145 ) ;
#15185=CARTESIAN_POINT ( 'NONE',  ( 18.12178482187499640, 4.985214923628404904, -1.565624999385478722 ) ) ;
#15187=CARTESIAN_POINT ( 'NONE',  ( 26.99999999999999645, 3.464101615137755275, -7.781249998770935150 ) ) ;
#15191=ORIENTED_EDGE ( 'NONE', *, *, #2236, .T. ) ;
#15194=CARTESIAN_POINT ( 'NONE',  ( 34.17230835010118994, -5.407089921784861808, 164.7417095288869859 ) ) ;
#15202=CARTESIAN_POINT ( 'NONE',  ( 37.49302179100721588, 3.604726614523238837, 166.8791739800475113 ) ) ;
#15220=CARTESIAN_POINT ( 'NONE',  ( 25.18576762276457259, -3.604726614523244610, 169.4804705771697968 ) ) ;
#15221=CARTESIAN_POINT ( 'NONE',  ( 24.85073125303116726, 3.464101615137512358, 162.8563391000565161 ) ) ;
#15222=ADVANCED_FACE ( 'NONE', ( #7035 ), #21067, .T. ) ;
#15229=CARTESIAN_POINT ( 'NONE',  ( 33.79808337967844523, 5.407089921784857367, 160.4642985439555218 ) ) ;
#15230=CARTESIAN_POINT ( 'NONE',  ( 15.24356964374999990, 0.000000000000000000, -5.653124999385472194 ) ) ;
#15235=CARTESIAN_POINT ( 'NONE',  ( 20.99999999999999645, 6.646953231504538984, -5.653124999385485516 ) ) ;
#15239=EDGE_CURVE ( 'NONE', #22746, #9403, #29760, .T. ) ;
#15247=CARTESIAN_POINT ( 'NONE',  ( 18.12178482187499640, 4.985214923628404904, -7.978124999385494576 ) ) ;
#15255=CARTESIAN_POINT ( 'NONE',  ( 27.59297993499679791, -5.407089921784865361, 161.1765693489562352 ) ) ;
#15259=CARTESIAN_POINT ( 'NONE',  ( 26.99999999999999645, 7.347880794884117764E-16, -1.068749998770962550 ) ) ;
#15266=ORIENTED_EDGE ( 'NONE', *, *, #36966, .F. ) ;
#15267=CARTESIAN_POINT ( 'NONE',  ( 21.00000000000000000, 6.928203230275506996, -7.312499999999986677 ) ) ;
#15272=CARTESIAN_POINT ( 'NONE',  ( 28.06852345636367119, -5.407089921784859143, 166.6120566704193493 ) ) ;
#15281=CARTESIAN_POINT ( 'NONE',  ( 25.22662187717753568, 0.000000000000000000, 169.9474368419002985 ) ) ;
#15282=CARTESIAN_POINT ( 'NONE',  ( 21.00000000000000000, 6.646953231504538984, -5.653124999385485516 ) ) ;
#15291=CARTESIAN_POINT ( 'NONE',  ( 37.34434378849074676, -3.464101615137751278, 167.9744248827517197 ) ) ;
#15296=CARTESIAN_POINT ( 'NONE',  ( 23.87821517812500005, -4.985214923628404016, -0.5531249993854792102 ) ) ;
#15305=CARTESIAN_POINT ( 'NONE',  ( 31.31406506914986920, 7.209453229046482114, 167.8903031944757629 ) ) ;
#15317=CARTESIAN_POINT ( 'NONE',  ( 15.00000000000000000, 0.000000000000000000, -0.4500000000000059508 ) ) ;
#15320=CARTESIAN_POINT ( 'NONE',  ( 28.06362094583411704, -5.407089921784865361, 166.5560207186516664 ) ) ;
#15321=UNCERTAINTY_MEASURE_WITH_UNIT (LENGTH_MEASURE( 1.000000000000000082E-05 ), #32625, 'distance_accuracy_value', 'NONE');
#15322=CARTESIAN_POINT ( 'NONE',  ( 36.98809468990261706, 3.464101615137759271, 163.9024790530773146 ) ) ;
#15328=VERTEX_POINT ( 'NONE', #35068 ) ;
#15333=CARTESIAN_POINT ( 'NONE',  ( 26.75643035624999655, 7.049594010296217766E-16, -4.078124999385480010 ) ) ;
#15343=CARTESIAN_POINT ( 'NONE',  ( 28.21190614766015159, -5.196152422706632912, 166.8536042073800729 ) ) ;
#15347=CARTESIAN_POINT ( 'NONE',  ( 18.00000000000000000, 5.196152422706630247, -7.218749998770951137 ) ) ;
#15348=CARTESIAN_POINT ( 'NONE',  ( 24.79520095057666396, 0.000000000000000000, 165.0162730863461604 ) ) ;
#15354=EDGE_CURVE ( 'NONE', #35216, #1170, #20679, .T. ) ;
#15361=CARTESIAN_POINT ( 'NONE',  ( 34.38638464322509947, 5.407089921784857367, 167.1886127560748321 ) ) ;
#15362=CARTESIAN_POINT ( 'NONE',  ( 15.24356964375000167, -3.323476615752272600, -1.903124999385467753 ) ) ;
#15376=CARTESIAN_POINT ( 'NONE',  ( 26.75643035624999655, 7.049594010296217766E-16, -2.165624999385467930 ) ) ;
#15378=CARTESIAN_POINT ( 'NONE',  ( 21.00000000000000000, -6.928203230275506996, -6.581249998770967835 ) ) ;
#15384=CARTESIAN_POINT ( 'NONE',  ( 27.86752052465190133, -5.407089921784865361, 164.3145826479452296 ) ) ;
#15386=( BOUNDED_CURVE ( )  B_SPLINE_CURVE ( 2, ( #14333, #17183, #20584, #14516, #25887, #31943, #6356 ),
 .UNSPECIFIED., .F., .F. ) 
 B_SPLINE_CURVE_WITH_KNOTS ( ( 3, 2, 2, 3 ),
 ( 0.3043478260869552088, 0.3115942028985494994, 0.3188405797101437900, 0.3260869565217381361 ),
 .UNSPECIFIED. ) 
 CURVE ( )  GEOMETRIC_REPRESENTATION_ITEM ( )  RATIONAL_B_SPLINE_CURVE ( ( 1.000000000000024647, 0.8660254037844140607, 1.000000000000000000, 0.8660254037844387076, 1.000000000000000000, 0.8660254037844571373, 0.9999999999999815703 ) ) 
 REPRESENTATION_ITEM ( '' )  );
#15393=CARTESIAN_POINT ( 'NONE',  ( 34.25565102910361759, -5.407089921784855591, 165.6943207089371981 ) ) ;
#15404=ADVANCED_FACE ( 'NONE', ( #21981 ), #27201, .T. ) ;
#15414=CARTESIAN_POINT ( 'NONE',  ( 15.81644453130096828, -3.010575440655008261, -7.999999999999994671 ) ) ;
#15415=DIRECTION ( 'NONE',  ( 0.9961946980917462113, 0.000000000000000000, -0.08715574274765118534 ) ) ;
#15418=ORIENTED_EDGE ( 'NONE', *, *, #26483, .F. ) ;
#15423=CARTESIAN_POINT ( 'NONE',  ( 23.87821517812499650, 4.985214923628404904, -4.453124999385494220 ) ) ;
#15426=VERTEX_POINT ( 'NONE', #17948 ) ;
#15427=CARTESIAN_POINT ( 'NONE',  ( 28.01580572647793943, -5.196152422706632912, 164.6121661366736078 ) ) ;
#15438=CARTESIAN_POINT ( 'NONE',  ( 20.99999999999999645, -6.646953231504538984, -6.890624999385480898 ) ) ;
#15442=CARTESIAN_POINT ( 'NONE',  ( 36.83448269341756998, -3.464101615137414214, 162.1466858989149102 ) ) ;
#15451=CARTESIAN_POINT ( 'NONE',  ( 15.00000000000000355, 7.347880794884112834E-16, -8.000000000000000000 ) ) ;
#15459=CARTESIAN_POINT ( 'NONE',  ( 15.00000000000000000, 3.464101615137752166, -7.237499999999992717 ) ) ;
#15460=CARTESIAN_POINT ( 'NONE',  ( 15.00000000000000000, 0.000000000000000000, -4.500000000000003553 ) ) ;
#15463=CARTESIAN_POINT ( 'NONE',  ( 24.87364111904954811, 0.000000000000000000, 165.9128483146287465 ) ) ;
#15467=ORIENTED_EDGE ( 'NONE', *, *, #34443, .T. ) ;
#15469=CARTESIAN_POINT ( 'NONE',  ( 29.51984228635672380, 5.908847293266075162, 159.3365288790247121 ) ) ;
#15470=CARTESIAN_POINT ( 'NONE',  ( 20.99999999999999645, -6.928203230275506996, -2.587499999999983480 ) ) ;
#15473=CARTESIAN_POINT ( 'NONE',  ( 15.24356964374999990, 3.323476615752268604, -8.278124999385466865 ) ) ;
#15480=CARTESIAN_POINT ( 'NONE',  ( 28.17268606342371129, -5.196152422706632912, 166.4053165932387515 ) ) ;
#15492=CARTESIAN_POINT ( 'NONE',  ( 26.99999999999967670, 3.464101615137938683, -7.837500000000005684 ) ) ;
#15494=CARTESIAN_POINT ( 'NONE',  ( 28.18128119854344860, -5.407089921784865361, 167.9008835610755455 ) ) ;
#15497=EDGE_CURVE ( 'NONE', #20530, #13274, #9050, .T. ) ;
#15505=DIRECTION ( 'NONE',  ( 0.9961946980917462113, 0.000000000000000000, -0.08715574274765178209 ) ) ;
#15510=CARTESIAN_POINT ( 'NONE',  ( 23.87821517812500005, -4.985214923628404016, -9.440624999385471838 ) ) ;
#15512=CARTESIAN_POINT ( 'NONE',  ( 37.24626209435294300, -3.604726614523238837, 164.0586977410752638 ) ) ;
#15513=CARTESIAN_POINT ( 'NONE',  ( 33.88511868327108090, 5.196152422706637353, 162.8564407400748451 ) ) ;
#15516=AXIS2_PLACEMENT_3D ( 'NONE', #22959, #5501, #5878 ) ;
#15521=ORIENTED_EDGE ( 'NONE', *, *, #33476, .F. ) ;
#15525=CARTESIAN_POINT ( 'NONE',  ( 15.24356964374999990, 3.323476615752268604, -5.690624999385482496 ) ) ;
#15532=DIRECTION ( 'NONE',  ( 0.08715574274765150453, 0.000000000000000000, 0.9961946980917461003 ) ) ;
#15534=CARTESIAN_POINT ( 'NONE',  ( 37.18746345154525557, -3.464101615137590073, 166.1812744261865191 ) ) ;
#15538=CARTESIAN_POINT ( 'NONE',  ( 30.98559686366965238, -7.209453229046475009, 164.1358944260424835 ) ) ;
#15549=CARTESIAN_POINT ( 'NONE',  ( 25.07300988058479874, -3.604726614523240613, 168.1916436865135722 ) ) ;
#15550=CARTESIAN_POINT ( 'NONE',  ( 21.00000000000000000, -6.646953231504538984, -2.278124999385469529 ) ) ;
#15552=CYLINDRICAL_SURFACE ( 'NONE', #13225, 5.999999999999994671 ) ;
#15553=CARTESIAN_POINT ( 'NONE',  ( 24.34069010239548447, -4.874609697617195536, -8.000000000000003553 ) ) ;
#15556=DIRECTION ( 'NONE',  ( 0.9961946980917462113, 0.000000000000000000, -0.08715574274765118534 ) ) ;
#15563=CARTESIAN_POINT ( 'NONE',  ( 23.87821517812500005, -4.985214923628404016, -2.690624999385465621 ) ) ;
#15565=CARTESIAN_POINT ( 'NONE',  ( 15.00000000000000000, 3.464101615137752166, -10.33124999877095362 ) ) ;
#15567=ORIENTED_EDGE ( 'NONE', *, *, #751, .T. ) ;
#15572=CARTESIAN_POINT ( 'NONE',  ( 24.71185827157421855, 0.000000000000000000, 164.0636619062959483 ) ) ;
#15580=CARTESIAN_POINT ( 'NONE',  ( 37.48975345065418452, 7.646167579472015790E-16, 166.8418166788690655 ) ) ;
#15590=VERTEX_POINT ( 'NONE', #14537 ) ;
#15598=CARTESIAN_POINT ( 'NONE',  ( 36.98482634954957859, 7.347880794884125653E-16, 163.8651217518988688 ) ) ;
#15599=CARTESIAN_POINT ( 'NONE',  ( 15.20137627347641285, 1.191849618220900631, -7.999999999999998224 ) ) ;
#15600=CYLINDRICAL_SURFACE ( 'NONE', #23628, 5.999999999999994671 ) ;
#15602=VERTEX_POINT ( 'NONE', #492 ) ;
#15607=CARTESIAN_POINT ( 'NONE',  ( 26.75643035624999655, -3.323476615752267715, -3.665624999385485694 ) ) ;
#15609=( BOUNDED_CURVE ( )  B_SPLINE_CURVE ( 2, ( #17537, #2928, #16976, #28519, #11645, #20567, #23403 ),
 .UNSPECIFIED., .F., .F. ) 
 B_SPLINE_CURVE_WITH_KNOTS ( ( 3, 2, 2, 3 ),
 ( 0.04347826086956579211, 0.05072463768116009658, 0.05797101449275439411, 0.06521739130434869858 ),
 .UNSPECIFIED. ) 
 CURVE ( )  GEOMETRIC_REPRESENTATION_ITEM ( )  RATIONAL_B_SPLINE_CURVE ( ( 0.9999999999999893419, 0.8660254037844493658, 1.000000000000000000, 0.8660254037844387076, 1.000000000000000000, 0.8660254037844226094, 1.000000000000016209 ) ) 
 REPRESENTATION_ITEM ( '' )  );
#15611=CARTESIAN_POINT ( 'NONE',  ( 15.24356964374999990, 0.000000000000000000, -7.340624999385481075 ) ) ;
#15614=EDGE_CURVE ( 'NONE', #25852, #34104, #5387, .T. ) ;
#15618=CARTESIAN_POINT ( 'NONE',  ( 33.64652983760650073, -5.196152422706629359, 160.1293577552730483 ) ) ;
#15623=CARTESIAN_POINT ( 'NONE',  ( 26.75643035624999655, 3.323476615752271268, -6.740624999385493865 ) ) ;
#15624=DIRECTION ( 'NONE',  ( 0.000000000000000000, 0.000000000000000000, 1.000000000000000000 ) ) ;
#15639=CARTESIAN_POINT ( 'NONE',  ( 24.66770419336863185, 0.000000000000000000, 160.7643302352881278 ) ) ;
#15641=CARTESIAN_POINT ( 'NONE',  ( 24.99999999999998934, 2.343145750507540814, 49.65004534589634488 ) ) ;
#15647=CARTESIAN_POINT ( 'NONE',  ( 26.99999999999999645, 3.464101615137755275, -6.487500000000020250 ) ) ;
#15652=CARTESIAN_POINT ( 'NONE',  ( 31.10325711637897328, -7.209453229046475009, 165.4807572684663342 ) ) ;
#15663=CARTESIAN_POINT ( 'NONE',  ( 15.24356964374999990, 3.323476615752268604, -9.628124999385486049 ) ) ;
#15669=DIRECTION ( 'NONE',  ( 0.9961946980917462113, 0.000000000000000000, -0.08715574274765178209 ) ) ;
#15670=CARTESIAN_POINT ( 'NONE',  ( 28.29034631613303929, -5.196152422706632912, 167.7501794356626306 ) ) ;
#15672=ADVANCED_FACE ( 'NONE', ( #6564 ), #35360, .T. ) ;
#15675=EDGE_CURVE ( 'NONE', #2680, #37220, #19414, .T. ) ;
#15681=ORIENTED_EDGE ( 'NONE', *, *, #36955, .F. ) ;
#15684=CARTESIAN_POINT ( 'NONE',  ( 37.30839204460733782, 7.347880794884117764E-16, 167.5634945697888440 ) ) ;
#15685=CARTESIAN_POINT ( 'NONE',  ( 37.36719068741531657, 7.646167579472024665E-16, 165.4409178846775603 ) ) ;
#15691=DIRECTION ( 'NONE',  ( 0.08715574274765150453, 0.000000000000000000, 0.9961946980917461003 ) ) ;
#15693=CARTESIAN_POINT ( 'NONE',  ( 36.71028575989448228, 7.347880794884125653E-16, 160.7271084529098744 ) ) ;
#15699=LINE ( 'NONE', #27250, #33605 ) ;
#15700=ORIENTED_EDGE ( 'NONE', *, *, #2267, .T. ) ;
#15701=CARTESIAN_POINT ( 'NONE',  ( 21.00000000000000000, -6.928203230275506996, -0.7875000000000005329 ) ) ;
#15703=CARTESIAN_POINT ( 'NONE',  ( 33.95006120609467359, 5.407089921784862696, 162.2014130487530110 ) ) ;
#15704=CARTESIAN_POINT ( 'NONE',  ( 33.75438506914960612, -5.196152422706635576, 161.3621486929372111 ) ) ;
#15714=CARTESIAN_POINT ( 'NONE',  ( 21.00000000000000000, 6.646953231504538984, -6.665624999385467930 ) ) ;
#15727=CARTESIAN_POINT ( 'NONE',  ( 37.21521286099908110, 7.646167579472015790E-16, 163.7038033798800711 ) ) ;
#15731=FACE_OUTER_BOUND ( 'NONE', #32238, .T. ) ;
#15737=ORIENTED_EDGE ( 'NONE', *, *, #11097, .F. ) ;
#15738=CARTESIAN_POINT ( 'NONE',  ( 28.02930337212723089, -5.407089921784859143, 166.1637690562780278 ) ) ;
#15739=CARTESIAN_POINT ( 'NONE',  ( 23.87821517812500005, -4.985214923628404016, -3.590624999385477523 ) ) ;
#15741=CARTESIAN_POINT ( 'NONE',  ( 24.90318630322867932, -4.417295604025225586, -7.999999999999998224 ) ) ;
#15742=CARTESIAN_POINT ( 'NONE',  ( 34.34268633269625326, -5.196152422706635576, 168.0864629050564929 ) ) ;
#15753=CARTESIAN_POINT ( 'NONE',  ( 21.00000000000000000, -6.646953231504538984, -0.9281249993854503444 ) ) ;
#15756=CARTESIAN_POINT ( 'NONE',  ( 21.00000000000000000, -6.928203230275506996, -8.831249998770948295 ) ) ;
#15757=VERTEX_POINT ( 'NONE', #15853 ) ;
#15759=EDGE_CURVE ( 'NONE', #24412, #35079, #3715, .T. ) ;
#15760=VERTEX_POINT ( 'NONE', #21173 ) ;
#15764=CARTESIAN_POINT ( 'NONE',  ( 34.09386818162830224, -5.407089921784861808, 163.8451343006043999 ) ) ;
#15765=EDGE_CURVE ( 'NONE', #12608, #31196, #1072, .T. ) ;
#15772=CARTESIAN_POINT ( 'NONE',  ( 28.01623001071507701, 5.407089921784856479, 166.0143398515642730 ) ) ;
#15789=CARTESIAN_POINT ( 'NONE',  ( 15.00000000000000000, 0.000000000000000000, -5.849999999999994316 ) ) ;
#15792=CARTESIAN_POINT ( 'NONE',  ( 30.74292259240310443, 6.928203230275514990, 161.3621148129311109 ) ) ;
#15799=CARTESIAN_POINT ( 'NONE',  ( 15.24356964374999990, 3.323476615752268604, -5.240624999385486760 ) ) ;
#15811=( BOUNDED_CURVE ( )  B_SPLINE_CURVE ( 2, ( #23372, #34922, #8966, #6110, #17692, #31522, #29231 ),
 .UNSPECIFIED., .F., .F. ) 
 B_SPLINE_CURVE_WITH_KNOTS ( ( 3, 2, 2, 3 ),
 ( 0.1086956521739126380, 0.1159420289855069286, 0.1231884057971012053, 0.1304347826086954820 ),
 .UNSPECIFIED. ) 
 CURVE ( )  GEOMETRIC_REPRESENTATION_ITEM ( )  RATIONAL_B_SPLINE_CURVE ( ( 1.000000000000007327, 0.8660254037844312691, 1.000000000000000000, 0.8660254037844387076, 1.000000000000000000, 0.8660254037844418162, 0.9999999999999968914 ) ) 
 REPRESENTATION_ITEM ( '' )  );
#15816=FACE_OUTER_BOUND ( 'NONE', #33, .T. ) ;
#15820=CARTESIAN_POINT ( 'NONE',  ( 20.99999999999999645, 0.000000000000000000, -8.000000000000000000 ) ) ;
#15830=( BOUNDED_CURVE ( )  B_SPLINE_CURVE ( 2, ( #30055, #18516, #19267, #4829, #4089, #21355, #22098 ),
 .UNSPECIFIED., .F., .F. ) 
 B_SPLINE_CURVE_WITH_KNOTS ( ( 3, 2, 2, 3 ),
 ( 0.1086956521739118053, 0.1159420289855061098, 0.1231884057971004143, 0.1304347826086947049 ),
 .UNSPECIFIED. ) 
 CURVE ( )  GEOMETRIC_REPRESENTATION_ITEM ( )  RATIONAL_B_SPLINE_CURVE ( ( 1.000000000000022871, 0.8660254037844159480, 1.000000000000000000, 0.8660254037844387076, 1.000000000000000000, 0.8660254037844561381, 0.9999999999999825695 ) ) 
 REPRESENTATION_ITEM ( '' )  );
#15834=EDGE_LOOP ( 'NONE', ( #22330, #32816, #20344, #22835 ) ) ;
#15838=CARTESIAN_POINT ( 'NONE',  ( 24.83115269446006934, 3.604726614523236616, 165.4272033993090076 ) ) ;
#15844=ORIENTED_EDGE ( 'NONE', *, *, #5730, .T. ) ;
#15848=DIRECTION ( 'NONE',  ( 0.08715574274765150453, 0.000000000000000000, 0.9961946980917461003 ) ) ;
#15849=CARTESIAN_POINT ( 'NONE',  ( 26.75643035624999655, -3.323476615752267715, -9.853124999385466154 ) ) ;
#15853=CARTESIAN_POINT ( 'NONE',  ( 25.22171936664797798, 0.000000000000000000, 169.8914008901326724 ) ) ;
#15859=CARTESIAN_POINT ( 'NONE',  ( 31.28219875076131018, -6.928203230275506996, 167.5260695085981411 ) ) ;
#15873=CARTESIAN_POINT ( 'NONE',  ( 37.17435860658612512, 3.604726614523243278, 163.2368371151495694 ) ) ;
#15885=CARTESIAN_POINT ( 'NONE',  ( 15.00000000000000000, 0.000000000000000000, -4.443749998770951670 ) ) ;
#15889=ORIENTED_EDGE ( 'NONE', *, *, #25804, .T. ) ;
#15890=CARTESIAN_POINT ( 'NONE',  ( 26.99999999999999645, 7.347880794884117764E-16, -2.024999999999999023 ) ) ;
#15892=CARTESIAN_POINT ( 'NONE',  ( 30.80420397407610622, 7.209453229046482114, 162.0625642106390956 ) ) ;
#15893=CARTESIAN_POINT ( 'NONE',  ( 36.67433401601106624, 3.464101615137759271, 160.3161781399470271 ) ) ;
#15895=CARTESIAN_POINT ( 'NONE',  ( 36.71028575989448228, 7.347880794884125653E-16, 160.7271084529098744 ) ) ;
#15901=CARTESIAN_POINT ( 'NONE',  ( 21.00000000000000355, 0.000000000000000000, 50.00000000000001421 ) ) ;
#15904=CARTESIAN_POINT ( 'NONE',  ( 18.12178482187500350, -4.985214923628407568, -6.028124999385486404 ) ) ;
#15918=CARTESIAN_POINT ( 'NONE',  ( 27.78090950529641745, 5.407089921784856479, 163.3246141667165716 ) ) ;
#15921=CARTESIAN_POINT ( 'NONE',  ( 15.00000000000034461, -3.464101615137956003, -3.956249998770951404 ) ) ;
#15922=LINE ( 'NONE', #33903, #7871 ) ;
#15929=CARTESIAN_POINT ( 'NONE',  ( 24.71349244175073778, 3.604726614523236616, 164.0823405568851570 ) ) ;
#15930=CARTESIAN_POINT ( 'NONE',  ( 18.12178482187499640, 4.985214923628404904, -2.015624999385456917 ) ) ;
#15933=CARTESIAN_POINT ( 'NONE',  ( 25.47825260081467036, 3.464101615137757051, 170.0289409263170626 ) ) ;
#15934=LINE ( 'NONE', #10233, #36805 ) ;
#15944=CARTESIAN_POINT ( 'NONE',  ( 23.87821517812500005, -4.985214923628404016, -3.590624999385477523 ) ) ;
#15946=CARTESIAN_POINT ( 'NONE',  ( 18.00000000000000000, 5.196152422706630247, -9.018749998770946519 ) ) ;
#15947=ORIENTED_EDGE ( 'NONE', *, *, #10404, .T. ) ;
#15953=CARTESIAN_POINT ( 'NONE',  ( 27.59297993499679791, -5.407089921784865361, 161.1765693489562352 ) ) ;
#15962=DIRECTION ( 'NONE',  ( 0.9961946980917462113, 0.000000000000000000, -0.08715574274765118534 ) ) ;
#15966=ADVANCED_FACE ( 'NONE', ( #19032 ), #2506, .F. ) ;
#15974=FACE_OUTER_BOUND ( 'NONE', #30433, .T. ) ;
#15980=CARTESIAN_POINT ( 'NONE',  ( 21.00000000000000355, 0.000000000000000000, 50.00000000000001421 ) ) ;
#15990=CARTESIAN_POINT ( 'NONE',  ( 21.00000000000000000, -6.646953231504538984, -4.640624999385471128 ) ) ;
#15994=CARTESIAN_POINT ( 'NONE',  ( 20.99999999999999645, 6.646953231504538984, -6.553124999385445903 ) ) ;
#16009=CARTESIAN_POINT ( 'NONE',  ( 26.97716818855048260, 0.000000000000000000, 49.47706554351410801 ) ) ;
#16012=LINE ( 'NONE', #12975, #5949 ) ;
#16014=ORIENTED_EDGE ( 'NONE', *, *, #36792, .F. ) ;
#16025=FACE_OUTER_BOUND ( 'NONE', #32112, .T. ) ;
#16026=FACE_OUTER_BOUND ( 'NONE', #22641, .T. ) ;
#16029=CARTESIAN_POINT ( 'NONE',  ( 27.99008328789078703, -5.407089921784859143, 165.7154814421367348 ) ) ;
#16030=CARTESIAN_POINT ( 'NONE',  ( 23.99999999999999645, 5.196152422706631135, -1.950000000000007283 ) ) ;
#16032=ORIENTED_EDGE ( 'NONE', *, *, #20856, .F. ) ;
#16037=CARTESIAN_POINT ( 'NONE',  ( 26.75643035624999655, -3.323476615752267271, -0.8531249993854884694 ) ) ;
#16040=CARTESIAN_POINT ( 'NONE',  ( 18.12178482187500350, -4.985214923628407568, -8.615624999385479654 ) ) ;
#16043=( BOUNDED_CURVE ( )  B_SPLINE_CURVE ( 2, ( #23811, #14394, #25951, #15470, #14212, #27024, #2823 ),
 .UNSPECIFIED., .F., .F. ) 
 B_SPLINE_CURVE_WITH_KNOTS ( ( 3, 2, 2, 3 ),
 ( 0.2391304347826092025, 0.2463768115942035208, 0.2536231884057978392, 0.2608695652173921298 ),
 .UNSPECIFIED. ) 
 CURVE ( )  GEOMETRIC_REPRESENTATION_ITEM ( )  RATIONAL_B_SPLINE_CURVE ( ( 0.9999999999999907851, 0.8660254037844479225, 1.000000000000000000, 0.8660254037844387076, 1.000000000000000000, 0.8660254037844232755, 1.000000000000015321 ) ) 
 REPRESENTATION_ITEM ( '' )  );
#16047=CARTESIAN_POINT ( 'NONE',  ( 0.000000000000000000, 0.000000000000000000, 0.000000000000000000 ) ) ;
#16048=CARTESIAN_POINT ( 'NONE',  ( 37.15151170766156952, 7.347880794884117764E-16, 165.7703441132237003 ) ) ;
#16053=CARTESIAN_POINT ( 'NONE',  ( 20.99999999999999645, 6.646953231504538984, -1.265624999385487115 ) ) ;
#16058=VECTOR ( 'NONE', #10423, 1000.000000000000000 ) ;
#16062=( BOUNDED_CURVE ( )  B_SPLINE_CURVE ( 2, ( #1252, #26657, #24202, #24389, #3723, #21558, #33103, #32347, #15296, #687, #23828, #26849, #12258, #7147, #30262, #16611, #36863, #24754, #13765, #1816, #36304, #13574, #25311, #7889, #4474, #19282, #36683, #16053, #5031, #2374, #21741, #10908, #13949, #22485, #36124, #13385, #21925, #30822, #24937, #1632, #10165, #36492, #33472, #34031, #27601, #8075, #30457, #10535, #19650, #10721, #22295, #33290, #33848, #7516, #19088, #31192, #22112, #33660, #18904, #7700, #19463, #7331, #2184, #4845, #16424, #30640, #31010, #13204, #27970, #2001, #10352, #25127, #4656, #16239, #27789, #5217, #28153, #16793, #28338, #17536, #31925, #19834, #25686, #6142, #34769, #23402, #3300, #34951, #22853, #2560, #23220, #29070, #2742, #14495, #8811, #31555, #25497, #11644, #14130, #34403, #34216, #11285, #31374, #37235, #8441, #17719, #23036, #11466, #5957, #26230, #20009, #3114, #28706, #5579, #29260, #20384, #17165, #5395, #8261, #14315, #25868, #37050, #20566, #31742, #17350, #14681, #268, #37416, #11098, #34582, #8624, #20192, #5770, #28892, #2927, #26052, #80, #11831, #8996, #32109, #22671, #16975, #28517, #35132, #18669, #26609, #3488, #14871, #24343, #4050, #35884, #18480, #1200, #18101, #7100, #30020, #30211, #12397, #26418, #33053, #26798, #830, #9558, #29642, #21134, #3865, #32671, #18286, #638, #29828, #3679, #12207, #452, #15623, #24153, #20752, #35513, #15438, #32298, #21321, #12021, #9928, #9748, #12773, #17909, #6714, #6527, #26987, #23970, #1014, #9184, #35696, #23590, #21509, #12587, #15059, #6338, #32861, #35318, #23780, #6908, #27176, #29453, #9373, #20947, #32480, #15247, #30593, #19042 ),
 .UNSPECIFIED., .F., .F. ) 
 B_SPLINE_CURVE_WITH_KNOTS ( ( 3, 2, 2, 2, 2, 2, 2, 2, 2, 2, 2, 2, 2, 2, 2, 2, 2, 2, 2, 2, 2, 2, 2, 2, 2, 2, 2, 2, 2, 2, 2, 2, 2, 2, 2, 2, 2, 2, 2, 2, 2, 2, 2, 2, 2, 2, 2, 2, 2, 2, 2, 2, 2, 2, 2, 2, 2, 2, 2, 2, 2, 2, 2, 2, 2, 2, 2, 2, 2, 2, 2, 2, 2, 2, 2, 2, 2, 2, 2, 2, 2, 2, 2, 2, 2, 2, 2, 2, 2, 2, 2, 2, 2, 2, 2, 2, 2, 2, 2, 2, 2, 2, 2, 2, 3 ),
 ( 0.000000000000000000, 0.007246376811594203854, 0.01449275362318840771, 0.02173913043478261156, 0.02898550724637681542, 0.03623188405797101580, 0.04347826086956522312, 0.05072463768115942351, 0.05797101449275363083, 0.06521739130434782428, 0.07246376811594203160, 0.07971014492753622505, 0.08695652173913044625, 0.09420289855072463969, 0.1014492753623188470, 0.1086956521739130266, 0.1159420289855072617, 0.1231884057971014551, 0.1304347826086956486, 0.1376811594202898559, 0.1449275362318840632, 0.1521739130434782705, 0.1594202898550724501, 0.1666666666666666574, 0.1739130434782608925, 0.1811594202898550721, 0.1884057971014492794, 0.1956521739130434867, 0.2028985507246376940, 0.2101449275362318736, 0.2173913043478260532, 0.2246376811594203160, 0.2318840579710145233, 0.2391304347826087029, 0.2463768115942029102, 0.2536231884057971175, 0.2608695652173912971, 0.2681159420289855322, 0.2753623188405797118, 0.2826086956521738913, 0.2898550724637681264, 0.2971014492753623060, 0.3043478260869565410, 0.3115942028985507206, 0.3188405797101449002, 0.3260869565217391353, 0.3333333333333333148, 0.3405797101449275499, 0.3478260869565217850, 0.3550724637681159090, 0.3623188405797101441, 0.3695652173913043237, 0.3768115942028985588, 0.3840579710144927383, 0.3913043478260869734, 0.3985507246376811530, 0.4057971014492753881, 0.4130434782608695676, 0.4202898550724637472, 0.4275362318840579823, 0.4347826086956521063, 0.4420289855072463969, 0.4492753623188406320, 0.4565217391304347561, 0.4637681159420290466, 0.4710144927536231707, 0.4782608695652174058, 0.4855072463768115854, 0.4927536231884058204, 0.5000000000000000000, 0.5072463768115942351, 0.5144927536231883591, 0.5217391304347825942, 0.5289855072463768293, 0.5362318840579710644, 0.5434782608695651884, 0.5507246376811594235, 0.5579710144927536586, 0.5652173913043477826, 0.5724637681159420177, 0.5797101449275362528, 0.5869565217391304879, 0.5942028985507246119, 0.6014492753623188470, 0.6086956521739130821, 0.6159420289855072062, 0.6231884057971014412, 0.6304347826086956763, 0.6376811594202898004, 0.6449275362318840354, 0.6521739130434782705, 0.6594202898550725056, 0.6666666666666666297, 0.6739130434782608647, 0.6811594202898550998, 0.6884057971014492239, 0.6956521739130435700, 0.7028985507246376940, 0.7101449275362318181, 0.7173913043478260532, 0.7246376811594202882, 0.7318840579710145233, 0.7391304347826086474, 0.7463768115942028825, 0.7485758418660213298 ),
 .UNSPECIFIED. ) 
 CURVE ( )  GEOMETRIC_REPRESENTATION_ITEM ( )  RATIONAL_B_SPLINE_CURVE ( ( 1.000000000000000000, 0.8660254037844387076, 1.000000000000000000, 0.8660254037844387076, 1.000000000000000000, 0.8660254037844387076, 1.000000000000000000, 0.8660254037844387076, 1.000000000000000000, 0.8660254037844387076, 1.000000000000000000, 0.8660254037844387076, 1.000000000000000000, 0.8660254037844387076, 1.000000000000000000, 0.8660254037844387076, 1.000000000000000000, 0.8660254037844387076, 1.000000000000000000, 0.8660254037844387076, 1.000000000000000000, 0.8660254037844387076, 1.000000000000000000, 0.8660254037844387076, 1.000000000000000000, 0.8660254037844387076, 1.000000000000000000, 0.8660254037844387076, 1.000000000000000000, 0.8660254037844387076, 1.000000000000000000, 0.8660254037844387076, 1.000000000000000000, 0.8660254037844387076, 1.000000000000000000, 0.8660254037844387076, 1.000000000000000000, 0.8660254037844387076, 1.000000000000000000, 0.8660254037844387076, 1.000000000000000000, 0.8660254037844387076, 1.000000000000000000, 0.8660254037844387076, 1.000000000000000000, 0.8660254037844387076, 1.000000000000000000, 0.8660254037844387076, 1.000000000000000000, 0.8660254037844387076, 1.000000000000000000, 0.8660254037844387076, 1.000000000000000000, 0.8660254037844387076, 1.000000000000000000, 0.8660254037844387076, 1.000000000000000000, 0.8660254037844387076, 1.000000000000000000, 0.8660254037844387076, 1.000000000000000000, 0.8660254037844387076, 1.000000000000000000, 0.8660254037844387076, 1.000000000000000000, 0.8660254037844387076, 1.000000000000000000, 0.8660254037844387076, 1.000000000000000000, 0.8660254037844387076, 1.000000000000000000, 0.8660254037844387076, 1.000000000000000000, 0.8660254037844387076, 1.000000000000000000, 0.8660254037844387076, 1.000000000000000000, 0.8660254037844387076, 1.000000000000000000, 0.8660254037844387076, 1.000000000000000000, 0.8660254037844387076, 1.000000000000000000, 0.8660254037844387076, 1.000000000000000000, 0.8660254037844387076, 1.000000000000000000, 0.8660254037844387076, 1.000000000000000000, 0.8660254037844387076, 1.000000000000000000, 0.8660254037844387076, 1.000000000000000000, 0.8660254037844387076, 1.000000000000000000, 0.8660254037844387076, 1.000000000000000000, 0.8660254037844387076, 1.000000000000000000, 0.8660254037844387076, 1.000000000000000000, 0.8660254037844387076, 1.000000000000000000, 0.8660254037844387076, 1.000000000000000000, 0.8660254037844387076, 1.000000000000000000, 0.8660254037844387076, 1.000000000000000000, 0.8660254037844387076, 1.000000000000000000, 0.8660254037844387076, 1.000000000000000000, 0.8660254037844387076, 1.000000000000000000, 0.8660254037844387076, 1.000000000000000000, 0.8660254037844387076, 1.000000000000000000, 0.8660254037844387076, 1.000000000000000000, 0.8660254037844387076, 1.000000000000000000, 0.8660254037844387076, 1.000000000000000000, 0.8660254037844387076, 1.000000000000000000, 0.8660254037844387076, 1.000000000000000000, 0.8660254037844387076, 1.000000000000000000, 0.8660254037844387076, 1.000000000000000000, 0.8660254037844387076, 1.000000000000000000, 0.8660254037844387076, 1.000000000000000000, 0.8660254037844387076, 1.000000000000000000, 0.8660254037844387076, 1.000000000000000000, 0.8660254037844387076, 1.000000000000000000, 0.8660254037844387076, 1.000000000000000000, 0.8660254037844387076, 1.000000000000000000, 0.8660254037844387076, 1.000000000000000000, 0.8660254037844387076, 1.000000000000000000, 0.8660254037844387076, 1.000000000000000000, 0.8660254037844387076, 1.000000000000000000, 0.8660254037844387076, 1.000000000000000000, 0.8660254037844387076, 1.000000000000000000, 0.8660254037844387076, 1.000000000000000000, 0.8660254037844387076, 1.000000000000000000, 0.8660254037844387076, 1.000000000000000000, 0.8660254037844387076, 1.000000000000000000, 0.8660254037844387076, 1.000000000000000000, 0.8660254037844387076, 1.000000000000000000, 0.8660254037844387076, 1.000000000000000000, 0.8660254037844387076, 1.000000000000000000, 0.8660254037844387076, 1.000000000000000000, 0.8660254037844387076, 1.000000000000000000, 0.8660254037844387076, 1.000000000000000000, 0.8660254037844387076, 1.000000000000000000, 0.8660254037844387076, 1.000000000000000000, 0.8660254037844387076, 1.000000000000000000, 0.8660254037844387076, 1.000000000000000000, 0.8660254037844387076, 1.000000000000000000, 0.8660254037844387076, 1.000000000000000000, 0.8660254037844387076, 1.000000000000000000, 0.8660254037844387076, 1.000000000000000000, 0.8660254037844387076, 1.000000000000000000, 0.8660254037844387076, 1.000000000000000000, 0.8660254037844387076, 1.000000000000000000, 0.8660254037844387076, 1.000000000000000000, 0.8660254037844387076, 1.000000000000000000, 0.9593432414028914001, 0.9433623850486823059 ) ) 
 REPRESENTATION_ITEM ( '' )  );
#16063=CARTESIAN_POINT ( 'NONE',  ( 31.03952447949476223, 7.209453229046482114, 164.7522898954867401 ) ) ;
#16077=ORIENTED_EDGE ( 'NONE', *, *, #4990, .T. ) ;
#16078=CARTESIAN_POINT ( 'NONE',  ( 15.00000000000000178, -3.464101615137757051, -3.112500000000005596 ) ) ;
#16079=CARTESIAN_POINT ( 'NONE',  ( 37.09591843811324452, 3.604726614523243278, 162.3402618868670118 ) ) ;
#16080=CARTESIAN_POINT ( 'NONE',  ( 33.67594490067671842, -5.196152422706635576, 160.4655734646546534 ) ) ;
#16085=ORIENTED_EDGE ( 'NONE', *, *, #23832, .T. ) ;
#16089=CARTESIAN_POINT ( 'NONE',  ( 18.12178482187499640, 4.985214923628404904, -7.528124999385488181 ) ) ;
#16100=( BOUNDED_CURVE ( )  B_SPLINE_CURVE ( 2, ( #33665, #33478, #18537, #33297, #7706, #7153, #24578 ),
 .UNSPECIFIED., .F., .F. ) 
 B_SPLINE_CURVE_WITH_KNOTS ( ( 3, 2, 2, 3 ),
 ( 0.7608695652173899093, 0.7681159420289840334, 0.7753623188405783795, 0.7826086956521726146 ),
 .UNSPECIFIED. ) 
 CURVE ( )  GEOMETRIC_REPRESENTATION_ITEM ( )  RATIONAL_B_SPLINE_CURVE ( ( 1.000000000000026645, 0.8660254037844120623, 1.000000000000000000, 0.8660254037844387076, 1.000000000000000000, 0.8660254037844633546, 0.9999999999999753530 ) ) 
 REPRESENTATION_ITEM ( '' )  );
#16103=EDGE_CURVE ( 'NONE', #2107, #13050, #10264, .T. ) ;
#16105=CARTESIAN_POINT ( 'NONE',  ( 30.75027635825099281, -7.209453229046475009, 161.4461687411947821 ) ) ;
#16107=CARTESIAN_POINT ( 'NONE',  ( 24.89321967762106169, 0.000000000000000000, 163.3419840153761982 ) ) ;
#16115=CARTESIAN_POINT ( 'NONE',  ( 37.13350435217314782, -3.604726614523235284, 162.7698708504190392 ) ) ;
#16116=CARTESIAN_POINT ( 'NONE',  ( 21.00000000000000000, 6.646953231504538984, -4.753124999385462068 ) ) ;
#16117=ADVANCED_FACE ( 'NONE', ( #5160 ), #33976, .T. ) ;
#16119=CARTESIAN_POINT ( 'NONE',  ( 37.34107544803060108, 3.464101615137759271, 167.9370675803488666 ) ) ;
#16122=CARTESIAN_POINT ( 'NONE',  ( 25.05990503573306682, 0.000000000000000000, 165.2472063767010013 ) ) ;
#16125=ORIENTED_EDGE ( 'NONE', *, *, #23212, .T. ) ;
#16126=ORIENTED_EDGE ( 'NONE', *, *, #5885, .F. ) ;
#16128=AXIS2_PLACEMENT_3D ( 'NONE', #2101, #19188, #19377 ) ;
#16130=CARTESIAN_POINT ( 'NONE',  ( 21.00000000000000000, 6.646953231504538984, -3.853124999385470595 ) ) ;
#16132=CARTESIAN_POINT ( 'NONE',  ( 21.00000000000000000, -6.928203230275506996, -9.281249998770942256 ) ) ;
#16134=ORIENTED_EDGE ( 'NONE', *, *, #9448, .T. ) ;
#16138=CARTESIAN_POINT ( 'NONE',  ( 24.51248951003896437, 3.604726614523240613, 161.7848665344110657 ) ) ;
#16152=VECTOR ( 'NONE', #19557, 1000.000000000000000 ) ;
#16174=CARTESIAN_POINT ( 'NONE',  ( 21.00000000000000000, -6.646953231504538984, -5.990624999385490312 ) ) ;
#16177=ORIENTED_EDGE ( 'NONE', *, *, #11731, .T. ) ;
#16178=CARTESIAN_POINT ( 'NONE',  ( 26.75643035624999655, 7.049594010296217766E-16, -7.565624999385455851 ) ) ;
#16181=CARTESIAN_POINT ( 'NONE',  ( 34.48606902399273366, -5.407089921784861808, 168.3280104420172449 ) ) ;
#16197=DIRECTION ( 'NONE',  ( 0.08715574274765150453, 0.000000000000000000, 0.9961946980917461003 ) ) ;
#16210=ORIENTED_EDGE ( 'NONE', *, *, #26275, .T. ) ;
#16214=CARTESIAN_POINT ( 'NONE',  ( 31.02481694790609268, -7.209453229046475009, 164.5841820401837765 ) ) ;
#16220=VERTEX_POINT ( 'NONE', #11226 ) ;
#16221=CARTESIAN_POINT ( 'NONE',  ( 26.99999999999999645, 3.464101615137755275, -5.981249998770952203 ) ) ;
#16224=CARTESIAN_POINT ( 'NONE',  ( 26.97716818855048260, 0.000000000000000000, 49.47706554351410801 ) ) ;
#16225=CARTESIAN_POINT ( 'NONE',  ( 26.75643035624999655, 7.049594010296217766E-16, -8.915624999385475036 ) ) ;
#16234=CARTESIAN_POINT ( 'NONE',  ( 34.11717084844381986, -5.196152422706629359, 165.5088091249684510 ) ) ;
#16239=CARTESIAN_POINT ( 'NONE',  ( 15.24356964374999990, 3.323476615752268604, -2.990624999385476102 ) ) ;
#16248=CARTESIAN_POINT ( 'NONE',  ( 25.44556919728433542, -3.464101615137774814, 169.6553679145326612 ) ) ;
#16249=CARTESIAN_POINT ( 'NONE',  ( 30.96108431102187808, 7.209453229046482114, 163.8557146672041824 ) ) ;
#16254=CARTESIAN_POINT ( 'NONE',  ( 26.99999999999999645, 7.347880794884117764E-16, -6.918749998770956644 ) ) ;
#16257=CARTESIAN_POINT ( 'NONE',  ( 24.00000000000000000, -5.196152422706629359, -7.893749998770960730 ) ) ;
#16264=CARTESIAN_POINT ( 'NONE',  ( 26.99999999999999645, -3.464101615137751278, -1.612499999999998046 ) ) ;
#16265=CARTESIAN_POINT ( 'NONE',  ( 27.85444716323975101, 5.407089921784862696, 164.1651534432314747 ) ) ;
#16266=CARTESIAN_POINT ( 'NONE',  ( 24.69711925643884598, 0.000000000000000000, 161.1005459446697614 ) ) ;
#16276=CARTESIAN_POINT ( 'NONE',  ( 25.24620043574905282, 0.000000000000000000, 167.3765725426477502 ) ) ;
#16278=CARTESIAN_POINT ( 'NONE',  ( 15.24356964374999990, 0.000000000000000000, -7.453124999385495997 ) ) ;
#16290=CARTESIAN_POINT ( 'NONE',  ( 24.48144027668511669, 0.000000000000000000, 161.4299721732159014 ) ) ;
#16291=CARTESIAN_POINT ( 'NONE',  ( 23.99999999999999645, 5.196152422706631135, -0.9937499987709430549 ) ) ;
#16300=CARTESIAN_POINT ( 'NONE',  ( 24.75598086634022010, 0.000000000000000000, 164.5679854722048958 ) ) ;
#16301=CARTESIAN_POINT ( 'NONE',  ( 21.00000000000000000, -6.646953231504538984, -5.428124999385471661 ) ) ;
#16303=CARTESIAN_POINT ( 'NONE',  ( 17.39339328860229728, 4.563019727067374909, -8.000000000000001776 ) ) ;
#16304=CARTESIAN_POINT ( 'NONE',  ( 31.37044394018619542, 6.928203230275514990, 168.5347166391916574 ) ) ;
#16305=CARTESIAN_POINT ( 'NONE',  ( 24.69711925643884598, 0.000000000000000000, 161.1005459446697614 ) ) ;
#16314=CARTESIAN_POINT ( 'NONE',  ( 15.02283181144952628, 7.347880794884122694E-16, 50.52293445648592751 ) ) ;
#16315=CARTESIAN_POINT ( 'NONE',  ( 21.00000000000000000, -6.646953231504538984, -4.978124999385476812 ) ) ;
#16317=CARTESIAN_POINT ( 'NONE',  ( 23.99999999999999645, 5.196152422706631135, -9.993749998770951493 ) ) ;
#16319=( BOUNDED_CURVE ( )  B_SPLINE_CURVE ( 2, ( #2565, #5584, #17170, #33853, #5223, #28712, #14320 ),
 .UNSPECIFIED., .F., .F. ) 
 B_SPLINE_CURVE_WITH_KNOTS ( ( 3, 2, 2, 3 ),
 ( 0.5434782608695641892, 0.5507246376811585353, 0.5579710144927527704, 0.5652173913043470055 ),
 .UNSPECIFIED. ) 
 CURVE ( )  GEOMETRIC_REPRESENTATION_ITEM ( )  RATIONAL_B_SPLINE_CURVE ( ( 1.000000000000018430, 0.8660254037844202779, 1.000000000000000000, 0.8660254037844387076, 1.000000000000000000, 0.8660254037844530295, 0.9999999999999856781 ) ) 
 REPRESENTATION_ITEM ( '' )  );
#16332=ORIENTED_EDGE ( 'NONE', *, *, #15497, .T. ) ;
#16350=CARTESIAN_POINT ( 'NONE',  ( 18.00000000000000000, 5.196152422706630247, -9.525000000000005684 ) ) ;
#16351=ORIENTED_EDGE ( 'NONE', *, *, #27045, .F. ) ;
#16354=ADVANCED_FACE ( 'NONE', ( #23351 ), #8946, .T. ) ;
#16357=CARTESIAN_POINT ( 'NONE',  ( 23.87821517812499650, 4.985214923628404904, -6.703124999385495997 ) ) ;
#16373=CARTESIAN_POINT ( 'NONE',  ( 18.00000000000000000, 5.196152422706630247, -6.824999999999997513 ) ) ;
#16378=DIRECTION ( 'NONE',  ( 0.000000000000000000, 0.000000000000000000, 1.000000000000000000 ) ) ;
#16382=EDGE_CURVE ( 'NONE', #22329, #36867, #2733, .T. ) ;
#16385=VERTEX_POINT ( 'NONE', #29405 ) ;
#16401=CARTESIAN_POINT ( 'NONE',  ( 36.94394061169700905, 3.604726614523238837, 160.6031473820695226 ) ) ;
#16402=CARTESIAN_POINT ( 'NONE',  ( 15.24356964374999990, 3.323476615752268604, -0.7406249993854975289 ) ) ;
#16404=ORIENTED_EDGE ( 'NONE', *, *, #19300, .T. ) ;
#16406=ORIENTED_EDGE ( 'NONE', *, *, #34019, .T. ) ;
#16408=CARTESIAN_POINT ( 'NONE',  ( 24.00000000000000000, -5.196152422706629359, -5.193749998770952558 ) ) ;
#16409=CARTESIAN_POINT ( 'NONE',  ( 23.87821517812500005, -4.985214923628404016, -0.8906249993854697955 ) ) ;
#16410=CARTESIAN_POINT ( 'NONE',  ( 27.80663194388356629, 5.196152422706630247, 162.2212988612534730 ) ) ;
#16419=CARTESIAN_POINT ( 'NONE',  ( 33.99951059573448475, -5.196152422706629359, 164.1639462825446003 ) ) ;
#16424=CARTESIAN_POINT ( 'NONE',  ( 23.87821517812499650, 4.985214923628404904, -2.653124999385497951 ) ) ;
#16433=CARTESIAN_POINT ( 'NONE',  ( 27.97210741594907901, 5.407089921784862696, 165.5100162856553538 ) ) ;
#16448=CARTESIAN_POINT ( 'NONE',  ( 15.00000000000021316, -3.464101615137879620, -6.206249998770965171 ) ) ;
#16450=CARTESIAN_POINT ( 'NONE',  ( 15.00000000000000178, -3.464101615137757051, -2.662500000000009415 ) ) ;
#16451=CARTESIAN_POINT ( 'NONE',  ( 26.48145948632588187, -2.034413479899699340, -8.000000000000001776 ) ) ;
#16452=CARTESIAN_POINT ( 'NONE',  ( 24.71185827157421855, 0.000000000000000000, 164.0636619062959483 ) ) ;
#16453=CARTESIAN_POINT ( 'NONE',  ( 33.64979817785242489, 5.196152422706637353, 160.1667150552271437 ) ) ;
#16464=CARTESIAN_POINT ( 'NONE',  ( 26.75643035624999655, -3.323476615752267715, -8.615624999385470772 ) ) ;
#16477=CARTESIAN_POINT ( 'NONE',  ( 27.58480908411420529, 5.407089921784856479, 161.0831760960101349 ) ) ;
#16478=CARTESIAN_POINT ( 'NONE',  ( 21.00000000000000000, -6.928203230275506996, -1.181249998770955267 ) ) ;
#16488=CARTESIAN_POINT ( 'NONE',  ( 37.29692136982500728, 3.604726614523238837, 164.6377359093410746 ) ) ;
#16489=CARTESIAN_POINT ( 'NONE',  ( 26.75643035624999655, -3.323476615752267715, -6.253124999385469174 ) ) ;
#16491=CARTESIAN_POINT ( 'NONE',  ( 37.64173127707041289, 7.646167579472024665E-16, 168.5789311836665831 ) ) ;
#16492=CARTESIAN_POINT ( 'NONE',  ( 25.32137226386890205, 3.464101615137757051, 168.2357904697519189 ) ) ;
#16498=ORIENTED_EDGE ( 'NONE', *, *, #11242, .T. ) ;
#16502=CARTESIAN_POINT ( 'NONE',  ( 26.75643035624999655, 3.323476615752271712, -4.378124999385460292 ) ) ;
#16504=CARTESIAN_POINT ( 'NONE',  ( 26.99999999999999645, 7.347880794884117764E-16, -2.868749998770958598 ) ) ;
#16505=CARTESIAN_POINT ( 'NONE',  ( 26.75643035624999655, 3.323476615752271712, -1.340624999385481075 ) ) ;
#16506=EDGE_CURVE ( 'NONE', #5916, #20921, #9882, .T. ) ;
#16527=FACE_OUTER_BOUND ( 'NONE', #7120, .T. ) ;
#16532=CARTESIAN_POINT ( 'NONE',  ( 15.02283181144952628, 7.347880794884122694E-16, 50.52293445648592751 ) ) ;
#16545=CARTESIAN_POINT ( 'NONE',  ( 15.24356964374999990, 0.000000000000000000, -7.903124999385474858 ) ) ;
#16552=CARTESIAN_POINT ( 'NONE',  ( 31.35328515338631306, 7.209453229046482114, 168.3385908086170559 ) ) ;
#16554=CARTESIAN_POINT ( 'NONE',  ( 28.40800656884236730, -5.196152422706632912, 169.0950422780865097 ) ) ;
#16578=CIRCLE ( 'NONE', #3849, 3.999999999999996447 ) ;
#16588=CARTESIAN_POINT ( 'NONE',  ( 33.91574363238778034, 5.407089921784857367, 161.8091613863793725 ) ) ;
#16592=ORIENTED_EDGE ( 'NONE', *, *, #7515, .T. ) ;
#16594=ORIENTED_EDGE ( 'NONE', *, *, #88, .F. ) ;
#16595=CARTESIAN_POINT ( 'NONE',  ( 26.99999999999999645, -3.464101615137751278, -5.156249998770954690 ) ) ;
#16596=CARTESIAN_POINT ( 'NONE',  ( 23.87821517812500005, -4.985214923628404016, -2.690624999385465621 ) ) ;
#16599=CARTESIAN_POINT ( 'NONE',  ( 26.99999999999983658, 3.464101615137847645, -6.037499999999991651 ) ) ;
#16600=LINE ( 'NONE', #20000, #22663 ) ;
#16606=CARTESIAN_POINT ( 'NONE',  ( 25.10239346032254915, -3.464101615137757051, 165.7328512920207402 ) ) ;
#16611=CARTESIAN_POINT ( 'NONE',  ( 20.99999999999999645, 6.646953231504538984, -0.8156249993854914893 ) ) ;
#16620=CARTESIAN_POINT ( 'NONE',  ( 24.90469035240339934, 3.604726614523240613, 166.2677426758239108 ) ) ;
#16628=CARTESIAN_POINT ( 'NONE',  ( 15.00000000000000178, 0.000000000000000000, -3.599999999999992095 ) ) ;
#16633=CARTESIAN_POINT ( 'NONE',  ( 15.00000000000000000, 0.000000000000000000, -2.193749998770949894 ) ) ;
#16638=CARTESIAN_POINT ( 'NONE',  ( 21.00000000000000000, 6.928203230275506996, -3.262499999999993516 ) ) ;
#16639=CARTESIAN_POINT ( 'NONE',  ( 21.68347279894478774, -5.929004884096451988, -8.000000000000005329 ) ) ;
#16640=CARTESIAN_POINT ( 'NONE',  ( 30.72576380560321851, 7.209453229046482114, 161.1659889823564811 ) ) ;
#16642=CARTESIAN_POINT ( 'NONE',  ( 28.29077060037018043, 5.407089921784856479, 169.1523531505532674 ) ) ;
#16649=CARTESIAN_POINT ( 'NONE',  ( 28.24132121073036927, -5.196152422706638241, 167.1898199167616781 ) ) ;
#16651=CARTESIAN_POINT ( 'NONE',  ( 26.75643035624999655, 3.323476615752271712, -8.990624999385502747 ) ) ;
#16654=CARTESIAN_POINT ( 'NONE',  ( 15.00000000000058620, 3.464101615138089674, -7.237500000000000711 ) ) ;
#16656=CARTESIAN_POINT ( 'NONE',  ( 31.09590335053109555, 6.928203230275514990, 165.3967033402026914 ) ) ;
#16660=ADVANCED_FACE ( 'NONE', ( #18624 ), #29972, .T. ) ;
#16664=CARTESIAN_POINT ( 'NONE',  ( 33.90267027097563357, -5.407089921784855591, 161.6597321816656176 ) ) ;
#16676=CARTESIAN_POINT ( 'NONE',  ( 34.17721086063072988, -5.407089921784855591, 164.7977454806546120 ) ) ;
#16677=CARTESIAN_POINT ( 'NONE',  ( 15.24356964375000167, -3.323476615752272600, -4.153124999385478411 ) ) ;
#16679=CARTESIAN_POINT ( 'NONE',  ( 34.36840877128340566, -5.407089921784861808, 166.9831475995933943 ) ) ;
#16680=CARTESIAN_POINT ( 'NONE',  ( 37.18419511108482567, 3.464101615137759271, 166.1439171237837229 ) ) ;
#16684=VECTOR ( 'NONE', #24774, 1000.000000000000000 ) ;
#16691=CARTESIAN_POINT ( 'NONE',  ( 26.75643035624999655, 7.049594010296217766E-16, -3.965624999385464200 ) ) ;
#16694=CARTESIAN_POINT ( 'NONE',  ( 15.24356964374999990, 0.000000000000000000, -1.153124999385496396 ) ) ;
#16706=AXIS2_PLACEMENT_3D ( 'NONE', #29675, #9406, #35169 ) ;
#16709=DIRECTION ( 'NONE',  ( 0.08715574274765142126, 0.000000000000000000, 0.9961946980917461003 ) ) ;
#16715=ORIENTED_EDGE ( 'NONE', *, *, #27441, .F. ) ;
#16722=CARTESIAN_POINT ( 'NONE',  ( 15.00000000000000355, 7.347880794884112834E-16, -8.000000000000000000 ) ) ;
#16723=DIRECTION ( 'NONE',  ( 1.000000000000000000, 0.000000000000000000, 0.000000000000000000 ) ) ;
#16725=CARTESIAN_POINT ( 'NONE',  ( 26.99999999999999645, 3.464101615137755275, -8.737500000000000711 ) ) ;
#16730=CARTESIAN_POINT ( 'NONE',  ( 23.87821517812499650, 4.985214923628404904, -7.153124999385473970 ) ) ;
#16735=CARTESIAN_POINT ( 'NONE',  ( 25.10079077358561150, 3.604726614523240613, 168.5091807465304043 ) ) ;
#16757=CARTESIAN_POINT ( 'NONE',  ( 37.23322021648719726, 3.464101615137916035, 166.7042766426847322 ) ) ;
#16765=DIRECTION ( 'NONE',  ( 0.000000000000000000, 0.000000000000000000, 1.000000000000000000 ) ) ;
#16770=CARTESIAN_POINT ( 'NONE',  ( 30.84832656884210067, 7.209453229046475009, 162.5668877765479863 ) ) ;
#16771=CARTESIAN_POINT ( 'NONE',  ( 15.00000000000000355, 7.347880794884112834E-16, -8.000000000000000000 ) ) ;
#16773=EDGE_CURVE ( 'NONE', #29577, #31993, #12730, .T. ) ;
#16774=ORIENTED_EDGE ( 'NONE', *, *, #8770, .T. ) ;
#16777=CARTESIAN_POINT ( 'NONE',  ( 18.00000000000000000, 5.196152422706630247, -4.518749998770942966 ) ) ;
#16778=CARTESIAN_POINT ( 'NONE',  ( 15.24356964374999990, 0.000000000000000000, -1.940624999385465177 ) ) ;
#16788=CARTESIAN_POINT ( 'NONE',  ( 33.96029051149804445, -5.196152422706629359, 163.7156586684033073 ) ) ;
#16793=CARTESIAN_POINT ( 'NONE',  ( 26.75643035624999655, 3.323476615752271268, -3.140624999385464022 ) ) ;
#16800=CARTESIAN_POINT ( 'NONE',  ( 15.00000000000000000, 0.000000000000000000, -7.200000000000011724 ) ) ;
#16804=DIRECTION ( 'NONE',  ( 0.08715574274765150453, 0.000000000000000000, 0.9961946980917461003 ) ) ;
#16805=CARTESIAN_POINT ( 'NONE',  ( 24.59092967851185207, 3.604726614523240613, 162.6814417626936518 ) ) ;
#16810=CARTESIAN_POINT ( 'NONE',  ( 27.70204505258639216, -5.196152422706632912, 161.0258652235433487 ) ) ;
#16820=CARTESIAN_POINT ( 'NONE',  ( 15.00000000000000000, 0.000000000000000000, -3.599999999999992095 ) ) ;
#16822=CARTESIAN_POINT ( 'NONE',  ( 24.35560917309319251, 3.604726614523240613, 159.9917160778459220 ) ) ;
#16824=CARTESIAN_POINT ( 'NONE',  ( 25.14491336835161306, 3.604726614523236616, 169.0135043124392951 ) ) ;
#16828=ORIENTED_EDGE ( 'NONE', *, *, #26777, .T. ) ;
#16831=CARTESIAN_POINT ( 'NONE',  ( 30.75272761356932705, 6.928203230275506996, 161.4741867176907988 ) ) ;
#16834=CARTESIAN_POINT ( 'NONE',  ( 23.87821517812500005, -4.985214923628404016, -8.203124999385469351 ) ) ;
#16836=( BOUNDED_CURVE ( )  B_SPLINE_CURVE ( 2, ( #26438, #28723, #5789, #37436, #29471, #470, #3507 ),
 .UNSPECIFIED., .F., .F. ) 
 B_SPLINE_CURVE_WITH_KNOTS ( ( 3, 2, 2, 3 ),
 ( 0.3913043478260864183, 0.3985507246376804869, 0.4057971014492746109, 0.4130434782608686795 ),
 .UNSPECIFIED. ) 
 CURVE ( )  GEOMETRIC_REPRESENTATION_ITEM ( )  RATIONAL_B_SPLINE_CURVE ( ( 1.000000000000010214, 0.8660254037844284936, 1.000000000000000000, 0.8660254037844387076, 1.000000000000000000, 0.8660254037844551389, 0.9999999999999835687 ) ) 
 REPRESENTATION_ITEM ( '' )  );
#16839=CARTESIAN_POINT ( 'NONE',  ( 18.00000000000000000, 5.196152422706630247, -7.275000000000003908 ) ) ;
#16840=CARTESIAN_POINT ( 'NONE',  ( 24.55170959427540822, 3.604726614523240613, 162.2331541485523587 ) ) ;
#16852=CARTESIAN_POINT ( 'NONE',  ( 37.56329110859752518, 7.646167579472024665E-16, 167.6823559553839971 ) ) ;
#16861=VERTEX_POINT ( 'NONE', #10626 ) ;
#16862=CARTESIAN_POINT ( 'NONE',  ( 36.94394061169700905, 3.604726614523238837, 160.6031473820695226 ) ) ;
#16863=CARTESIAN_POINT ( 'NONE',  ( 21.00000000000000000, -6.646953231504538984, -4.528124999385448213 ) ) ;
#16865=CARTESIAN_POINT ( 'NONE',  ( 37.59924285248093412, -3.604726614523238837, 168.0932862683468159 ) ) ;
#16866=CARTESIAN_POINT ( 'NONE',  ( 25.16449192692313019, 3.464101615137757051, 166.4426400131867467 ) ) ;
#16867=CARTESIAN_POINT ( 'NONE',  ( 27.00000000000013500, 3.464101615137676227, -0.1875000000000186240 ) ) ;
#16874=( BOUNDED_CURVE ( )  B_SPLINE_CURVE ( 2, ( #1175, #9531, #12749, #26956, #986, #34919, #8963 ),
 .UNSPECIFIED., .F., .F. ) 
 B_SPLINE_CURVE_WITH_KNOTS ( ( 3, 2, 2, 3 ),
 ( 0.1304347826086947049, 0.1376811594202889955, 0.1449275362318833138, 0.1521739130434776044 ),
 .UNSPECIFIED. ) 
 CURVE ( )  GEOMETRIC_REPRESENTATION_ITEM ( )  RATIONAL_B_SPLINE_CURVE ( ( 1.000000000000017319, 0.8660254037844211661, 1.000000000000000000, 0.8660254037844387076, 1.000000000000000000, 0.8660254037844510311, 0.9999999999999876765 ) ) 
 REPRESENTATION_ITEM ( '' )  );
#16880=CARTESIAN_POINT ( 'NONE',  ( 26.75643035624999655, 7.049594010296217766E-16, -2.728124999385489247 ) ) ;
#16906=EDGE_CURVE ( 'NONE', #26157, #12608, #28250, .T. ) ;
#16907=CARTESIAN_POINT ( 'NONE',  ( 27.97658564224149558, -5.196152422706632912, 164.1638785225323431 ) ) ;
#16908=FACE_OUTER_BOUND ( 'NONE', #29343, .T. ) ;
#16910=CARTESIAN_POINT ( 'NONE',  ( 26.99999999999999645, 3.464101615137755275, -9.637499999999990408 ) ) ;
#16916=CARTESIAN_POINT ( 'NONE',  ( 26.75643035624999655, 3.323476615752271712, -7.640624999385485339 ) ) ;
#16922=CARTESIAN_POINT ( 'NONE',  ( 37.56655944895057075, 3.604726614523243278, 167.7197132565624713 ) ) ;
#16928=CARTESIAN_POINT ( 'NONE',  ( 28.25155051613373658, 5.407089921784856479, 168.7040655364119743 ) ) ;
#16931=CARTESIAN_POINT ( 'NONE',  ( 20.99999999999999645, 6.928203230275506996, -1.406249998770969123 ) ) ;
#16938=ORIENTED_EDGE ( 'NONE', *, *, #11477, .T. ) ;
#16949=EDGE_LOOP ( 'NONE', ( #29213, #10701, #27123 ) ) ;
#16955=CARTESIAN_POINT ( 'NONE',  ( 36.97989235558041798, 7.646167579472015790E-16, 161.0140776950323698 ) ) ;
#16958=VERTEX_POINT ( 'NONE', #8717 ) ;
#16961=CARTESIAN_POINT ( 'NONE',  ( 21.00000000000000000, -6.928203230275506996, -7.481249998770959309 ) ) ;
#16962=CARTESIAN_POINT ( 'NONE',  ( 20.99999999999999645, -6.646953231504538984, -2.278124999385469529 ) ) ;
#16963=CARTESIAN_POINT ( 'NONE',  ( 18.00000000000000000, 5.196152422706630247, -6.374999999999992006 ) ) ;
#16971=CARTESIAN_POINT ( 'NONE',  ( 25.05990503573306682, 0.000000000000000000, 165.2472063767010013 ) ) ;
#16975=CARTESIAN_POINT ( 'NONE',  ( 20.99999999999999645, -6.646953231504538984, -5.540624999385494576 ) ) ;
#16976=CARTESIAN_POINT ( 'NONE',  ( 18.00000000000000000, 5.196152422706630247, -0.5249999999999976907 ) ) ;
#16979=VERTEX_POINT ( 'NONE', #3020 ) ;
#16984=DIRECTION ( 'NONE',  ( 1.000000000000000000, 0.000000000000000000, -0.000000000000000000 ) ) ;
#16985=CARTESIAN_POINT ( 'NONE',  ( 37.12860184164360788, -3.604726614523238837, 162.7138348986514131 ) ) ;
#16987=EDGE_CURVE ( 'NONE', #5563, #6369, #32286, .T. ) ;
#16991=CARTESIAN_POINT ( 'NONE',  ( 25.12854018303972126, 0.000000000000000000, 166.0317097002238995 ) ) ;
#17000=CARTESIAN_POINT ( 'NONE',  ( 21.00000000000000000, -6.928203230275506996, -5.287499999999990763 ) ) ;
#17001=FACE_OUTER_BOUND ( 'NONE', #11210, .T. ) ;
#17002=CARTESIAN_POINT ( 'NONE',  ( 36.82137784845814821, 3.604726614523243278, 159.2022485878780174 ) ) ;
#17004=CARTESIAN_POINT ( 'NONE',  ( 36.59589384753818564, 3.464101615137759271, 159.4196029116644695 ) ) ;
#17009=EDGE_LOOP ( 'NONE', ( #34505, #5539, #5632, #7633 ) ) ;
#17012=CARTESIAN_POINT ( 'NONE',  ( 15.00000000000021316, 3.464101615137874735, -4.931249998770944387 ) ) ;
#17014=CARTESIAN_POINT ( 'NONE',  ( 23.87821517812499650, 4.985214923628404904, -8.953124999385497773 ) ) ;
#17019=CARTESIAN_POINT ( 'NONE',  ( 26.99999999999999645, 7.347880794884117764E-16, -6.468749998770951137 ) ) ;
#17020=CARTESIAN_POINT ( 'NONE',  ( 24.59746635921792546, -3.604726614523244610, 162.7561563650505150 ) ) ;
#17033=CARTESIAN_POINT ( 'NONE',  ( 27.46714883140487373, 5.407089921784856479, 159.7383132535862842 ) ) ;
#17034=CARTESIAN_POINT ( 'NONE',  ( 18.00000000000000355, -5.196152422706632912, -0.7687499987709400795 ) ) ;
#17038=DIRECTION ( 'NONE',  ( 0.08715574274765150453, 0.000000000000000000, 0.9961946980917461003 ) ) ;
#17044=CARTESIAN_POINT ( 'NONE',  ( 36.97989235558041798, 7.646167579472015790E-16, 161.0140776950323698 ) ) ;
#17045=CARTESIAN_POINT ( 'NONE',  ( 26.75643035624999655, 3.323476615752271712, -8.878124999385482496 ) ) ;
#17047=CARTESIAN_POINT ( 'NONE',  ( 34.38148213269554532, 5.407089921784862696, 167.1325768043071776 ) ) ;
#17048=CARTESIAN_POINT ( 'NONE',  ( 25.17102860762920713, -3.464101615137761048, 166.5173546155436100 ) ) ;
#17049=CARTESIAN_POINT ( 'NONE',  ( 26.99999999999999645, 7.347880794884117764E-16, -2.418749998770952647 ) ) ;
#17052=( BOUNDED_CURVE ( )  B_SPLINE_CURVE ( 2, ( #26595, #626, #3478, #23208, #5944, #3666, #9172 ),
 .UNSPECIFIED., .F., .F. ) 
 B_SPLINE_CURVE_WITH_KNOTS ( ( 3, 2, 2, 3 ),
 ( 0.9130434782608682909, 0.9202898550724624149, 0.9275362318840564280, 0.9347826086956505520 ),
 .UNSPECIFIED. ) 
 CURVE ( )  GEOMETRIC_REPRESENTATION_ITEM ( )  RATIONAL_B_SPLINE_CURVE ( ( 1.000000000000022649, 0.8660254037844161701, 1.000000000000000000, 0.8660254037844387076, 1.000000000000000000, 0.8660254037844694608, 0.9999999999999692468 ) ) 
 REPRESENTATION_ITEM ( '' )  );
#17056=ORIENTED_EDGE ( 'NONE', *, *, #34648, .T. ) ;
#17058=EDGE_CURVE ( 'NONE', #2107, #2079, #31647, .T. ) ;
#17062=CARTESIAN_POINT ( 'NONE',  ( 15.24356964374999990, 3.323476615752268604, -1.640624999385488891 ) ) ;
#17079=CARTESIAN_POINT ( 'NONE',  ( 37.33453876732481547, -3.464101615137594514, 167.8623529779919750 ) ) ;
#17084=CARTESIAN_POINT ( 'NONE',  ( 37.64663378759995283, 7.646167579472015790E-16, 168.6349671354342092 ) ) ;
#17088=CARTESIAN_POINT ( 'NONE',  ( 23.87821517812500005, -4.985214923628404016, -0.4406249993854638447 ) ) ;
#17089=CARTESIAN_POINT ( 'NONE',  ( 27.00000000000063238, 3.464101615137388013, -5.137500000000009948 ) ) ;
#17095=CARTESIAN_POINT ( 'NONE',  ( 15.00000000000000000, 3.464101615137752166, -8.587500000000012790 ) ) ;
#17101=CARTESIAN_POINT ( 'NONE',  ( 26.75643035624999655, 3.323476615752271712, -8.540624999385476812 ) ) ;
#17103=ORIENTED_EDGE ( 'NONE', *, *, #26558, .F. ) ;
#17106=CARTESIAN_POINT ( 'NONE',  ( 25.02561894546576582, 0.000000000000000000, 167.6499628194262357 ) ) ;
#17118=CARTESIAN_POINT ( 'NONE',  ( 18.00000000000000000, 5.196152422706630247, -0.4687499987709453642 ) ) ;
#17124=EDGE_CURVE ( 'NONE', #10985, #31911, #18027, .T. ) ;
#17130=CARTESIAN_POINT ( 'NONE',  ( 30.89980292934887629, 6.928203230275514990, 163.1552652694962546 ) ) ;
#17131=DIRECTION ( 'NONE',  ( 0.08715574274765143514, 0.000000000000000000, 0.9961946980917462113 ) ) ;
#17132=DIRECTION ( 'NONE',  ( 0.000000000000000000, 0.000000000000000000, 1.000000000000000000 ) ) ;
#17137=ORIENTED_EDGE ( 'NONE', *, *, #24193, .T. ) ;
#17139=CARTESIAN_POINT ( 'NONE',  ( 31.14492845593375847, 6.928203230275506996, 165.9570628591036439 ) ) ;
#17144=CARTESIAN_POINT ( 'NONE',  ( 27.59788244552635206, -5.407089921784859143, 161.2326053007238897 ) ) ;
#17145=CARTESIAN_POINT ( 'NONE',  ( 26.75643035624999655, 3.323476615752271712, -2.690624999385500260 ) ) ;
#17151=CARTESIAN_POINT ( 'NONE',  ( 26.99999999999999645, -3.464101615137751278, -6.056249998770946164 ) ) ;
#17152=CARTESIAN_POINT ( 'NONE',  ( 20.99999999999999645, 6.646953231504538984, -3.853124999385470595 ) ) ;
#17154=CARTESIAN_POINT ( 'NONE',  ( 20.00041297495057080, 5.668978411116884608, -10.14010147226209035 ) ) ;
#17161=CARTESIAN_POINT ( 'NONE',  ( 24.94224478302373527, 0.000000000000000000, 163.9023435342771506 ) ) ;
#17165=CARTESIAN_POINT ( 'NONE',  ( 23.87821517812500005, -4.985214923628404016, -4.603124999385476812 ) ) ;
#17170=CARTESIAN_POINT ( 'NONE',  ( 33.92107042726159705, -5.196152422706629359, 163.2673710542620427 ) ) ;
#17173=CARTESIAN_POINT ( 'NONE',  ( 21.00000000000016342, -4.000000000000002665, 50.00000000000000000 ) ) ;
#17175=CARTESIAN_POINT ( 'NONE',  ( 33.85854767620964623, -5.407089921784861808, 161.1554086157566985 ) ) ;
#17178=CARTESIAN_POINT ( 'NONE',  ( 15.00000000000000355, 7.347880794884112834E-16, -8.000000000000000000 ) ) ;
#17183=CARTESIAN_POINT ( 'NONE',  ( 14.99999999999936229, 3.464101615137384904, -3.581249998770946075 ) ) ;
#17187=CARTESIAN_POINT ( 'NONE',  ( 24.00000000000000000, -5.196152422706629359, -4.799999999999998934 ) ) ;
#17188=CARTESIAN_POINT ( 'NONE',  ( 37.17765843037913953, -3.464101615137540779, 166.0692025214268313 ) ) ;
#17189=CARTESIAN_POINT ( 'NONE',  ( 36.85732959234155004, 7.646167579472024665E-16, 159.6131789008408646 ) ) ;
#17191=CARTESIAN_POINT ( 'NONE',  ( 27.60072650153512441, 5.196152422706636465, 159.8677888857873768 ) ) ;
#17198=DIRECTION ( 'NONE',  ( 1.000000000000000000, 0.000000000000000000, 0.000000000000000000 ) ) ;
#17200=CARTESIAN_POINT ( 'NONE',  ( 33.73804336749152810, 5.196152422706631135, 161.1753621882693892 ) ) ;
#17202=CARTESIAN_POINT ( 'NONE',  ( 26.75643035624999655, 7.049594010296217766E-16, -9.478124999385496352 ) ) ;
#17206=CARTESIAN_POINT ( 'NONE',  ( 33.87162103762178589, 5.407089921784862696, 161.3048378204704534 ) ) ;
#17215=AXIS2_PLACEMENT_3D ( 'NONE', #16047, #4651, #19645 ) ;
#17220=CARTESIAN_POINT ( 'NONE',  ( 21.27583786793474019, 5.761682509828531806, -8.000000000000005329 ) ) ;
#17221=CARTESIAN_POINT ( 'NONE',  ( 28.32508817407707014, 5.407089921784862696, 169.5446048129269059 ) ) ;
#17222=CARTESIAN_POINT ( 'NONE',  ( 18.00000000000000000, 5.196152422706630247, -1.368749998770957266 ) ) ;
#17229=CARTESIAN_POINT ( 'NONE',  ( 20.99999999999999645, 0.000000000000000000, 50.00000000000000000 ) ) ;
#17230=ORIENTED_EDGE ( 'NONE', *, *, #8492, .T. ) ;
#17231=CARTESIAN_POINT ( 'NONE',  ( 37.05506418370028143, -3.604726614523235284, 161.8732956221364816 ) ) ;
#17232=CARTESIAN_POINT ( 'NONE',  ( 15.24356964375000167, -3.323476615752272600, -7.303124999385448568 ) ) ;
#17234=CARTESIAN_POINT ( 'NONE',  ( 25.14654753852813229, -3.604726614523244610, 169.0321829630285322 ) ) ;
#17235=CARTESIAN_POINT ( 'NONE',  ( 34.26424616422337266, -5.196152422706635576, 167.1898876767739353 ) ) ;
#17246=EDGE_CURVE ( 'NONE', #17383, #35216, #23551, .T. ) ;
#17247=CARTESIAN_POINT ( 'NONE',  ( 15.24356964374999990, 3.323476615752268604, -1.190624999385493377 ) ) ;
#17255=CARTESIAN_POINT ( 'NONE',  ( 26.99999999999999289, 0.000000000000000000, -8.000000000000000000 ) ) ;
#17262=ADVANCED_FACE ( 'NONE', ( #927, #6620 ), #12110, .T. ) ;
#17264=DIRECTION ( 'NONE',  ( 0.9961946980917462113, 0.000000000000000000, -0.08715574274765118534 ) ) ;
#17268=( BOUNDED_CURVE ( )  B_SPLINE_CURVE ( 2, ( #31358, #5383, #16963, #22657, #34203, #2914, #14303 ),
 .UNSPECIFIED., .F., .F. ) 
 B_SPLINE_CURVE_WITH_KNOTS ( ( 3, 2, 2, 3 ),
 ( 0.6086956521739130821, 0.6159420289855073172, 0.6231884057971016633, 0.6304347826086960094 ),
 .UNSPECIFIED. ) 
 CURVE ( )  GEOMETRIC_REPRESENTATION_ITEM ( )  RATIONAL_B_SPLINE_CURVE ( ( 1.000000000000000000, 0.8660254037844387076, 1.000000000000000000, 0.8660254037844387076, 1.000000000000000000, 0.8660254037844326014, 1.000000000000006217 ) ) 
 REPRESENTATION_ITEM ( '' )  );
#17271=CARTESIAN_POINT ( 'NONE',  ( 28.26462387754589045, -5.407089921784859143, 168.8534947411257576 ) ) ;
#17280=ORIENTED_EDGE ( 'NONE', *, *, #17592, .T. ) ;
#17281=ORIENTED_EDGE ( 'NONE', *, *, #3854, .F. ) ;
#17285=CARTESIAN_POINT ( 'NONE',  ( 15.24356964374999990, 3.323476615752268604, -9.740624999385508076 ) ) ;
#17292=CARTESIAN_POINT ( 'NONE',  ( 28.10284103007056089, -5.407089921784865361, 167.0043083327929878 ) ) ;
#17299=CARTESIAN_POINT ( 'NONE',  ( 25.10569328411516921, 3.604726614523236616, 168.5652166982980305 ) ) ;
#17315=DIRECTION ( 'NONE',  ( 0.9961946980917462113, 0.000000000000000000, -0.08715574274765118534 ) ) ;
#17316=AXIS2_PLACEMENT_3D ( 'NONE', #30368, #7621, #27523 ) ;
#17327=CARTESIAN_POINT ( 'NONE',  ( 36.90145218710753738, 7.646167579472015790E-16, 160.1175024667497837 ) ) ;
#17328=CARTESIAN_POINT ( 'NONE',  ( 15.24356964374999990, 0.000000000000000000, -1.603124999385474592 ) ) ;
#17334=CARTESIAN_POINT ( 'NONE',  ( 26.99999999999999645, 3.464101615137755275, -6.431249998770947940 ) ) ;
#17335=CARTESIAN_POINT ( 'NONE',  ( 23.87821517812500005, -4.985214923628404016, -2.240624999385460114 ) ) ;
#17345=CARTESIAN_POINT ( 'NONE',  ( 24.82785287066744573, -3.464101615137757051, 162.5948379930317458 ) ) ;
#17350=CARTESIAN_POINT ( 'NONE',  ( 23.87821517812499650, 4.985214923628404904, -4.903124999385472194 ) ) ;
#17354=VERTEX_POINT ( 'NONE', #32392 ) ;
#17358=DIRECTION ( 'NONE',  ( 0.000000000000000000, 0.000000000000000000, 1.000000000000000000 ) ) ;
#17359=CARTESIAN_POINT ( 'NONE',  ( 24.51248951003896437, 3.604726614523240613, 161.7848665344110657 ) ) ;
#17372=VERTEX_POINT ( 'NONE', #3589 ) ;
#17373=CARTESIAN_POINT ( 'NONE',  ( 18.00000000000000355, -5.196152422706632912, -4.425000000000012257 ) ) ;
#17375=CARTESIAN_POINT ( 'NONE',  ( 24.36214585379926234, -3.604726614523244610, 160.0664306802028136 ) ) ;
#17377=CARTESIAN_POINT ( 'NONE',  ( 25.22335353682449721, 3.604726614523236616, 169.9100795407218811 ) ) ;
#17381=( BOUNDED_CURVE ( )  B_SPLINE_CURVE ( 2, ( #24238, #7185, #35784, #3385, #14954, #26502, #9267 ),
 .UNSPECIFIED., .F., .F. ) 
 B_SPLINE_CURVE_WITH_KNOTS ( ( 3, 2, 2, 3 ),
 ( 0.5217391304347817060, 0.5289855072463759411, 0.5362318840579700652, 0.5434782608695641892 ),
 .UNSPECIFIED. ) 
 CURVE ( )  GEOMETRIC_REPRESENTATION_ITEM ( )  RATIONAL_B_SPLINE_CURVE ( ( 1.000000000000016431, 0.8660254037844222763, 1.000000000000000000, 0.8660254037844387076, 1.000000000000000000, 0.8660254037844571373, 0.9999999999999815703 ) ) 
 REPRESENTATION_ITEM ( '' )  );
#17383=VERTEX_POINT ( 'NONE', #27091 ) ;
#17385=CARTESIAN_POINT ( 'NONE',  ( 24.99999999999998934, -2.343145750507539926, 49.65004534589634488 ) ) ;
#17388=CARTESIAN_POINT ( 'NONE',  ( 23.87821517812499650, 4.985214923628404904, -5.240624999385462779 ) ) ;
#17390=EDGE_CURVE ( 'NONE', #35535, #12708, #1116, .T. ) ;
#17396=CARTESIAN_POINT ( 'NONE',  ( 25.37366570962461054, 0.000000000000000000, 168.8335072898312887 ) ) ;
#17400=CYLINDRICAL_SURFACE ( 'NONE', #1574, 6.000000000000001776 ) ;
#17406=CARTESIAN_POINT ( 'NONE',  ( 25.90932369323456541, 3.028670999275696829, -8.000000000000000000 ) ) ;
#17407=CARTESIAN_POINT ( 'NONE',  ( 33.74578993402985816, -5.407089921784855591, 159.8665817251004739 ) ) ;
#17408=CARTESIAN_POINT ( 'NONE',  ( 26.99999999999999645, 7.347880794884117764E-16, -3.318749998770964549 ) ) ;
#17418=CARTESIAN_POINT ( 'NONE',  ( 30.75027635825099281, -7.209453229046475009, 161.4461687411947821 ) ) ;
#17419=CARTESIAN_POINT ( 'NONE',  ( 21.00000000000000000, -6.646953231504538984, -8.128124999385477167 ) ) ;
#17421=CARTESIAN_POINT ( 'NONE',  ( 28.24664800560418243, 5.407089921784862696, 168.6480295846443482 ) ) ;
#17422=CARTESIAN_POINT ( 'NONE',  ( 37.17765843037876294, -3.464101615137755275, 166.0692025214268597 ) ) ;
#17429=VERTEX_POINT ( 'NONE', #35416 ) ;
#17433=CARTESIAN_POINT ( 'NONE',  ( 21.00000000000000000, 6.646953231504538984, -3.965624999385493510 ) ) ;
#17441=CARTESIAN_POINT ( 'NONE',  ( 30.88999790839687876, -6.928203230275506996, 163.0431933671852676 ) ) ;
#17453=EDGE_CURVE ( 'NONE', #11581, #4178, #9467, .T. ) ;
#17454=CARTESIAN_POINT ( 'NONE',  ( 37.34761212884377812, 7.347880794884117764E-16, 168.0117821839301087 ) ) ;
#17457=CARTESIAN_POINT ( 'NONE',  ( 25.11222996482124259, -3.604726614523240613, 168.6399313006548937 ) ) ;
#17459=CYLINDRICAL_SURFACE ( 'NONE', #7300, 4.000000000000000888 ) ;
#17461=FACE_OUTER_BOUND ( 'NONE', #27391, .T. ) ;
#17463=CARTESIAN_POINT ( 'NONE',  ( 33.96029051149804445, -5.196152422706629359, 163.7156586684033073 ) ) ;
#17464=CARTESIAN_POINT ( 'NONE',  ( 37.22014685496823461, 7.347880794884125653E-16, 166.5548474367465985 ) ) ;
#17473=CARTESIAN_POINT ( 'NONE',  ( 21.00000000000000000, 6.646953231504538984, -9.815624999385470062 ) ) ;
#17476=ADVANCED_FACE ( 'NONE', ( #28926 ), #8844, .T. ) ;
#17480=CARTESIAN_POINT ( 'NONE',  ( 34.32918868704696536, -5.407089921784861808, 166.5348599854521296 ) ) ;
#17487=CARTESIAN_POINT ( 'NONE',  ( 37.52897353489062482, 7.646167579472015790E-16, 167.2901042930103586 ) ) ;
#17498=EDGE_CURVE ( 'NONE', #21163, #29577, #21900, .T. ) ;
#17500=CARTESIAN_POINT ( 'NONE',  ( 20.99999999999999645, 0.000000000000000000, -8.000000000000000000 ) ) ;
#17511=ORIENTED_EDGE ( 'NONE', *, *, #27441, .T. ) ;
#17515=CARTESIAN_POINT ( 'NONE',  ( 30.59339602130522096, -7.209453229046475009, 159.6530182846296384 ) ) ;
#17516=CARTESIAN_POINT ( 'NONE',  ( 18.12178482187499640, 4.985214923628404904, -2.578124999385478233 ) ) ;
#17519=ORIENTED_EDGE ( 'NONE', *, *, #7007, .F. ) ;
#17522=CARTESIAN_POINT ( 'NONE',  ( 18.12178482187499640, 4.985214923628404904, -4.715624999385465088 ) ) ;
#17525=EDGE_CURVE ( 'NONE', #6022, #25349, #22126, .T. ) ;
#17531=CARTESIAN_POINT ( 'NONE',  ( 36.87370277765342763, -3.464101615137751278, 162.5949735130562317 ) ) ;
#17536=CARTESIAN_POINT ( 'NONE',  ( 26.75643035624999655, -3.323476615752267271, -3.215624999385489957 ) ) ;
#17537=CARTESIAN_POINT ( 'NONE',  ( 15.00000000000000000, 0.000000000000000000, -0.4500000000000059508 ) ) ;
#17544=DIRECTION ( 'NONE',  ( 0.000000000000000000, 0.000000000000000000, 1.000000000000000000 ) ) ;
#17545=CARTESIAN_POINT ( 'NONE',  ( 30.90225418466721408, -7.209453229046482114, 163.1832832459922713 ) ) ;
#17548=EDGE_CURVE ( 'NONE', #29003, #26829, #3148, .T. ) ;
#17555=CARTESIAN_POINT ( 'NONE',  ( 15.00000000000058620, 3.464101615138089674, -7.631249998770955223 ) ) ;
#17560=CARTESIAN_POINT ( 'NONE',  ( 21.00000000000000000, -6.928203230275506996, -5.737500000000017586 ) ) ;
#17561=CARTESIAN_POINT ( 'NONE',  ( 21.00000000000000355, 0.000000000000000000, 50.00000000000001421 ) ) ;
#17564=CARTESIAN_POINT ( 'NONE',  ( 34.29487111334006499, -5.407089921784855591, 166.1426083230784911 ) ) ;
#17574=CARTESIAN_POINT ( 'NONE',  ( 21.00000000000000000, 6.646953231504538984, -7.453124999385469351 ) ) ;
#17581=CARTESIAN_POINT ( 'NONE',  ( 24.39482925732963281, 3.604726614523240613, 160.4400036919872150 ) ) ;
#17590=EDGE_CURVE ( 'NONE', #3817, #10799, #19699, .T. ) ;
#17591=ORIENTED_EDGE ( 'NONE', *, *, #34228, .F. ) ;
#17592=EDGE_CURVE ( 'NONE', #7912, #28136, #25763, .T. ) ;
#17595=CARTESIAN_POINT ( 'NONE',  ( 23.77150201299510712, 5.059023344826917068, -8.000000000000028422 ) ) ;
#17596=CARTESIAN_POINT ( 'NONE',  ( 28.41593846164884241, 5.957544813848095089, 159.6438083957854133 ) ) ;
#17597=CARTESIAN_POINT ( 'NONE',  ( 18.00000000000000000, 5.196152422706630247, -2.268749998770941190 ) ) ;
#17603=EDGE_CURVE ( 'NONE', #33644, #1610, #20601, .T. ) ;
#17604=( BOUNDED_CURVE ( )  B_SPLINE_CURVE ( 2, ( #21996, #21808, #33361, #10421, #7397, #4730, #16305 ),
 .UNSPECIFIED., .F., .F. ) 
 B_SPLINE_CURVE_WITH_KNOTS ( ( 3, 2, 2, 3 ),
 ( 0.8478260869565201752, 0.8550724637681145213, 0.8623188405797089784, 0.8695652173913032135 ),
 .UNSPECIFIED. ) 
 CURVE ( )  GEOMETRIC_REPRESENTATION_ITEM ( )  RATIONAL_B_SPLINE_CURVE ( ( 1.000000000000028644, 0.8660254037844099528, 1.000000000000000000, 0.8660254037844387076, 1.000000000000000000, 0.8660254037844592467, 0.9999999999999794609 ) ) 
 REPRESENTATION_ITEM ( '' )  );
#17607=CARTESIAN_POINT ( 'NONE',  ( 15.00000000000000000, 0.000000000000000000, -1.349999999999990097 ) ) ;
#17609=CARTESIAN_POINT ( 'NONE',  ( 24.67754069786733240, 0.000000000000000000, 163.6714102439223097 ) ) ;
#17610=CARTESIAN_POINT ( 'NONE',  ( 26.75643035624999655, 3.323476615752271712, -8.428124999385486760 ) ) ;
#17612=CARTESIAN_POINT ( 'NONE',  ( 34.13308826586474254, -5.407089921784861808, 164.2934219147456929 ) ) ;
#17613=CARTESIAN_POINT ( 'NONE',  ( 25.08932009880328096, 0.000000000000000000, 165.5834220860826349 ) ) ;
#17619=VECTOR ( 'NONE', #9839, 1000.000000000000000 ) ;
#17625=CARTESIAN_POINT ( 'NONE',  ( 18.12178482187499640, 4.985214923628404904, -5.278124999385486404 ) ) ;
#17636=CARTESIAN_POINT ( 'NONE',  ( 21.00000000000000355, 0.000000000000000000, 50.00000000000001421 ) ) ;
#17650=FACE_OUTER_BOUND ( 'NONE', #15010, .T. ) ;
#17656=LINE ( 'NONE', #35070, #5472 ) ;
#17662=CARTESIAN_POINT ( 'NONE',  ( 15.24356964374999990, 3.323476615752268604, -8.390624999385488891 ) ) ;
#17665=ORIENTED_EDGE ( 'NONE', *, *, #17590, .F. ) ;
#17669=CARTESIAN_POINT ( 'NONE',  ( 37.40314243129871841, -3.604726614523238837, 165.8518481976404360 ) ) ;
#17675=CARTESIAN_POINT ( 'NONE',  ( 25.22662187717753568, 0.000000000000000000, 169.9474368419002985 ) ) ;
#17676=VERTEX_POINT ( 'NONE', #5803 ) ;
#17691=CARTESIAN_POINT ( 'NONE',  ( 25.25600545691528254, 0.000000000000000000, 167.4886444474074381 ) ) ;
#17692=CARTESIAN_POINT ( 'NONE',  ( 28.32956640036948315, -5.196152422706632912, 168.1984670498039236 ) ) ;
#17701=CARTESIAN_POINT ( 'NONE',  ( 21.00000000000000000, 6.646953231504538984, -2.165624999385510563 ) ) ;
#17704=ORIENTED_EDGE ( 'NONE', *, *, #7983, .F. ) ;
#17706=CARTESIAN_POINT ( 'NONE',  ( 26.75643035624999655, 3.323476615752271268, -6.178124999385475213 ) ) ;
#17715=CARTESIAN_POINT ( 'NONE',  ( 33.84263025878871645, -5.196152422706629359, 162.3707958259794566 ) ) ;
#17719=CARTESIAN_POINT ( 'NONE',  ( 20.99999999999999645, -6.646953231504538984, -4.190624999385508254 ) ) ;
#17728=CARTESIAN_POINT ( 'NONE',  ( 36.85406125198851157, -3.604726614523238837, 159.5758215996624187 ) ) ;
#17733=DIRECTION ( 'NONE',  ( 0.000000000000000000, 0.000000000000000000, 1.000000000000000000 ) ) ;
#17742=ORIENTED_EDGE ( 'NONE', *, *, #9927, .T. ) ;
#17743=CARTESIAN_POINT ( 'NONE',  ( 24.00000000000000000, -5.196152422706629359, -7.950000000000012612 ) ) ;
#17745=CARTESIAN_POINT ( 'NONE',  ( 20.99999999999999645, 0.000000000000000000, -8.000000000000000000 ) ) ;
#17747=CARTESIAN_POINT ( 'NONE',  ( 31.26013745332475224, -7.209453229046475009, 167.2739077250314779 ) ) ;
#17752=ORIENTED_EDGE ( 'NONE', *, *, #16103, .F. ) ;
#17753=CARTESIAN_POINT ( 'NONE',  ( 26.97716818855048260, 0.000000000000000000, 49.47706554351410801 ) ) ;
#17754=CARTESIAN_POINT ( 'NONE',  ( 27.58438479987706415, -5.196152422706632912, 159.6810023811194981 ) ) ;
#17757=CARTESIAN_POINT ( 'NONE',  ( 21.00000000000000000, -6.646953231504538984, -5.428124999385471661 ) ) ;
#17763=CARTESIAN_POINT ( 'NONE',  ( 26.99999999999983658, 3.464101615137847645, -6.431249998770946164 ) ) ;
#17764=CARTESIAN_POINT ( 'NONE',  ( 36.81810950810510974, 7.646167579472024665E-16, 159.1648912866995715 ) ) ;
#17777=CARTESIAN_POINT ( 'NONE',  ( 31.15718473220409379, 7.209453229046482114, 166.0971527379105908 ) ) ;
#17778=CARTESIAN_POINT ( 'NONE',  ( 26.99999999999999645, -3.464101615137751278, -2.906249998770944032 ) ) ;
#17785=AXIS2_PLACEMENT_3D ( 'NONE', #17229, #35388, #31800 ) ;
#17787=CARTESIAN_POINT ( 'NONE',  ( 36.63511393177383013, 3.464101615138219348, 159.8678905258058194 ) ) ;
#17789=ORIENTED_EDGE ( 'NONE', *, *, #28427, .T. ) ;
#17791=CARTESIAN_POINT ( 'NONE',  ( 15.00000000000000000, 3.464101615137752166, -0.03749999999999697325 ) ) ;
#17792=CARTESIAN_POINT ( 'NONE',  ( 34.19887935716262461, 5.196152422706637353, 166.4427416532051609 ) ) ;
#17793=CARTESIAN_POINT ( 'NONE',  ( 37.40641077165175687, 7.646167579472024665E-16, 165.8892054988188534 ) ) ;
#17794=CARTESIAN_POINT ( 'NONE',  ( 36.90638618107669799, 7.347880794884125653E-16, 162.9685465236163111 ) ) ;
#17802=VERTEX_POINT ( 'NONE', #7313 ) ;
#17807=CARTESIAN_POINT ( 'NONE',  ( 26.75643035624999655, -3.323476615752267715, -4.115624999385481431 ) ) ;
#17830=CARTESIAN_POINT ( 'NONE',  ( 26.99999999999958078, -3.464101615137992862, -0.7125000000000120126 ) ) ;
#17839=CARTESIAN_POINT ( 'NONE',  ( 24.90959286293295705, 3.604726614523236616, 166.3237786275915937 ) ) ;
#17841=CARTESIAN_POINT ( 'NONE',  ( 21.00000000000000000, 6.646953231504538984, -1.603124999385459937 ) ) ;
#17851=CARTESIAN_POINT ( 'NONE',  ( 18.12178482187500350, -4.985214923628407568, -9.628124999385478944 ) ) ;
#17853=CARTESIAN_POINT ( 'NONE',  ( 37.37702719191401002, 7.347880794884125653E-16, 168.3479978933117422 ) ) ;
#17857=CARTESIAN_POINT ( 'NONE',  ( 31.13757469008587719, -7.209453229046482114, 165.8730089308399442 ) ) ;
#17858=ADVANCED_FACE ( 'NONE', ( #35730 ), #32893, .T. ) ;
#17864=CARTESIAN_POINT ( 'NONE',  ( 28.02930337212723089, -5.407089921784859143, 166.1637690562780278 ) ) ;
#17865=ORIENTED_EDGE ( 'NONE', *, *, #29381, .F. ) ;
#17880=LINE ( 'NONE', #32265, #37006 ) ;
#17881=FACE_OUTER_BOUND ( 'NONE', #14113, .T. ) ;
#17884=DIRECTION ( 'NONE',  ( 0.000000000000000000, 0.000000000000000000, 1.000000000000000000 ) ) ;
#17885=ORIENTED_EDGE ( 'NONE', *, *, #36247, .F. ) ;
#17890=CARTESIAN_POINT ( 'NONE',  ( 33.70656984979341786, -5.407089921784855591, 159.4182941109592093 ) ) ;
#17891=CARTESIAN_POINT ( 'NONE',  ( 26.75643035624999655, -3.323476615752267715, -1.415624999385507232 ) ) ;
#17897=CARTESIAN_POINT ( 'NONE',  ( 23.87821517812500005, -4.985214923628404016, -5.840624999385479299 ) ) ;
#17905=CARTESIAN_POINT ( 'NONE',  ( 30.79194769780577445, 6.928203230275506996, 161.9224743318320634 ) ) ;
#17909=CARTESIAN_POINT ( 'NONE',  ( 23.87821517812499650, 4.985214923628404904, -7.153124999385473970 ) ) ;
#17918=CARTESIAN_POINT ( 'NONE',  ( 33.78010750773675852, -5.407089921784861808, 160.2588333874741124 ) ) ;
#17922=CARTESIAN_POINT ( 'NONE',  ( 15.00000000000017408, -3.464101615137856083, -2.156249998770938703 ) ) ;
#17924=EDGE_CURVE ( 'NONE', #12908, #21187, #11479, .T. ) ;
#17931=CARTESIAN_POINT ( 'NONE',  ( 23.99999999999999645, 5.196152422706631135, -6.000000000000005329 ) ) ;
#17933=CYLINDRICAL_SURFACE ( 'NONE', #31637, 5.999999999999994671 ) ;
#17935=CARTESIAN_POINT ( 'NONE',  ( 34.38638464322509947, 5.407089921784857367, 167.1886127560748321 ) ) ;
#17937=CARTESIAN_POINT ( 'NONE',  ( 27.64975160693779443, 5.196152422706630247, 160.4281484046883293 ) ) ;
#17939=ORIENTED_EDGE ( 'NONE', *, *, #14057, .T. ) ;
#17940=EDGE_LOOP ( 'NONE', ( #11449, #32754, #36567, #2219 ) ) ;
#17941=CARTESIAN_POINT ( 'NONE',  ( 24.97165984609394940, 0.000000000000000000, 164.2385592436587558 ) ) ;
#17944=CARTESIAN_POINT ( 'NONE',  ( 33.75438506914960612, -5.196152422706635576, 161.3621486929372111 ) ) ;
#17945=CARTESIAN_POINT ( 'NONE',  ( 15.24356964375000167, -3.323476615752272600, -6.853124999385484806 ) ) ;
#17948=CARTESIAN_POINT ( 'NONE',  ( 24.82458453031440726, 0.000000000000000000, 162.5574806918533000 ) ) ;
#17950=VECTOR ( 'NONE', #13304, 1000.000000000000000 ) ;
#17954=CARTESIAN_POINT ( 'NONE',  ( 27.54068648934820729, 5.407089921784862696, 160.5788525301012157 ) ) ;
#17968=CARTESIAN_POINT ( 'NONE',  ( 24.98966720158236043, -3.604726614523244610, 167.2390325064633885 ) ) ;
#17969=CARTESIAN_POINT ( 'NONE',  ( 21.00000000000000000, -6.928203230275506996, -3.431249998770965703 ) ) ;
#17973=LINE ( 'NONE', #29516, #22518 ) ;
#17974=DIRECTION ( 'NONE',  ( 0.000000000000000000, 0.000000000000000000, 1.000000000000000000 ) ) ;
#17976=CARTESIAN_POINT ( 'NONE',  ( 26.99999999999999645, 7.347880794884117764E-16, -0.2250000000000029754 ) ) ;
#17979=CARTESIAN_POINT ( 'NONE',  ( 27.50636891564131759, 5.407089921784856479, 160.1866008677275772 ) ) ;
#17980=CARTESIAN_POINT ( 'NONE',  ( 15.24356964375000167, -3.323476615752272600, -10.00312499938545407 ) ) ;
#17983=CARTESIAN_POINT ( 'NONE',  ( 37.21357869082257253, 3.604726614523243278, 163.6851247292908624 ) ) ;
#17985=CARTESIAN_POINT ( 'NONE',  ( 36.87043443719328195, 3.464101615137759271, 162.5576162106534639 ) ) ;
#17986=CARTESIAN_POINT ( 'NONE',  ( 15.00000000000000000, 0.000000000000000000, -7.143749998770959841 ) ) ;
#17991=VERTEX_POINT ( 'NONE', #24557 ) ;
#17997=CARTESIAN_POINT ( 'NONE',  ( 23.87821517812500005, -4.985214923628404016, -3.253124999385486937 ) ) ;
#18011=CARTESIAN_POINT ( 'NONE',  ( 37.13350435217316203, -3.604726614523235284, 162.7698708504190677 ) ) ;
#18014=DIRECTION ( 'NONE',  ( 0.000000000000000000, -1.000000000000000000, 0.000000000000000000 ) ) ;
#18018=CARTESIAN_POINT ( 'NONE',  ( 15.00000000000000000, 0.000000000000000000, -2.193749998770949894 ) ) ;
#18023=CARTESIAN_POINT ( 'NONE',  ( 24.99456971211191103, -3.604726614523240613, 167.2950684582310146 ) ) ;
#18024=CARTESIAN_POINT ( 'NONE',  ( 18.12178482187499640, 4.985214923628404904, -2.465624999385462868 ) ) ;
#18027=( BOUNDED_CURVE ( )  B_SPLINE_CURVE ( 2, ( #2644, #14220, #9280, #14966, #24064, #3960, #32958 ),
 .UNSPECIFIED., .F., .F. ) 
 B_SPLINE_CURVE_WITH_KNOTS ( ( 3, 2, 2, 3 ),
 ( 0.2826086956521750015, 0.2898550724637684040, 0.2971014492753618064, 0.3043478260869552088 ),
 .UNSPECIFIED. ) 
 CURVE ( )  GEOMETRIC_REPRESENTATION_ITEM ( )  RATIONAL_B_SPLINE_CURVE ( ( 0.9999999999999794609, 0.8660254037844592467, 1.000000000000000000, 0.8660254037844387076, 1.000000000000000000, 0.8660254037844633546, 0.9999999999999753530 ) ) 
 REPRESENTATION_ITEM ( '' )  );
#18030=CARTESIAN_POINT ( 'NONE',  ( 28.08444087378459741, -5.196152422706638241, 165.3966694601965060 ) ) ;
#18033=CARTESIAN_POINT ( 'NONE',  ( 31.15473347688575956, -6.928203230275514990, 166.0691347614145741 ) ) ;
#18037=CARTESIAN_POINT ( 'NONE',  ( 21.00000000000000000, 6.646953231504538984, -0.7031249993854685743 ) ) ;
#18039=CARTESIAN_POINT ( 'NONE',  ( 24.00000000000000000, -5.196152422706629359, -6.093749998770964460 ) ) ;
#18046=CARTESIAN_POINT ( 'NONE',  ( 27.97210741594907901, 5.407089921784862696, 165.5100162856553538 ) ) ;
#18049=AXIS2_PLACEMENT_3D ( 'NONE', #6308, #9153, #20536 ) ;
#18054=CARTESIAN_POINT ( 'NONE',  ( 28.10774354060011504, -5.407089921784859143, 167.0603442845606139 ) ) ;
#18073=CARTESIAN_POINT ( 'NONE',  ( 15.93765667431398825, -3.220065975715824536, -8.000000000000000000 ) ) ;
#18074=CYLINDRICAL_SURFACE ( 'NONE', #29645, 5.999999999999994671 ) ;
#18076=LINE ( 'NONE', #35487, #9386 ) ;
#18083=CARTESIAN_POINT ( 'NONE',  ( 18.12178482187500350, -4.985214923628407568, -5.578124999385480898 ) ) ;
#18088=CARTESIAN_POINT ( 'NONE',  ( 15.24356964375000167, -3.323476615752272600, -5.953124999385460470 ) ) ;
#18090=( BOUNDED_CURVE ( )  B_SPLINE_CURVE ( 2, ( #30975, #4251, #27752, #27375, #30607, #21886, #4992 ),
 .UNSPECIFIED., .F., .F. ) 
 B_SPLINE_CURVE_WITH_KNOTS ( ( 3, 2, 2, 3 ),
 ( 0.6739130434782595325, 0.6811594202898538786, 0.6884057971014482247, 0.6956521739130425708 ),
 .UNSPECIFIED. ) 
 CURVE ( )  GEOMETRIC_REPRESENTATION_ITEM ( )  RATIONAL_B_SPLINE_CURVE ( ( 1.000000000000024647, 0.8660254037844140607, 1.000000000000000000, 0.8660254037844387076, 1.000000000000000000, 0.8660254037844551389, 0.9999999999999835687 ) ) 
 REPRESENTATION_ITEM ( '' )  );
#18097=CARTESIAN_POINT ( 'NONE',  ( 27.84585202812001015, 5.196152422706630247, 162.6695864753947660 ) ) ;
#18101=CARTESIAN_POINT ( 'NONE',  ( 20.99999999999999645, -6.646953231504538984, -5.990624999385490312 ) ) ;
#18108=CARTESIAN_POINT ( 'NONE',  ( 15.00000000000000000, 0.000000000000000000, -6.693749998770953447 ) ) ;
#18121=CARTESIAN_POINT ( 'NONE',  ( 26.99999999999999645, -3.464101615137751278, -6.562499999999983125 ) ) ;
#18122=CARTESIAN_POINT ( 'NONE',  ( 20.99999999999999645, 6.928203230275506996, -3.262499999999992628 ) ) ;
#18125=CARTESIAN_POINT ( 'NONE',  ( 31.22091736908830839, -7.209453229046475009, 166.8256201108902133 ) ) ;
#18127=CARTESIAN_POINT ( 'NONE',  ( 24.66443585301628616, 3.464101615138150514, 160.7269729341096536 ) ) ;
#18130=ORIENTED_EDGE ( 'NONE', *, *, #9448, .F. ) ;
#18134=CARTESIAN_POINT ( 'NONE',  ( 15.00000000000000000, 0.000000000000000000, -3.543749998770939769 ) ) ;
#18136=CARTESIAN_POINT ( 'NONE',  ( 18.12178482187500350, -4.985214923628407568, -7.265624999385461358 ) ) ;
#18143=CARTESIAN_POINT ( 'NONE',  ( 28.41103801510778837, 5.957546011302761180, 159.5877722384327342 ) ) ;
#18155=CARTESIAN_POINT ( 'NONE',  ( 26.99999999999999645, 7.347880794884117764E-16, -7.874999999999992895 ) ) ;
#18156=CARTESIAN_POINT ( 'NONE',  ( 37.41297893579764633, -3.464101615137622936, 168.7589282062745610 ) ) ;
#18157=CARTESIAN_POINT ( 'NONE',  ( 34.44684893975629336, -5.407089921784861808, 167.8797228278759803 ) ) ;
#18168=CARTESIAN_POINT ( 'NONE',  ( 36.85896376251805862, -3.604726614523235284, 159.6318575514300449 ) ) ;
#18169=CARTESIAN_POINT ( 'NONE',  ( 26.75643035624999655, 7.049594010296217766E-16, -8.915624999385475036 ) ) ;
#18171=CARTESIAN_POINT ( 'NONE',  ( 31.38024896135242159, 6.928203230275506996, 168.6467885439513452 ) ) ;
#18172=CARTESIAN_POINT ( 'NONE',  ( 34.21152843433763024, -5.407089921784861808, 165.1899971430282505 ) ) ;
#18173=CARTESIAN_POINT ( 'NONE',  ( 30.99785313993998415, -6.928203230275514990, 164.2759843048494872 ) ) ;
#18174=CARTESIAN_POINT ( 'NONE',  ( 28.14980768084533125, 5.196152422706636465, 166.1438154837653656 ) ) ;
#18184=CARTESIAN_POINT ( 'NONE',  ( 26.75643035624999655, -3.323476615752267715, -5.015624999385472904 ) ) ;
#18191=EDGE_CURVE ( 'NONE', #22619, #23933, #596, .T. ) ;
#18196=AXIS2_PLACEMENT_3D ( 'NONE', #9411, #28741, #14354 ) ;
#18201=CARTESIAN_POINT ( 'NONE',  ( 24.75924920669326212, -3.604726614523240613, 164.6053427733833132 ) ) ;
#18204=CARTESIAN_POINT ( 'NONE',  ( 18.00000000000000355, -5.196152422706632912, -4.874999999999990230 ) ) ;
#18213=CARTESIAN_POINT ( 'NONE',  ( 24.98803303140584120, 3.604726614523236616, 167.2203538558741513 ) ) ;
#18214=CARTESIAN_POINT ( 'NONE',  ( 15.24356964374999990, 3.323476615752268604, -2.428124999385457894 ) ) ;
#18219=CARTESIAN_POINT ( 'NONE',  ( 20.99999999999999645, 6.928203230275506996, -3.206249998770952292 ) ) ;
#18223=ORIENTED_EDGE ( 'NONE', *, *, #1576, .F. ) ;
#18227=CARTESIAN_POINT ( 'NONE',  ( 15.24356964374999990, 0.000000000000000000, -1.490624999385459226 ) ) ;
#18229=CARTESIAN_POINT ( 'NONE',  ( 21.00000000000000000, 6.928203230275506996, -7.706249998770941190 ) ) ;
#18234=CARTESIAN_POINT ( 'NONE',  ( 34.10694154304044901, 5.407089921784862696, 163.9945635053181547 ) ) ;
#18237=( NAMED_UNIT ( * ) SI_UNIT ( $, .STERADIAN. ) SOLID_ANGLE_UNIT ( ) );
#18241=CARTESIAN_POINT ( 'NONE',  ( 37.36882485759181804, -3.604726614523235284, 165.4595965352667690 ) ) ;
#18242=ORIENTED_EDGE ( 'NONE', *, *, #6466, .T. ) ;
#18258=CARTESIAN_POINT ( 'NONE',  ( 17.00000000000002132, -2.343145750507694913, 50.17464377163449285 ) ) ;
#18268=CARTESIAN_POINT ( 'NONE',  ( 21.00000000000000000, 6.646953231504538984, -3.515624999385498217 ) ) ;
#18272=( BOUNDED_CURVE ( )  B_SPLINE_CURVE ( 2, ( #19506, #31052, #31232, #5074, #34259, #17763, #17019 ),
 .UNSPECIFIED., .F., .F. ) 
 B_SPLINE_CURVE_WITH_KNOTS ( ( 3, 2, 2, 3 ),
 ( 0.5652173913043473386, 0.5724637681159415736, 0.5797101449275359197, 0.5869565217391301548 ),
 .UNSPECIFIED. ) 
 CURVE ( )  GEOMETRIC_REPRESENTATION_ITEM ( )  RATIONAL_B_SPLINE_CURVE ( ( 1.000000000000008216, 0.8660254037844304920, 1.000000000000000000, 0.8660254037844387076, 1.000000000000000000, 0.8660254037844448138, 0.9999999999999938938 ) ) 
 REPRESENTATION_ITEM ( '' )  );
#18274=CARTESIAN_POINT ( 'NONE',  ( 15.24356964375000167, -3.323476615752272600, -5.503124999385465621 ) ) ;
#18286=CARTESIAN_POINT ( 'NONE',  ( 15.24356964375000167, -3.323476615752272600, -6.515624999385480010 ) ) ;
#18287=CARTESIAN_POINT ( 'NONE',  ( 23.99999999999999645, 5.196152422706631135, -2.400000000000013234 ) ) ;
#18291=CARTESIAN_POINT ( 'NONE',  ( 36.83775103377001869, 7.347880794884117764E-16, 162.1840432000934129 ) ) ;
#18308=ORIENTED_EDGE ( 'NONE', *, *, #34950, .T. ) ;
#18309=CARTESIAN_POINT ( 'NONE',  ( 23.99999999999999645, 5.196152422706631135, -6.450000000000011724 ) ) ;
#18310=( BOUNDED_CURVE ( )  B_SPLINE_CURVE ( 2, ( #24906, #37016, #19802, #22818, #10686, #8410, #31161 ),
 .UNSPECIFIED., .F., .F. ) 
 B_SPLINE_CURVE_WITH_KNOTS ( ( 3, 2, 2, 3 ),
 ( 0.4782608695652184050, 0.4855072463768126956, 0.4927536231884070417, 0.5000000000000013323 ),
 .UNSPECIFIED. ) 
 CURVE ( )  GEOMETRIC_REPRESENTATION_ITEM ( )  RATIONAL_B_SPLINE_CURVE ( ( 0.9999999999999815703, 0.8660254037844571373, 1.000000000000000000, 0.8660254037844387076, 1.000000000000000000, 0.8660254037844140607, 1.000000000000024647 ) ) 
 REPRESENTATION_ITEM ( '' )  );
#18314=CARTESIAN_POINT ( 'NONE',  ( 31.20130732697009535, 7.209453229046475009, 166.6014763038195383 ) ) ;
#18323=CARTESIAN_POINT ( 'NONE',  ( 15.24356964375000167, -3.323476615752272600, -8.653124999385468641 ) ) ;
#18330=CARTESIAN_POINT ( 'NONE',  ( 25.29522554115172639, 0.000000000000000000, 167.9369320615487311 ) ) ;
#18341=VECTOR ( 'NONE', #36761, 1000.000000000000000 ) ;
#18343=CARTESIAN_POINT ( 'NONE',  ( 25.10405911393864642, 0.000000000000000000, 168.5465380477087933 ) ) ;
#18352=LINE ( 'NONE', #1085, #16684 ) ;
#18357=CARTESIAN_POINT ( 'NONE',  ( 26.75643035624999655, 3.323476615752271712, -9.328124999385446259 ) ) ;
#18359=CARTESIAN_POINT ( 'NONE',  ( 28.01132750018552287, 5.407089921784862696, 165.9583038997966185 ) ) ;
#18360=CARTESIAN_POINT ( 'NONE',  ( 30.93902301358532014, 6.928203230275514990, 163.6035528836375192 ) ) ;
#18369=DIRECTION ( 'NONE',  ( 0.08715574274765150453, 0.000000000000000000, 0.9961946980917461003 ) ) ;
#18371=CARTESIAN_POINT ( 'NONE',  ( 15.24356964374999990, 3.323476615752268604, -6.140624999385478233 ) ) ;
#18374=VECTOR ( 'NONE', #16378, 1000.000000000000000 ) ;
#18386=CARTESIAN_POINT ( 'NONE',  ( 34.15106413780644345, 5.407089921784857367, 164.4988870712271023 ) ) ;
#18399=CARTESIAN_POINT ( 'NONE',  ( 24.95208128752243226, 0.000000000000000000, 166.8094235429113041 ) ) ;
#18400=CARTESIAN_POINT ( 'NONE',  ( 21.00000000000000000, -6.646953231504538984, -1.828124999385473792 ) ) ;
#18402=CARTESIAN_POINT ( 'NONE',  ( 14.99999999999965539, 3.464101615137553658, -3.637499999999990852 ) ) ;
#18412=COLOUR_RGB ( '',0.8941176470588234615, 0.8941176470588234615, 0.8941176470588234615 ) ;
#18415=CARTESIAN_POINT ( 'NONE',  ( 26.75643035624999655, 3.323476615752271712, -0.7781249993854945091 ) ) ;
#18417=VECTOR ( 'NONE', #33867, 1000.000000000000000 ) ;
#18418=CARTESIAN_POINT ( 'NONE',  ( 26.99999999999999645, 3.464101615137755275, -10.03124999877094581 ) ) ;
#18420=DIRECTION ( 'NONE',  ( 1.000000000000000000, 0.000000000000000000, 0.000000000000000000 ) ) ;
#18421=ORIENTED_EDGE ( 'NONE', *, *, #29074, .F. ) ;
#18425=CARTESIAN_POINT ( 'NONE',  ( 27.90674060888834518, -5.407089921784865361, 164.7628702620865226 ) ) ;
#18434=CARTESIAN_POINT ( 'NONE',  ( 31.27974749544297595, 7.209453229046475009, 167.4980515321021244 ) ) ;
#18435=VERTEX_POINT ( 'NONE', #19559 ) ;
#18448=CARTESIAN_POINT ( 'NONE',  ( 21.00000000000000355, 0.000000000000000000, 50.00000000000001421 ) ) ;
#18454=CARTESIAN_POINT ( 'NONE',  ( 18.20792125986140064, 5.080248635121038525, -7.999999999999994671 ) ) ;
#18458=ORIENTED_EDGE ( 'NONE', *, *, #16987, .F. ) ;
#18464=CARTESIAN_POINT ( 'NONE',  ( 21.00000000000000000, 6.646953231504538984, -4.415624999385457272 ) ) ;
#18468=CARTESIAN_POINT ( 'NONE',  ( 20.99999999999999645, -6.646953231504538984, -7.678124999385482319 ) ) ;
#18475=CARTESIAN_POINT ( 'NONE',  ( 33.62038311478219299, 5.196152422706631135, 159.8304993458455385 ) ) ;
#18478=( BOUNDED_CURVE ( )  B_SPLINE_CURVE ( 2, ( #33603, #1189, #7643, #19219, #15427, #26976, #27166 ),
 .UNSPECIFIED., .F., .F. ) 
 B_SPLINE_CURVE_WITH_KNOTS ( ( 3, 2, 2, 3 ),
 ( 0.4565217391304338679, 0.4637681159420281585, 0.4710144927536223936, 0.4782608695652166841 ),
 .UNSPECIFIED. ) 
 CURVE ( )  GEOMETRIC_REPRESENTATION_ITEM ( )  RATIONAL_B_SPLINE_CURVE ( ( 1.000000000000016431, 0.8660254037844222763, 1.000000000000000000, 0.8660254037844387076, 1.000000000000000000, 0.8660254037844520303, 0.9999999999999866773 ) ) 
 REPRESENTATION_ITEM ( '' )  );
#18480=CARTESIAN_POINT ( 'NONE',  ( 26.75643035624999655, -3.323476615752267271, -5.915624999385464378 ) ) ;
#18488=CARTESIAN_POINT ( 'NONE',  ( 29.48995970988985604, 6.148715791637015649, 159.4803054849043633 ) ) ;
#18493=CARTESIAN_POINT ( 'NONE',  ( 15.00000000000000000, 0.000000000000000000, -1.799999999999996048 ) ) ;
#18497=( BOUNDED_CURVE ( )  B_SPLINE_CURVE ( 2, ( #8390, #22981, #28098, #8205, #5158, #19782, #25442 ),
 .UNSPECIFIED., .F., .F. ) 
 B_SPLINE_CURVE_WITH_KNOTS ( ( 3, 2, 2, 3 ),
 ( 0.8260869565217379140, 0.8333333333333329263, 0.8405797101449278275, 0.8478260869565228397 ),
 .UNSPECIFIED. ) 
 CURVE ( )  GEOMETRIC_REPRESENTATION_ITEM ( )  RATIONAL_B_SPLINE_CURVE ( ( 1.000000000000022649, 0.8660254037844161701, 1.000000000000000000, 0.8660254037844387076, 1.000000000000000000, 0.8660254037844181685, 1.000000000000020428 ) ) 
 REPRESENTATION_ITEM ( '' )  );
#18501=ORIENTED_EDGE ( 'NONE', *, *, #36268, .F. ) ;
#18502=CARTESIAN_POINT ( 'NONE',  ( 15.00000000000000000, 0.000000000000000000, -6.750000000000006217 ) ) ;
#18507=CARTESIAN_POINT ( 'NONE',  ( 31.08364707426076023, 7.209453229046475009, 165.2566134613956876 ) ) ;
#18510=VERTEX_POINT ( 'NONE', #25231 ) ;
#18515=CARTESIAN_POINT ( 'NONE',  ( 15.24356964374999990, 0.000000000000000000, -0.1406249993854691294 ) ) ;
#18516=CARTESIAN_POINT ( 'NONE',  ( 27.00000000000058620, -3.464101615137410661, -1.162499999999995204 ) ) ;
#18518=CARTESIAN_POINT ( 'NONE',  ( 15.24356964374999990, 0.000000000000000000, -9.590624999385454430 ) ) ;
#18524=AXIS2_PLACEMENT_3D ( 'NONE', #25607, #36977, #31300 ) ;
#18525=CYLINDRICAL_SURFACE ( 'NONE', #25257, 4.000000000000000888 ) ;
#18526=CARTESIAN_POINT ( 'NONE',  ( 25.25273711656224407, 3.464101615137752166, 167.4512871462289922 ) ) ;
#18537=CARTESIAN_POINT ( 'NONE',  ( 33.72497000607938844, -5.196152422706629359, 161.0259329835556059 ) ) ;
#18538=DIRECTION ( 'NONE',  ( 0.08715574274765150453, 0.000000000000000000, 0.9961946980917461003 ) ) ;
#18539=CARTESIAN_POINT ( 'NONE',  ( 34.34226204845910502, 5.407089921784862696, 166.6842891901658845 ) ) ;
#18545=ADVANCED_FACE ( 'NONE', ( #24670 ), #5130, .T. ) ;
#18554=CARTESIAN_POINT ( 'NONE',  ( 24.36051168362275021, 3.604726614523236616, 160.0477520296135765 ) ) ;
#18555=ORIENTED_EDGE ( 'NONE', *, *, #29307, .T. ) ;
#18556=CARTESIAN_POINT ( 'NONE',  ( 15.24356964374999990, 0.000000000000000000, -10.04062499938546082 ) ) ;
#18557=CARTESIAN_POINT ( 'NONE',  ( 24.63014976274829593, 3.604726614523240613, 163.1297293768349164 ) ) ;
#18558=CARTESIAN_POINT ( 'NONE',  ( 24.81477950914817754, 0.000000000000000000, 162.4454087870936121 ) ) ;
#18561=EDGE_CURVE ( 'NONE', #35079, #32003, #20903, .T. ) ;
#18562=AXIS2_PLACEMENT_3D ( 'NONE', #23093, #13822, #19519 ) ;
#18570=CARTESIAN_POINT ( 'NONE',  ( 23.87821517812499650, 4.985214923628404904, -5.803124999385484095 ) ) ;
#18573=VECTOR ( 'NONE', #14082, 1000.000000000000000 ) ;
#18582=CARTESIAN_POINT ( 'NONE',  ( 26.99999999999999645, 7.347880794884117764E-16, -2.925000000000010925 ) ) ;
#18583=CARTESIAN_POINT ( 'NONE',  ( 37.14004103287923186, 3.604726614523238837, 162.8445854527759309 ) ) ;
#18593=ORIENTED_EDGE ( 'NONE', *, *, #35785, .T. ) ;
#18594=CARTESIAN_POINT ( 'NONE',  ( 37.37209319794485651, 7.646167579472015790E-16, 165.4969538364452148 ) ) ;
#18595=CARTESIAN_POINT ( 'NONE',  ( 23.87821517812499650, 4.985214923628404904, -3.440624999385466509 ) ) ;
#18598=CARTESIAN_POINT ( 'NONE',  ( 34.00277893598041601, 5.196152422706637353, 164.2013035824986957 ) ) ;
#18609=CARTESIAN_POINT ( 'NONE',  ( 18.12178482187500350, -4.985214923628407568, -2.765624999385457805 ) ) ;
#18611=CARTESIAN_POINT ( 'NONE',  ( 18.12178482187499640, 4.985214923628404904, -0.3281249993854762348 ) ) ;
#18612=( BOUNDED_CURVE ( )  B_SPLINE_CURVE ( 2, ( #31667, #2852, #3981, #18219, #24458, #27112, #27294 ),
 .UNSPECIFIED., .F., .F. ) 
 B_SPLINE_CURVE_WITH_KNOTS ( ( 3, 2, 2, 3 ),
 ( 0.2608695652173921298, 0.2681159420289864759, 0.2753623188405807110, 0.2826086956521750015 ),
 .UNSPECIFIED. ) 
 CURVE ( )  GEOMETRIC_REPRESENTATION_ITEM ( )  RATIONAL_B_SPLINE_CURVE ( ( 0.9999999999999845679, 0.8660254037844541397, 1.000000000000000000, 0.8660254037844387076, 1.000000000000000000, 0.8660254037844181685, 1.000000000000020428 ) ) 
 REPRESENTATION_ITEM ( '' )  );
#18619=CARTESIAN_POINT ( 'NONE',  ( 34.01542801315541453, -5.407089921784861808, 162.9485590723218422 ) ) ;
#18624=FACE_OUTER_BOUND ( 'NONE', #13420, .T. ) ;
#18628=CARTESIAN_POINT ( 'NONE',  ( 34.29487111334006499, -5.407089921784855591, 166.1426083230784911 ) ) ;
#18640=CYLINDRICAL_SURFACE ( 'NONE', #3663, 6.000000000000001776 ) ;
#18643=CARTESIAN_POINT ( 'NONE',  ( 27.00000000000036593, -3.464101615137536783, -5.662499999999986322 ) ) ;
#18647=DIRECTION ( 'NONE',  ( 0.000000000000000000, 0.000000000000000000, 1.000000000000000000 ) ) ;
#18654=CARTESIAN_POINT ( 'NONE',  ( 23.87821517812499650, 4.985214923628404904, -3.553124999385481875 ) ) ;
#18669=CARTESIAN_POINT ( 'NONE',  ( 15.24356964374999990, 0.000000000000000000, -5.653124999385472194 ) ) ;
#18673=CARTESIAN_POINT ( 'NONE',  ( 22.12957385106072294, -6.276043463296034908, -7.973380326861742695 ) ) ;
#18686=CARTESIAN_POINT ( 'NONE',  ( 37.29858702344112231, 7.347880794884125653E-16, 167.4514226650291562 ) ) ;
#18696=CARTESIAN_POINT ( 'NONE',  ( 34.11184405356999605, 5.407089921784857367, 164.0505994570858093 ) ) ;
#18704=DIRECTION ( 'NONE',  ( 0.000000000000000000, 0.000000000000000000, 1.000000000000000000 ) ) ;
#18708=CARTESIAN_POINT ( 'NONE',  ( 26.75643035624999655, 3.323476615752271712, -8.428124999385486760 ) ) ;
#18711=( BOUNDED_CURVE ( )  B_SPLINE_CURVE ( 2, ( #1967, #13916, #13165, #25093, #19804, #24721, #10317 ),
 .UNSPECIFIED., .F., .F. ) 
 B_SPLINE_CURVE_WITH_KNOTS ( ( 3, 2, 2, 3 ),
 ( 0.3695652173913035465, 0.3768115942028978371, 0.3840579710144921277, 0.3913043478260864183 ),
 .UNSPECIFIED. ) 
 CURVE ( )  GEOMETRIC_REPRESENTATION_ITEM ( )  RATIONAL_B_SPLINE_CURVE ( ( 1.000000000000014433, 0.8660254037844243857, 1.000000000000000000, 0.8660254037844387076, 1.000000000000000000, 0.8660254037844489217, 0.9999999999999897859 ) ) 
 REPRESENTATION_ITEM ( '' )  );
#18716=CARTESIAN_POINT ( 'NONE',  ( 25.17756528844239483, 0.000000000000000000, 166.5920692191248804 ) ) ;
#18721=CARTESIAN_POINT ( 'NONE',  ( 30.78214267663954473, 6.928203230275514990, 161.8104024270723755 ) ) ;
#18729=CARTESIAN_POINT ( 'NONE',  ( 24.74781001545762393, 3.604726614523240613, 164.4745922192587670 ) ) ;
#18742=CARTESIAN_POINT ( 'NONE',  ( 24.00000000000000000, -5.196152422706629359, -6.093749998770964460 ) ) ;
#18744=CARTESIAN_POINT ( 'NONE',  ( 18.00000000000000000, 5.196152422706630247, -1.425000000000009592 ) ) ;
#18746=CARTESIAN_POINT ( 'NONE',  ( 27.82830044041545747, -5.407089921784865361, 163.8662950338039650 ) ) ;
#18747=CARTESIAN_POINT ( 'NONE',  ( 27.71838675424445597, 5.196152422706636465, 161.2126517282112275 ) ) ;
#18757=CARTESIAN_POINT ( 'NONE',  ( 15.24356964374999990, 3.323476615752268604, -7.040624999385501681 ) ) ;
#18768=( BOUNDED_CURVE ( )  B_SPLINE_CURVE ( 2, ( #27794, #36498, #30268, #10541, #27976, #22301, #25133 ),
 .UNSPECIFIED., .F., .F. ) 
 B_SPLINE_CURVE_WITH_KNOTS ( ( 3, 2, 2, 3 ),
 ( 0.6521739130434773823, 0.6594202898550715064, 0.6666666666666654084, 0.6739130434782595325 ),
 .UNSPECIFIED. ) 
 CURVE ( )  GEOMETRIC_REPRESENTATION_ITEM ( )  RATIONAL_B_SPLINE_CURVE ( ( 1.000000000000016431, 0.8660254037844222763, 1.000000000000000000, 0.8660254037844387076, 1.000000000000000000, 0.8660254037844633546, 0.9999999999999753530 ) ) 
 REPRESENTATION_ITEM ( '' )  );
#18769=EDGE_CURVE ( 'NONE', #407, #18510, #13149, .T. ) ;
#18772=ADVANCED_FACE ( 'NONE', ( #15731 ), #32591, .T. ) ;
#18774=CARTESIAN_POINT ( 'NONE',  ( 24.79846929092969887, -3.604726614523240613, 165.0536303875245778 ) ) ;
#18785=CARTESIAN_POINT ( 'NONE',  ( 37.32960477335537774, -3.604726614523235284, 165.0113089211254760 ) ) ;
#18786=CARTESIAN_POINT ( 'NONE',  ( 26.75643035624999655, 3.323476615752271712, -3.928124999385464999 ) ) ;
#18787=DIRECTION ( 'NONE',  ( 0.000000000000000000, 0.000000000000000000, 1.000000000000000000 ) ) ;
#18788=CARTESIAN_POINT ( 'NONE',  ( 34.35575969410840003, 5.196152422706637353, 168.2358921097703046 ) ) ;
#18796=ORIENTED_EDGE ( 'NONE', *, *, #35289, .F. ) ;
#18799=CARTESIAN_POINT ( 'NONE',  ( 23.87821517812500005, -4.985214923628404016, -0.8906249993854697955 ) ) ;
#18801=CARTESIAN_POINT ( 'NONE',  ( 26.99999999999999645, -3.464101615137751278, -9.206249998770948295 ) ) ;
#18808=CARTESIAN_POINT ( 'NONE',  ( 27.69756682629397915, 5.407089921784862696, 162.3720029866663594 ) ) ;
#18835=ORIENTED_EDGE ( 'NONE', *, *, #35764, .F. ) ;
#18840=CARTESIAN_POINT ( 'NONE',  ( 26.75643035624999655, 7.049594010296217766E-16, -4.078124999385480010 ) ) ;
#18844=CARTESIAN_POINT ( 'NONE',  ( 15.24356964375000167, -3.323476615752272600, -7.303124999385448568 ) ) ;
#18849=CARTESIAN_POINT ( 'NONE',  ( 36.59916218799832421, -3.464101615137751278, 159.4569602140672089 ) ) ;
#18853=DIRECTION ( 'NONE',  ( 0.000000000000000000, 0.000000000000000000, 1.000000000000000000 ) ) ;
#18854=CARTESIAN_POINT ( 'NONE',  ( 36.79853094953357129, 7.347880794884117764E-16, 161.7357555859521199 ) ) ;
#18869=CARTESIAN_POINT ( 'NONE',  ( 31.33122385594975512, 6.928203230275514990, 168.0864290250503643 ) ) ;
#18875=CARTESIAN_POINT ( 'NONE',  ( 20.99999999999999645, -6.928203230275506996, -7.031249998770932486 ) ) ;
#18878=CARTESIAN_POINT ( 'NONE',  ( 24.75271252598717808, 3.604726614523236616, 164.5306281710264216 ) ) ;
#18882=VERTEX_POINT ( 'NONE', #21053 ) ;
#18886=CARTESIAN_POINT ( 'NONE',  ( 24.58926402489574770, 0.000000000000000000, 159.8677550070055702 ) ) ;
#18889=CARTESIAN_POINT ( 'NONE',  ( 14.99999999999978684, 3.464101615137630485, -5.887500000000001954 ) ) ;
#18890=CARTESIAN_POINT ( 'NONE',  ( 23.87821517812500005, -4.985214923628404016, -8.090624999385454430 ) ) ;
#18899=CARTESIAN_POINT ( 'NONE',  ( 28.32956640036948315, -5.196152422706632912, 168.1984670498039236 ) ) ;
#18904=CARTESIAN_POINT ( 'NONE',  ( 18.12178482187500350, -4.985214923628407568, -2.428124999385494753 ) ) ;
#18908=EDGE_CURVE ( 'NONE', #7860, #8427, #24767, .T. ) ;
#18913=CARTESIAN_POINT ( 'NONE',  ( 37.24626209435294300, -3.604726614523238837, 164.0586977410752638 ) ) ;
#18928=CARTESIAN_POINT ( 'NONE',  ( 18.00000000000000000, 5.196152422706630247, -1.874999999999987788 ) ) ;
#18929=CARTESIAN_POINT ( 'NONE',  ( 24.55170959427540822, 3.604726614523240613, 162.2331541485523587 ) ) ;
#18930=CARTESIAN_POINT ( 'NONE',  ( 36.75277418448394684, 3.464101615137759271, 161.2127533682296132 ) ) ;
#18935=ORIENTED_EDGE ( 'NONE', *, *, #31965, .T. ) ;
#18938=CARTESIAN_POINT ( 'NONE',  ( 20.99999999999999645, 6.928203230275506996, -1.012500000000014388 ) ) ;
#18941=CARTESIAN_POINT ( 'NONE',  ( 26.75643035624999655, -3.323476615752267715, -5.465624999385500615 ) ) ;
#18944=LINE ( 'NONE', #22525, #6453 ) ;
#18954=CARTESIAN_POINT ( 'NONE',  ( 36.97989235558041798, 7.646167579472015790E-16, 161.0140776950323698 ) ) ;
#18957=CARTESIAN_POINT ( 'NONE',  ( 29.54925929127992745, 5.908847637349538218, 159.6727443940304738 ) ) ;
#18965=CARTESIAN_POINT ( 'NONE',  ( 27.97700992647863316, 5.407089921784856479, 165.5660522374229799 ) ) ;
#18966=CARTESIAN_POINT ( 'NONE',  ( 15.24356964375000167, -3.323476615752272600, -5.503124999385465621 ) ) ;
#18968=CARTESIAN_POINT ( 'NONE',  ( 25.48152094116770883, 0.000000000000000000, 170.0662982274954800 ) ) ;
#18974=ORIENTED_EDGE ( 'NONE', *, *, #27471, .T. ) ;
#18978=CARTESIAN_POINT ( 'NONE',  ( 21.00000000000000000, 6.646953231504538984, -4.303124999385465443 ) ) ;
#18981=CARTESIAN_POINT ( 'NONE',  ( 15.00000000000000000, 0.000000000000000000, -8.493749998770949716 ) ) ;
#18989=CARTESIAN_POINT ( 'NONE',  ( 36.89981801693102170, 3.604726614523243278, 160.0988238161606034 ) ) ;
#18997=VERTEX_POINT ( 'NONE', #554 ) ;
#19012=CARTESIAN_POINT ( 'NONE',  ( 18.00000000000000355, -5.196152422706632912, -2.175000000000010481 ) ) ;
#19024=CARTESIAN_POINT ( 'NONE',  ( 18.12178482187500350, -4.985214923628407568, -6.028124999385486404 ) ) ;
#19029=CARTESIAN_POINT ( 'NONE',  ( 26.75643035624999655, 3.323476615752271268, -7.078124999385466687 ) ) ;
#19031=( BOUNDED_CURVE ( )  B_SPLINE_CURVE ( 2, ( #21579, #30478, #18742, #7723, #4126, #16448, #25151 ),
 .UNSPECIFIED., .F., .F. ) 
 B_SPLINE_CURVE_WITH_KNOTS ( ( 3, 2, 2, 3 ),
 ( 0.5434782608695644113, 0.5507246376811587574, 0.5579710144927531035, 0.5652173913043473386 ),
 .UNSPECIFIED. ) 
 CURVE ( )  GEOMETRIC_REPRESENTATION_ITEM ( )  RATIONAL_B_SPLINE_CURVE ( ( 1.000000000000014433, 0.8660254037844243857, 1.000000000000000000, 0.8660254037844387076, 1.000000000000000000, 0.8660254037844469233, 0.9999999999999917843 ) ) 
 REPRESENTATION_ITEM ( '' )  );
#19032=FACE_OUTER_BOUND ( 'NONE', #10228, .T. ) ;
#19037=CARTESIAN_POINT ( 'NONE',  ( 28.48305061405702787, 5.725134515572932514, 159.4403097883560179 ) ) ;
#19042=CARTESIAN_POINT ( 'NONE',  ( 19.80074372294634344, 5.630122097104456991, -7.999999999999998224 ) ) ;
#19051=DIRECTION ( 'NONE',  ( 1.000000000000000000, 0.000000000000000000, 0.000000000000000000 ) ) ;
#19062=ORIENTED_EDGE ( 'NONE', *, *, #30444, .F. ) ;
#19063=DIRECTION ( 'NONE',  ( 0.000000000000000000, 0.000000000000000000, 1.000000000000000000 ) ) ;
#19066=CARTESIAN_POINT ( 'NONE',  ( 34.09877069215784218, -5.407089921784855591, 163.9011702523720544 ) ) ;
#19073=CARTESIAN_POINT ( 'NONE',  ( 24.00000000000000000, -5.196152422706629359, -4.293749998770940657 ) ) ;
#19077=CARTESIAN_POINT ( 'NONE',  ( 23.87821517812500005, -4.985214923628404016, -7.640624999385475569 ) ) ;
#19084=CARTESIAN_POINT ( 'NONE',  ( 28.21190614766015159, -5.196152422706632912, 166.8536042073800729 ) ) ;
#19088=CARTESIAN_POINT ( 'NONE',  ( 26.75643035624999655, 7.049594010296217766E-16, -2.278124999385483740 ) ) ;
#19092=VERTEX_POINT ( 'NONE', #33530 ) ;
#19100=CARTESIAN_POINT ( 'NONE',  ( 37.29201885929546023, 3.604726614523243278, 164.5816999575734201 ) ) ;
#19115=CARTESIAN_POINT ( 'NONE',  ( 15.00000000000000000, 3.464101615137752166, -1.387499999999984190 ) ) ;
#19116=CARTESIAN_POINT ( 'NONE',  ( 30.90225418466721763, -7.209453229046482114, 163.1832832459922713 ) ) ;
#19117=CARTESIAN_POINT ( 'NONE',  ( 27.73146011565660984, -5.196152422706638241, 161.3620809329249539 ) ) ;
#19119=CARTESIAN_POINT ( 'NONE',  ( 29.48995970988985604, 6.148715791637016537, 159.4803054849043917 ) ) ;
#19129=CARTESIAN_POINT ( 'NONE',  ( 26.75643035624999655, -3.323476615752267715, -5.915624999385464378 ) ) ;
#19130=EDGE_CURVE ( 'NONE', #21667, #25349, #5081, .T. ) ;
#19134=CARTESIAN_POINT ( 'NONE',  ( 37.41624727615045742, 7.347880794884125653E-16, 168.7962855074530069 ) ) ;
#19143=CARTESIAN_POINT ( 'NONE',  ( 36.93740393099094632, -3.604726614523235284, 160.5284327797126025 ) ) ;
#19144=CARTESIAN_POINT ( 'NONE',  ( 15.00000000000000000, 0.000000000000000000, -0.3937499987709536242 ) ) ;
#19146=CARTESIAN_POINT ( 'NONE',  ( 30.88019288723065259, -6.928203230275514990, 162.9311214624255797 ) ) ;
#19155=CARTESIAN_POINT ( 'NONE',  ( 31.10325711637897683, -7.209453229046475009, 165.4807572684663342 ) ) ;
#19156=CARTESIAN_POINT ( 'NONE',  ( 18.12178482187499640, 4.985214923628404904, -6.065624999385454963 ) ) ;
#19159=CARTESIAN_POINT ( 'NONE',  ( 17.99789842368819848, 4.964426654962620589, -7.999999999999996447 ) ) ;
#19160=CARTESIAN_POINT ( 'NONE',  ( 25.40308077269482112, 0.000000000000000000, 169.1697229992128939 ) ) ;
#19166=ORIENTED_EDGE ( 'NONE', *, *, #34621, .T. ) ;
#19171=CARTESIAN_POINT ( 'NONE',  ( 18.12178482187500350, -4.985214923628407568, -3.215624999385463312 ) ) ;
#19173=CARTESIAN_POINT ( 'NONE',  ( 15.00000000000000000, 0.000000000000000000, -8.943749998770956111 ) ) ;
#19175=VERTEX_POINT ( 'NONE', #22171 ) ;
#19180=EDGE_CURVE ( 'NONE', #590, #22708, #13443, .T. ) ;
#19185=CARTESIAN_POINT ( 'NONE',  ( 25.22662187717753568, 0.000000000000000000, 169.9474368419002985 ) ) ;
#19187=ORIENTED_EDGE ( 'NONE', *, *, #8048, .F. ) ;
#19188=DIRECTION ( 'NONE',  ( 0.08715574274765143514, 0.000000000000000000, 0.9961946980917462113 ) ) ;
#19189=CARTESIAN_POINT ( 'NONE',  ( 36.68087069682425039, 7.347880794884117764E-16, 160.3908927435282692 ) ) ;
#19196=ORIENTED_EDGE ( 'NONE', *, *, #1070, .F. ) ;
#19205=CARTESIAN_POINT ( 'NONE',  ( 20.99999999999999645, 0.000000000000000000, -8.000000000000000000 ) ) ;
#19207=CARTESIAN_POINT ( 'NONE',  ( 18.00000000000000000, 5.196152422706630247, -9.074999999999999289 ) ) ;
#19215=CARTESIAN_POINT ( 'NONE',  ( 23.87821517812500005, -4.985214923628404016, -6.403124999385473082 ) ) ;
#19219=CARTESIAN_POINT ( 'NONE',  ( 31.00765816110621031, -6.928203230275506996, 164.3880562096091467 ) ) ;
#19222=CARTESIAN_POINT ( 'NONE',  ( 37.63846293671737442, -3.604726614523238837, 168.5415738824881373 ) ) ;
#19234=CARTESIAN_POINT ( 'NONE',  ( 15.02283181144952628, 7.347880794884122694E-16, 50.52293445648592751 ) ) ;
#19236=EDGE_CURVE ( 'NONE', #23945, #7924, #13706, .T. ) ;
#19249=APPLICATION_CONTEXT ( 'automotive_design' ) ;
#19258=CARTESIAN_POINT ( 'NONE',  ( 34.07262396933355575, 5.407089921784857367, 163.6023118429445162 ) ) ;
#19263=ORIENTED_EDGE ( 'NONE', *, *, #15354, .F. ) ;
#19265=CARTESIAN_POINT ( 'NONE',  ( 26.99999999999999645, -3.464101615137751278, -3.806249998770967480 ) ) ;
#19267=CARTESIAN_POINT ( 'NONE',  ( 24.00000000000000000, -5.196152422706629359, -1.200000000000006617 ) ) ;
#19275=VECTOR ( 'NONE', #35701, 1000.000000000000000 ) ;
#19276=CARTESIAN_POINT ( 'NONE',  ( 25.13507686385291251, 3.464101615137752166, 166.1064243038051131 ) ) ;
#19282=CARTESIAN_POINT ( 'NONE',  ( 15.24356964374999990, 3.323476615752268604, -1.190624999385493377 ) ) ;
#19288=CARTESIAN_POINT ( 'NONE',  ( 25.25927379726847022, -3.464101615137840984, 167.5260017485858555 ) ) ;
#19291=DIRECTION ( 'NONE',  ( 0.000000000000000000, 0.000000000000000000, 1.000000000000000000 ) ) ;
#19292=CARTESIAN_POINT ( 'NONE',  ( 37.16782192588006239, -3.604726614523238837, 163.1621225127927062 ) ) ;
#19297=CARTESIAN_POINT ( 'NONE',  ( 23.99999999999999645, 5.196152422706631135, -2.793749998770966858 ) ) ;
#19300=EDGE_CURVE ( 'NONE', #16385, #10052, #15922, .T. ) ;
#19308=CARTESIAN_POINT ( 'NONE',  ( 24.00000000000000000, -5.196152422706629359, -2.549999999999996714 ) ) ;
#19310=CARTESIAN_POINT ( 'NONE',  ( 30.94147426890365793, -7.209453229046482114, 163.6315708601335643 ) ) ;
#19311=CARTESIAN_POINT ( 'NONE',  ( 24.85726793373765631, -3.464101615137761048, 162.9310537024133509 ) ) ;
#19322=CARTESIAN_POINT ( 'NONE',  ( 15.24356964374999990, 0.000000000000000000, -9.703124999385471128 ) ) ;
#19334=CARTESIAN_POINT ( 'NONE',  ( 37.02238078016989675, 3.604726614523238837, 161.4997226103520802 ) ) ;
#19335=CARTESIAN_POINT ( 'NONE',  ( 21.00000000000000000, 6.928203230275506996, -0.9562499987709413007 ) ) ;
#19340=DIRECTION ( 'NONE',  ( 0.08715574274765150453, 0.000000000000000000, 0.9961946980917461003 ) ) ;
#19344=ORIENTED_EDGE ( 'NONE', *, *, #35882, .F. ) ;
#19345=CARTESIAN_POINT ( 'NONE',  ( 27.82012958953286130, 5.407089921784856479, 163.7729017808578362 ) ) ;
#19346=CARTESIAN_POINT ( 'NONE',  ( 26.75643035624999655, 3.323476615752271712, -6.178124999385475213 ) ) ;
#19349=CARTESIAN_POINT ( 'NONE',  ( 31.42927406654086298, -6.928203230275514990, 169.2071480604036253 ) ) ;
#19355=ORIENTED_EDGE ( 'NONE', *, *, #33739, .T. ) ;
#19356=ORIENTED_EDGE ( 'NONE', *, *, #13571, .F. ) ;
#19359=CARTESIAN_POINT ( 'NONE',  ( 26.75643035624999655, 3.323476615752271712, -3.028124999385441107 ) ) ;
#19363=CARTESIAN_POINT ( 'NONE',  ( 23.87821517812500005, -4.985214923628404016, -2.803124999385481431 ) ) ;
#19365=ORIENTED_EDGE ( 'NONE', *, *, #5231, .F. ) ;
#19375=ORIENTED_EDGE ( 'NONE', *, *, #27762, .T. ) ;
#19377=DIRECTION ( 'NONE',  ( 0.9961946980917462113, 0.000000000000000000, -0.08715574274765178209 ) ) ;
#19378=FACE_OUTER_BOUND ( 'NONE', #11972, .T. ) ;
#19395=CARTESIAN_POINT ( 'NONE',  ( 18.91622499444735084, 5.725135169889072451, -9.986452812430625769 ) ) ;
#19401=CARTESIAN_POINT ( 'NONE',  ( 26.75643035624999655, -3.323476615752267715, -7.265624999385483562 ) ) ;
#19414=CIRCLE ( 'NONE', #9719, 4.000000000000001776 ) ;
#19416=CYLINDRICAL_SURFACE ( 'NONE', #33381, 6.000000000000001776 ) ;
#19420=CARTESIAN_POINT ( 'NONE',  ( 21.00000000000000355, 0.000000000000000000, 50.00000000000001421 ) ) ;
#19425=DIRECTION ( 'NONE',  ( 1.000000000000000000, 0.000000000000000000, 0.000000000000000000 ) ) ;
#19432=VECTOR ( 'NONE', #3524, 1000.000000000000000 ) ;
#19433=ORIENTED_EDGE ( 'NONE', *, *, #17548, .T. ) ;
#19439=CARTESIAN_POINT ( 'NONE',  ( 24.64158895398392701, -3.604726614523240613, 163.2604799309594910 ) ) ;
#19440=CARTESIAN_POINT ( 'NONE',  ( 15.24356964374999990, 0.000000000000000000, -0.2531249993854844949 ) ) ;
#19446=CARTESIAN_POINT ( 'NONE',  ( 15.00000000000000178, -3.464101615137757051, -4.406249998770951137 ) ) ;
#19447=CARTESIAN_POINT ( 'NONE',  ( 15.24356964374999990, 3.323476615752268604, -2.878124999385485161 ) ) ;
#19457=CARTESIAN_POINT ( 'NONE',  ( 27.96351228082934171, 5.196152422706630247, 164.0144493178186167 ) ) ;
#19463=CARTESIAN_POINT ( 'NONE',  ( 15.24356964374999990, 0.000000000000000000, -2.503124999385486493 ) ) ;
#19467=ORIENTED_EDGE ( 'NONE', *, *, #1357, .T. ) ;
#19468=CARTESIAN_POINT ( 'NONE',  ( 24.00000000000000000, -5.196152422706629359, -6.599999999999994316 ) ) ;
#19472=CARTESIAN_POINT ( 'NONE',  ( 34.18538171151332961, 5.407089921784862696, 164.8911387336007408 ) ) ;
#19476=( BOUNDED_CURVE ( )  B_SPLINE_CURVE ( 2, ( #28449, #2853, #11767, #11, #11577, #20500, #17464 ),
 .UNSPECIFIED., .F., .F. ) 
 B_SPLINE_CURVE_WITH_KNOTS ( ( 3, 2, 2, 3 ),
 ( 0.2173913043478258034, 0.2246376811594198442, 0.2318840579710139127, 0.2391304347826079535 ),
 .UNSPECIFIED. ) 
 CURVE ( )  GEOMETRIC_REPRESENTATION_ITEM ( )  RATIONAL_B_SPLINE_CURVE ( ( 1.000000000000005107, 0.8660254037844334896, 1.000000000000000000, 0.8660254037844387076, 1.000000000000000000, 0.8660254037844525854, 0.9999999999999861222 ) ) 
 REPRESENTATION_ITEM ( '' )  );
#19479=DIRECTION ( 'NONE',  ( 0.000000000000000000, 0.000000000000000000, 1.000000000000000000 ) ) ;
#19487=CARTESIAN_POINT ( 'NONE',  ( 26.99999999999999645, -3.464101615137751278, -2.962500000000017675 ) ) ;
#19488=CARTESIAN_POINT ( 'NONE',  ( 31.01746318205820785, 6.928203230275514990, 164.5001281119201053 ) ) ;
#19490=CARTESIAN_POINT ( 'NONE',  ( 27.46224632087531958, 5.407089921784862696, 159.6822773018186297 ) ) ;
#19492=CARTESIAN_POINT ( 'NONE',  ( 27.63994658577156827, 5.196152422706636465, 160.3160764999286698 ) ) ;
#19494=FACE_OUTER_BOUND ( 'NONE', #13614, .T. ) ;
#19500=CARTESIAN_POINT ( 'NONE',  ( 34.22502607998692525, -5.196152422706635576, 166.7416000626326422 ) ) ;
#19502=CARTESIAN_POINT ( 'NONE',  ( 21.00000000000000000, -6.646953231504538984, -10.04062499938548392 ) ) ;
#19506=CARTESIAN_POINT ( 'NONE',  ( 15.00000000000000000, 0.000000000000000000, -6.243749998770947940 ) ) ;
#19516=CARTESIAN_POINT ( 'NONE',  ( 33.78501001826630556, -5.407089921784855591, 160.3148693392417670 ) ) ;
#19519=DIRECTION ( 'NONE',  ( 1.000000000000000000, 0.000000000000000000, 0.000000000000000000 ) ) ;
#19525=DIRECTION ( 'NONE',  ( 0.000000000000000000, 0.000000000000000000, 1.000000000000000000 ) ) ;
#19527=CARTESIAN_POINT ( 'NONE',  ( 37.21194452064604974, -3.604726614523235284, 163.6664460787016253 ) ) ;
#19528=CARTESIAN_POINT ( 'NONE',  ( 23.87821517812500005, -4.985214923628404016, -6.290624999385458160 ) ) ;
#19530=CARTESIAN_POINT ( 'NONE',  ( 37.52080268400804641, -3.604726614523238837, 167.1967110400642866 ) ) ;
#19531=CARTESIAN_POINT ( 'NONE',  ( 28.24132121073036927, -5.196152422706638241, 167.1898199167616781 ) ) ;
#19537=ORIENTED_EDGE ( 'NONE', *, *, #20756, .T. ) ;
#19538=( BOUNDED_CURVE ( )  B_SPLINE_CURVE ( 2, ( #31529, #5554, #8596, #17139, #5742, #2899, #14471 ),
 .UNSPECIFIED., .F., .F. ) 
 B_SPLINE_CURVE_WITH_KNOTS ( ( 3, 2, 2, 3 ),
 ( 0.3043478260869560414, 0.3115942028985501655, 0.3188405797101442340, 0.3260869565217384136 ),
 .UNSPECIFIED. ) 
 CURVE ( )  GEOMETRIC_REPRESENTATION_ITEM ( )  RATIONAL_B_SPLINE_CURVE ( ( 1.000000000000009326, 0.8660254037844296038, 1.000000000000000000, 0.8660254037844387076, 1.000000000000000000, 0.8660254037844520303, 0.9999999999999866773 ) ) 
 REPRESENTATION_ITEM ( '' )  );
#19541=CARTESIAN_POINT ( 'NONE',  ( 15.24356964374999990, 3.323476615752268604, -3.328124999385480898 ) ) ;
#19544=CARTESIAN_POINT ( 'NONE',  ( 18.12178482187499640, 4.985214923628404904, -0.7781249993854821856 ) ) ;
#19557=DIRECTION ( 'NONE',  ( 0.000000000000000000, 0.000000000000000000, 1.000000000000000000 ) ) ;
#19559=CARTESIAN_POINT ( 'NONE',  ( 15.00000000000000000, 0.000000000000000000, -7.143749998770959841 ) ) ;
#19564=CARTESIAN_POINT ( 'NONE',  ( 18.00000000000000000, 5.196152422706630247, -4.518749998770942966 ) ) ;
#19565=VERTEX_POINT ( 'NONE', #9383 ) ;
#19571=CARTESIAN_POINT ( 'NONE',  ( 37.11229162342512211, 7.347880794884117764E-16, 165.3220564990824073 ) ) ;
#19575=CARTESIAN_POINT ( 'NONE',  ( 15.00000000000000178, -3.464101615137757051, -8.962500000000012790 ) ) ;
#19580=CARTESIAN_POINT ( 'NONE',  ( 18.12178482187500350, -4.985214923628407568, -7.378124999385477167 ) ) ;
#19588=CARTESIAN_POINT ( 'NONE',  ( 31.33367511126808935, -7.209453229046482114, 168.1144470015464378 ) ) ;
#19589=EDGE_CURVE ( 'NONE', #14162, #31631, #4807, .T. ) ;
#19592=CARTESIAN_POINT ( 'NONE',  ( 18.00000000000000355, -5.196152422706632912, -7.574999999999998401 ) ) ;
#19600=MECHANICAL_DESIGN_GEOMETRIC_PRESENTATION_REPRESENTATION('',(#14744),#7500);
#19612=CARTESIAN_POINT ( 'NONE',  ( 17.01522120763301871, 4.898587196589416773E-16, 50.34862297099062545 ) ) ;
#19620=ORIENTED_EDGE ( 'NONE', *, *, #17390, .T. ) ;
#19622=LINE ( 'NONE', #5191, #8709 ) ;
#19627=CARTESIAN_POINT ( 'NONE',  ( 30.88754665307854097, 7.209453229046475009, 163.0151753906892793 ) ) ;
#19630=ORIENTED_EDGE ( 'NONE', *, *, #534, .F. ) ;
#19631=ORIENTED_EDGE ( 'NONE', *, *, #27204, .T. ) ;
#19633=CARTESIAN_POINT ( 'NONE',  ( 21.00000000000000000, 6.928203230275506996, -5.006249998770934795 ) ) ;
#19634=CARTESIAN_POINT ( 'NONE',  ( 23.87821517812499650, 4.985214923628404904, -2.540624999385482141 ) ) ;
#19645=DIRECTION ( 'NONE',  ( 1.000000000000000000, 0.000000000000000000, 0.000000000000000000 ) ) ;
#19646=CARTESIAN_POINT ( 'NONE',  ( 28.01580572647793943, -5.196152422706632912, 164.6121661366736078 ) ) ;
#19650=CARTESIAN_POINT ( 'NONE',  ( 15.24356964374999990, 0.000000000000000000, -2.053124999385480542 ) ) ;
#19659=CARTESIAN_POINT ( 'NONE',  ( 37.01420992928731835, 7.646167579472024665E-16, 161.4063293574060083 ) ) ;
#19675=CARTESIAN_POINT ( 'NONE',  ( 23.99999999999999645, 5.196152422706631135, -4.649999999999987921 ) ) ;
#19676=CARTESIAN_POINT ( 'NONE',  ( 25.40019891165470511, -3.899351167896716319, -7.999999999999994671 ) ) ;
#19677=CARTESIAN_POINT ( 'NONE',  ( 36.86059793269458140, 3.604726614523243278, 159.6505362020193104 ) ) ;
#19679=CARTESIAN_POINT ( 'NONE',  ( 36.58935716683210870, -3.464101615137755275, 159.3448883093075779 ) ) ;
#19687=DIRECTION ( 'NONE',  ( 0.9961946980917462113, 0.000000000000000000, -0.08715574274765118534 ) ) ;
#19689=CARTESIAN_POINT ( 'NONE',  ( 18.12178482187500350, -4.985214923628407568, -8.278124999385488181 ) ) ;
#19692=CARTESIAN_POINT ( 'NONE',  ( 28.36878648460592700, -5.196152422706632912, 168.6467546639452166 ) ) ;
#19693=CARTESIAN_POINT ( 'NONE',  ( 37.05669835387680422, 3.604726614523243278, 161.8919742727257187 ) ) ;
#19699=( BOUNDED_CURVE ( )  B_SPLINE_CURVE ( 3, ( #23255, #17385, #25902, #35168 ),
 .UNSPECIFIED., .F., .F. ) 
 B_SPLINE_CURVE_WITH_KNOTS ( ( 4, 4 ),
 ( 3.141592653589793116, 4.712388980384647930 ),
 .UNSPECIFIED. ) 
 CURVE ( )  GEOMETRIC_REPRESENTATION_ITEM ( )  RATIONAL_B_SPLINE_CURVE ( ( 1.000000000000000000, 0.8047378541243747074, 0.8047378541243747074, 1.000000000000000000 ) ) 
 REPRESENTATION_ITEM ( '' )  );
#19703=CARTESIAN_POINT ( 'NONE',  ( 33.91574363238778034, 5.407089921784857367, 161.8091613863793725 ) ) ;
#19705=CARTESIAN_POINT ( 'NONE',  ( 18.00000000000000000, 5.196152422706630247, -0.4687499987709453642 ) ) ;
#19713=CARTESIAN_POINT ( 'NONE',  ( 24.74614436184151955, 0.000000000000000000, 161.6609054635707423 ) ) ;
#19716=CARTESIAN_POINT ( 'NONE',  ( 33.99418380086066804, 5.407089921784857367, 162.7057366146619586 ) ) ;
#19717=CARTESIAN_POINT ( 'NONE',  ( 15.24356964374999990, 3.323476615752268604, -6.478124999385451055 ) ) ;
#19719=CARTESIAN_POINT ( 'NONE',  ( 31.19640481644053764, 7.209453229046482114, 166.5454403520519122 ) ) ;
#19720=CARTESIAN_POINT ( 'NONE',  ( 37.13843834614232264, -3.464101615137755275, 165.6209149072855666 ) ) ;
#19729=ORIENTED_EDGE ( 'NONE', *, *, #29819, .F. ) ;
#19733=CARTESIAN_POINT ( 'NONE',  ( 21.00000000000000000, -6.646953231504538984, -6.778124999385457983 ) ) ;
#19736=CARTESIAN_POINT ( 'NONE',  ( 21.00000000000000000, 6.646953231504538984, -1.265624999385487115 ) ) ;
#19743=VECTOR ( 'NONE', #23898, 1000.000000000000000 ) ;
#19749=CARTESIAN_POINT ( 'NONE',  ( 26.99999999999999289, 0.000000000000000000, -8.000000000000000000 ) ) ;
#19759=( BOUNDED_CURVE ( )  B_SPLINE_CURVE ( 2, ( #23149, #13875, #34691, #36789, #2299, #13690, #25238 ),
 .UNSPECIFIED., .F., .F. ) 
 B_SPLINE_CURVE_WITH_KNOTS ( ( 3, 2, 2, 3 ),
 ( 0.2608695652173921298, 0.2681159420289864759, 0.2753623188405807110, 0.2826086956521750015 ),
 .UNSPECIFIED. ) 
 CURVE ( )  GEOMETRIC_REPRESENTATION_ITEM ( )  RATIONAL_B_SPLINE_CURVE ( ( 0.9999999999999845679, 0.8660254037844541397, 1.000000000000000000, 0.8660254037844387076, 1.000000000000000000, 0.8660254037844181685, 1.000000000000020428 ) ) 
 REPRESENTATION_ITEM ( '' )  );
#19767=CARTESIAN_POINT ( 'NONE',  ( 21.00000000000000000, 6.928203230275506996, -9.112500000000002487 ) ) ;
#19768=ORIENTED_EDGE ( 'NONE', *, *, #28427, .F. ) ;
#19773=CARTESIAN_POINT ( 'NONE',  ( 26.75643035624999655, 7.049594010296217766E-16, -7.228124999385493687 ) ) ;
#19780=CARTESIAN_POINT ( 'NONE',  ( 34.53836246964132073, 5.407089921784862696, 168.9257272608723213 ) ) ;
#19782=CARTESIAN_POINT ( 'NONE',  ( 36.64491895294136015, 3.464101615137448409, 159.9799624305653936 ) ) ;
#19796=ORIENTED_EDGE ( 'NONE', *, *, #352, .T. ) ;
#19798=DIRECTION ( 'NONE',  ( 0.000000000000000000, 0.000000000000000000, 1.000000000000000000 ) ) ;
#19802=CARTESIAN_POINT ( 'NONE',  ( 18.00000000000000000, 5.196152422706630247, -5.418749998770955756 ) ) ;
#19804=CARTESIAN_POINT ( 'NONE',  ( 28.09424589495082714, -5.196152422706632912, 165.5087413649561938 ) ) ;
#19811=CIRCLE ( 'NONE', #30681, 4.000000000000001776 ) ;
#19815=CARTESIAN_POINT ( 'NONE',  ( 30.82871652672388052, -7.209453229046475009, 162.3427439694773398 ) ) ;
#19819=EDGE_LOOP ( 'NONE', ( #1514, #19630, #7108, #3087 ) ) ;
#19820=CARTESIAN_POINT ( 'NONE',  ( 24.00000000000000000, -5.196152422706629359, -5.643749998770958065 ) ) ;
#19821=CARTESIAN_POINT ( 'NONE',  ( 18.12178482187500350, -4.985214923628407568, -3.215624999385463312 ) ) ;
#19823=LINE ( 'NONE', #25300, #5615 ) ;
#19829=CARTESIAN_POINT ( 'NONE',  ( 34.09102412561951212, 5.196152422706631135, 165.2099507155409412 ) ) ;
#19834=CARTESIAN_POINT ( 'NONE',  ( 20.99999999999999645, -6.646953231504538984, -3.290624999385483918 ) ) ;
#19842=CARTESIAN_POINT ( 'NONE',  ( 30.86303410043077022, -7.209453229046482114, 162.7349956318509783 ) ) ;
#19847=CARTESIAN_POINT ( 'NONE',  ( 20.99999999999999645, 0.000000000000000000, -8.000000000000000000 ) ) ;
#19857=CARTESIAN_POINT ( 'NONE',  ( 15.00000000000000178, -3.464101615137757051, -3.562500000000000888 ) ) ;
#19859=CARTESIAN_POINT ( 'NONE',  ( 24.47980610650860100, -3.604726614523244610, 161.4112935226266359 ) ) ;
#19861=CARTESIAN_POINT ( 'NONE',  ( 37.57146195948011069, 3.604726614523238837, 167.7757492083300690 ) ) ;
#19863=DIRECTION ( 'NONE',  ( 0.000000000000000000, 0.000000000000000000, 1.000000000000000000 ) ) ;
#19870=CARTESIAN_POINT ( 'NONE',  ( 15.24356964375000167, -3.323476615752272600, -8.765624999385490668 ) ) ;
#19872=AXIS2_PLACEMENT_3D ( 'NONE', #15980, #12941, #1370 ) ;
#19874=DIRECTION ( 'NONE',  ( 0.08715574274765150453, 0.000000000000000000, 0.9961946980917461003 ) ) ;
#19876=CARTESIAN_POINT ( 'NONE',  ( 37.09265009776020605, 7.646167579472024665E-16, 162.3029045856885659 ) ) ;
#19887=CARTESIAN_POINT ( 'NONE',  ( 36.81974367828161121, -3.604726614523235284, 159.1835699372887802 ) ) ;
#19888=CARTESIAN_POINT ( 'NONE',  ( 26.99999999999999645, -3.464101615137751278, -0.6562499987709655702 ) ) ;
#19897=CARTESIAN_POINT ( 'NONE',  ( 33.95496371662422064, 5.407089921784857367, 162.2574490005206655 ) ) ;
#19898=VECTOR ( 'NONE', #5845, 1000.000000000000000 ) ;
#19899=CARTESIAN_POINT ( 'NONE',  ( 15.24356964374999990, 0.000000000000000000, -8.690624999385471838 ) ) ;
#19901=CARTESIAN_POINT ( 'NONE',  ( 28.10284103007056089, -5.407089921784865361, 167.0043083327929878 ) ) ;
#19902=CARTESIAN_POINT ( 'NONE',  ( 25.21024869186565098, -3.464101615137761048, 166.9656422296849314 ) ) ;
#19908=VERTEX_POINT ( 'NONE', #21292 ) ;
#19915=CARTESIAN_POINT ( 'NONE',  ( 21.00000000000000000, 6.646953231504538984, -0.8156249993854914893 ) ) ;
#19922=ADVANCED_FACE ( 'NONE', ( #15974 ), #30371, .F. ) ;
#19936=CARTESIAN_POINT ( 'NONE',  ( 23.99999999999999645, 5.196152422706631135, -4.593749998770962684 ) ) ;
#19940=CARTESIAN_POINT ( 'NONE',  ( 15.24356964374999990, 0.000000000000000000, -0.5906249993854750802 ) ) ;
#19947=CARTESIAN_POINT ( 'NONE',  ( 24.00000000000000000, -5.196152422706629359, -9.750000000000008882 ) ) ;
#19948=ORIENTED_EDGE ( 'NONE', *, *, #11558, .T. ) ;
#19952=CARTESIAN_POINT ( 'NONE',  ( 15.24356964374999990, 3.323476615752268604, -10.19062499938547184 ) ) ;
#19957=CARTESIAN_POINT ( 'NONE',  ( 34.22460179574976991, 5.407089921784862696, 165.3394263477420054 ) ) ;
#19963=CARTESIAN_POINT ( 'NONE',  ( 34.42560472746153977, 5.407089921784857367, 167.6369003702161251 ) ) ;
#19978=CARTESIAN_POINT ( 'NONE',  ( 18.00000000000000000, 5.196152422706630247, -4.068749998770964993 ) ) ;
#19990=CARTESIAN_POINT ( 'NONE',  ( 33.82423010250274586, -5.407089921784855591, 160.7631569533830600 ) ) ;
#19991=CARTESIAN_POINT ( 'NONE',  ( 15.24356964374999990, 3.323476615752268604, -1.640624999385488891 ) ) ;
#19994=ORIENTED_EDGE ( 'NONE', *, *, #36236, .F. ) ;
#19997=CARTESIAN_POINT ( 'NONE',  ( 18.00000000000000355, -5.196152422706632912, -7.068749998770940124 ) ) ;
#19998=CARTESIAN_POINT ( 'NONE',  ( 18.12178482187499640, 4.985214923628404904, -2.465624999385462868 ) ) ;
#19999=CARTESIAN_POINT ( 'NONE',  ( 36.56647878446842981, 3.464101615137479495, 159.0833872022827791 ) ) ;
#20000=CARTESIAN_POINT ( 'NONE',  ( 24.99999999999999289, 0.000000000000000000, -8.000000000000000000 ) ) ;
#20005=CARTESIAN_POINT ( 'NONE',  ( 33.93414378867374381, 5.196152422706631135, 163.4168002589758260 ) ) ;
#20009=CARTESIAN_POINT ( 'NONE',  ( 18.12178482187499640, 4.985214923628404904, -4.378124999385474503 ) ) ;
#20010=CARTESIAN_POINT ( 'NONE',  ( 20.99999999999999645, -6.928203230275506996, -1.687500000000023981 ) ) ;
#20013=ORIENTED_EDGE ( 'NONE', *, *, #5504, .F. ) ;
#20019=CARTESIAN_POINT ( 'NONE',  ( 30.76498388983966237, 7.209453229046482114, 161.6142765964977741 ) ) ;
#20029=CARTESIAN_POINT ( 'NONE',  ( 26.99999999999999645, 7.347880794884117764E-16, -1.574999999999993072 ) ) ;
#20033=CARTESIAN_POINT ( 'NONE',  ( 26.99999999999999645, 3.464101615137755275, -4.687500000000006217 ) ) ;
#20035=CARTESIAN_POINT ( 'NONE',  ( 33.71474070067601048, 5.407089921784862696, 159.5116873639053097 ) ) ;
#20037=CARTESIAN_POINT ( 'NONE',  ( 25.10569328411516921, 3.604726614523236616, 168.5652166982980305 ) ) ;
#20048=CARTESIAN_POINT ( 'NONE',  ( 15.24356964374999990, 3.323476615752268604, -8.840624999385484628 ) ) ;
#20054=CARTESIAN_POINT ( 'NONE',  ( 24.63014976274829593, 3.604726614523240613, 163.1297293768349164 ) ) ;
#20061=ORIENTED_EDGE ( 'NONE', *, *, #1566, .F. ) ;
#20063=CARTESIAN_POINT ( 'NONE',  ( 34.28712454680172783, 5.196152422706631135, 167.4513887862474064 ) ) ;
#20065=CARTESIAN_POINT ( 'NONE',  ( 33.83389300460937932, 6.917534487978453051, 159.1041492265317174 ) ) ;
#20066=CARTESIAN_POINT ( 'NONE',  ( 23.99999999999999645, 5.196152422706631135, -1.893749998770954956 ) ) ;
#20075=CARTESIAN_POINT ( 'NONE',  ( 24.67427235751429748, 3.604726614523236616, 163.6340529427438639 ) ) ;
#20076=CARTESIAN_POINT ( 'NONE',  ( 21.00000000000000000, 6.646953231504538984, -6.553124999385445903 ) ) ;
#20079=CARTESIAN_POINT ( 'NONE',  ( 37.52733936471412335, 3.604726614523243278, 167.2714256424211499 ) ) ;
#20080=CARTESIAN_POINT ( 'NONE',  ( 25.13180852339276683, -3.464101615137761048, 166.0690670014023453 ) ) ;
#20081=LINE ( 'NONE', #3001, #19898 ) ;
#20093=CARTESIAN_POINT ( 'NONE',  ( 15.24356964374999990, 0.000000000000000000, -0.7031249993854904456 ) ) ;
#20104=CARTESIAN_POINT ( 'NONE',  ( 25.01087993033039325, 0.000000000000000000, 164.6868468578000488 ) ) ;
#20114=CARTESIAN_POINT ( 'NONE',  ( 23.87821517812500005, -4.985214923628404016, -0.8906249993854697955 ) ) ;
#20123=EDGE_CURVE ( 'NONE', #28188, #30148, #24499, .T. ) ;
#20124=EDGE_LOOP ( 'NONE', ( #21656, #21215, #6463, #22464, #20880 ) ) ;
#20129=CARTESIAN_POINT ( 'NONE',  ( 23.87821517812499650, 4.985214923628404904, -8.953124999385497773 ) ) ;
#20131=( BOUNDED_CURVE ( )  B_SPLINE_CURVE ( 2, ( #35772, #27067, #32185, #30098, #17792, #4130, #9630 ),
 .UNSPECIFIED., .F., .F. ) 
 B_SPLINE_CURVE_WITH_KNOTS ( ( 3, 2, 2, 3 ),
 ( 0.2608695652173909085, 0.2681159420289850326, 0.2753623188405790456, 0.2826086956521731142 ),
 .UNSPECIFIED. ) 
 CURVE ( )  GEOMETRIC_REPRESENTATION_ITEM ( )  RATIONAL_B_SPLINE_CURVE ( ( 1.000000000000007105, 0.8660254037844313801, 1.000000000000000000, 0.8660254037844387076, 1.000000000000000000, 0.8660254037844530295, 0.9999999999999856781 ) ) 
 REPRESENTATION_ITEM ( '' )  );
#20135=CARTESIAN_POINT ( 'NONE',  ( 27.98518077736123288, -5.407089921784865361, 165.6594454903691087 ) ) ;
#20139=CARTESIAN_POINT ( 'NONE',  ( 21.00000000000000355, 0.000000000000000000, 50.00000000000001421 ) ) ;
#20143=CARTESIAN_POINT ( 'NONE',  ( 37.57146195948011069, 3.604726614523238837, 167.7757492083300690 ) ) ;
#20146=CARTESIAN_POINT ( 'NONE',  ( 24.00000000000000000, -5.196152422706629359, -7.050000000000000711 ) ) ;
#20150=ADVANCED_FACE ( 'NONE', ( #6682 ), #18640, .T. ) ;
#20156=CARTESIAN_POINT ( 'NONE',  ( 24.93243976185750554, 0.000000000000000000, 163.7902716295174912 ) ) ;
#20165=ORIENTED_EDGE ( 'NONE', *, *, #31820, .T. ) ;
#20173=CARTESIAN_POINT ( 'NONE',  ( 18.12178482187499640, 4.985214923628404904, -3.028124999385484184 ) ) ;
#20176=ORIENTED_EDGE ( 'NONE', *, *, #7343, .T. ) ;
#20178=VERTEX_POINT ( 'NONE', #30930 ) ;
#20179=CARTESIAN_POINT ( 'NONE',  ( 23.99999999999999645, 5.196152422706631135, -6.393749998770958953 ) ) ;
#20180=CARTESIAN_POINT ( 'NONE',  ( 15.24356964375000167, -3.323476615752272600, -2.353124999385463489 ) ) ;
#20187=( BOUNDED_CURVE ( )  B_SPLINE_CURVE ( 2, ( #4800, #10305, #1584, #18673, #10121 ),
 .UNSPECIFIED., .F., .F. ) 
 B_SPLINE_CURVE_WITH_KNOTS ( ( 3, 2, 3 ),
 ( 0.7608695652173906865, 0.7681159420289852546, 0.7728738931639650422 ),
 .UNSPECIFIED. ) 
 CURVE ( )  GEOMETRIC_REPRESENTATION_ITEM ( )  RATIONAL_B_SPLINE_CURVE ( ( 1.000000000000012212, 0.8660254037844263841, 1.000000000000000000, 0.9120326476671286597, 0.9395835397632965602 ) ) 
 REPRESENTATION_ITEM ( '' )  );
#20188=CARTESIAN_POINT ( 'NONE',  ( 33.89492370443730351, 5.196152422706631135, 162.9685126448345329 ) ) ;
#20192=CARTESIAN_POINT ( 'NONE',  ( 15.24356964375000167, -3.323476615752272600, -5.165624999385461713 ) ) ;
#20193=DIRECTION ( 'NONE',  ( 0.000000000000000000, 0.000000000000000000, 1.000000000000000000 ) ) ;
#20200=CARTESIAN_POINT ( 'NONE',  ( 26.99999999999999645, 7.347880794884117764E-16, -6.018749998770944742 ) ) ;
#20202=CARTESIAN_POINT ( 'NONE',  ( 37.08938175740716758, -3.604726614523238837, 162.2655472845100917 ) ) ;
#20214=ORIENTED_EDGE ( 'NONE', *, *, #36489, .T. ) ;
#20215=CARTESIAN_POINT ( 'NONE',  ( 18.00000000000000000, 5.196152422706630247, -4.124999999999989342 ) ) ;
#20218=CARTESIAN_POINT ( 'NONE',  ( 30.76498388983966237, 7.209453229046482114, 161.6142765964977741 ) ) ;
#20220=CARTESIAN_POINT ( 'NONE',  ( 25.18740179294109183, 0.000000000000000000, 169.4991492277590339 ) ) ;
#20222=DIRECTION ( 'NONE',  ( 0.9961946980917462113, 0.000000000000000000, -0.08715574274765118534 ) ) ;
#20235=CARTESIAN_POINT ( 'NONE',  ( 26.99999999999999645, 7.347880794884117764E-16, -6.074999999999997513 ) ) ;
#20236=CARTESIAN_POINT ( 'NONE',  ( 34.39171143809891618, -5.196152422706629359, 168.6468224239574454 ) ) ;
#20239=( BOUNDED_CURVE ( )  B_SPLINE_CURVE ( 2, ( #31660, #11757, #5324, #35060, #26342, #23514, #17084, #378, #34506, #5687, #8546, #28623, #11200, #28440, #4, #37336, #25787, #34321, #31477, #2660, #14237, #11386, #17271, #28994, #23325, #23144, #34876, #28809, #2846, #14418, #25972, #34686, #20492, #20304, #31845, #17457, #32410, #3976, #1319, #9484, #21060, #32788, #26531, #562, #32598, #24080, #6450, #15549, #3785, #9671, #35246, #35813, #15361, #27107, #12887, #12128, #1131, #6638, #752, #12697, #12322, #9109, #21249, #24269, #27289, #9855, #23895, #35625, #29568, #942, #21434, #18023, #20675, #18213, #12516, #35436, #3605, #32974, #29754, #26914, #6823, #32223, #7028, #30137, #18399, #23704, #15172, #29375, #24452, #20871, #18594, #29948, #4168, #9299, #15738, #3413, #6262, #17839, #26719, #14982, #30884, #4907, #10039, #18785, #22361, #19155, #24818, #1504, #36002, #33539, #18965, #22178, #28036, #16488, #7579, #5097, #16676, #4539, #24634, #30703, #10787, #10417, #27667, #2068, #1691, #4350, #30326, #25001, #13642, #28223, #25195, #7392, #33724, #13451, #13266, #36371, #2251, #36747, #13830, #19527, #33910, #7952, #21992, #4723, #16300, #27847, #30519, #21616, #10598, #31074, #10229, #1880, #36557, #33357, #33167, #7213, #7765, #15929, #19345, #27478, #13080, #36184, #21804, #16115, #20264, #23289, #14379, #25562, #17609, #20075, #37300, #22921, #19716, #8690, #22545, #8874, #25937, #37114, #25377, #34094, #6023, #34466, #2620, #31256, #19897, #8509, #31802, #17231, #5282, #25747, #5840, #36926, #3180, #31994, #29140, #22735, #34833, #28582, #11349, #14196, #11162, #31620, #5648, #31439, #8144, #11714, #28769, #34284, #11531, #2809, #17044, #8327, #34645, #17418, #37480, #28958, #23102, #5461, #20452, #2996, #14566, #16862, #26118, #150, #28399, #10974, #2437, #14011, #32367, #26676, #29709, #6985, #3934, #23852, #35583, #6594, #9066, #15125, #21205, #26299, #30094, #26487, #706, #14756, #35390, #11902, #14940, #18168, #20637, #12278, #9439, #20826, #23469, #1089, #17979, #519, #899, #21017, #6406, #23660, #24038, #32551, #35770, #12469, #336, #18554, #35203, #9253, #32181 ),
 .UNSPECIFIED., .F., .F. ) 
 B_SPLINE_CURVE_WITH_KNOTS ( ( 3, 2, 2, 2, 2, 2, 2, 2, 2, 2, 2, 2, 2, 2, 2, 2, 2, 2, 2, 2, 2, 2, 2, 2, 2, 2, 2, 2, 2, 2, 2, 2, 2, 2, 2, 2, 2, 2, 2, 2, 2, 2, 2, 2, 2, 2, 2, 2, 2, 2, 2, 2, 2, 2, 2, 2, 2, 2, 2, 2, 2, 2, 2, 2, 2, 2, 2, 2, 2, 2, 2, 2, 2, 2, 2, 2, 2, 2, 2, 2, 2, 2, 2, 2, 2, 2, 2, 2, 2, 2, 2, 2, 2, 2, 2, 2, 2, 2, 2, 2, 2, 2, 2, 2, 2, 2, 2, 2, 2, 2, 2, 2, 2, 2, 2, 2, 2, 2, 2, 2, 2, 2, 2, 2, 2, 2, 2, 2, 2, 2, 2, 2, 2, 2, 3 ),
 ( 0.000000000000000000, 0.007499808115352593965, 0.01499961623070518793, 0.02249942434605778016, 0.02999923246141037586, 0.03749904057676296809, 0.04499884869211556032, 0.05249865680746815949, 0.05999846492282075172, 0.06749827303817333701, 0.07499808115352593618, 0.08249788926887852147, 0.08999769738423112064, 0.09749750549958371981, 0.1049973136149363190, 0.1124971217302889043, 0.1199969298456415034, 0.1274967379609940887, 0.1349965460763466740, 0.1424963541916992871, 0.1499961623070518724, 0.1574959704224044854, 0.1649957785377570429, 0.1724955866531096560, 0.1799953947684622413, 0.1874952028838148543, 0.1949950109991674396, 0.2024948191145200527, 0.2099946272298726380, 0.2174944353452252233, 0.2249942434605778085, 0.2324940515759304216, 0.2399938596912830069, 0.2474936678066355922, 0.2549934759219881775, 0.2624932840373407905, 0.2699930921526933481, 0.2774929002680460166, 0.2849927083833985741, 0.2924925164987511317, 0.2999923246141037447, 0.3074921327294563578, 0.3149919408448089708, 0.3224917489601615284, 0.3299915570755140859, 0.3374913651908667545, 0.3449911733062193120, 0.3524909814215719250, 0.3599907895369244826, 0.3674905976522771511, 0.3749904057676297087, 0.3824902138829822662, 0.3899900219983348792, 0.3974898301136874368, 0.4049896382290401053, 0.4124894463443926629, 0.4199892544597452759, 0.4274890625750978335, 0.4349888706904504465, 0.4424886788058030596, 0.4499884869211556171, 0.4574882950365082301, 0.4649881031518608432, 0.4724879112672134007, 0.4799877193825660138, 0.4874875274979185713, 0.4949873356132711844, 0.5024871437286237974, 0.5099869518439763549, 0.5174867599593290235, 0.5249865680746815810, 0.5324863761900341386, 0.5399861843053866961, 0.5474859924207393647, 0.5549858005360920332, 0.5624856086514444797, 0.5699854167667971483, 0.5774852248821498168, 0.5849850329975022634, 0.5924848411128549319, 0.5999846492282074895, 0.6074844573435601580, 0.6149842654589127156, 0.6224840735742652731, 0.6299838816896179416, 0.6374836898049703882, 0.6449834979203230567, 0.6524833060356757253, 0.6599831141510281718, 0.6674829222663808403, 0.6749827303817335089, 0.6824825384970860664, 0.6899823466124386240, 0.6974821547277911815, 0.7049819628431438501, 0.7124817709584964076, 0.7199815790738489651, 0.7274813871892016337, 0.7349811953045543023, 0.7424810034199067488, 0.7499808115352594173, 0.7574806196506119749, 0.7649804277659645324, 0.7724802358813172010, 0.7799800439966697585, 0.7874798521120224271, 0.7949796602273748736, 0.8024794683427275421, 0.8099792764580802107, 0.8174790845734326572, 0.8249788926887853258, 0.8324787008041379943, 0.8399785089194905519, 0.8474783170348431094, 0.8549781251501956669, 0.8624779332655483355, 0.8699777413809008930, 0.8774775494962534506, 0.8849773576116061191, 0.8924771657269586767, 0.8999769738423112342, 0.9074767819576639027, 0.9149765900730164603, 0.9224763981883690178, 0.9299762063037216864, 0.9374760144190742439, 0.9449758225344268014, 0.9524756306497793590, 0.9599754387651320275, 0.9674752468804846961, 0.9749750549958371426, 0.9824748631111898112, 0.9899746712265423687, 0.9974744793418949262, 1.000000000000000000 ),
 .UNSPECIFIED. ) 
 CURVE ( )  GEOMETRIC_REPRESENTATION_ITEM ( )  RATIONAL_B_SPLINE_CURVE ( ( 1.000000000000000000, 0.8660254037844387076, 1.000000000000000000, 0.8660254037844387076, 1.000000000000000000, 0.8660254037844387076, 1.000000000000000000, 0.8660254037844387076, 1.000000000000000000, 0.8660254037844387076, 1.000000000000000000, 0.8660254037844387076, 1.000000000000000000, 0.8660254037844387076, 1.000000000000000000, 0.8660254037844387076, 1.000000000000000000, 0.8660254037844387076, 1.000000000000000000, 0.8660254037844387076, 1.000000000000000000, 0.8660254037844387076, 1.000000000000000000, 0.8660254037844387076, 1.000000000000000000, 0.8660254037844387076, 1.000000000000000000, 0.8660254037844387076, 1.000000000000000000, 0.8660254037844387076, 1.000000000000000000, 0.8660254037844387076, 1.000000000000000000, 0.8660254037844387076, 1.000000000000000000, 0.8660254037844387076, 1.000000000000000000, 0.8660254037844387076, 1.000000000000000000, 0.8660254037844387076, 1.000000000000000000, 0.8660254037844387076, 1.000000000000000000, 0.8660254037844387076, 1.000000000000000000, 0.8660254037844387076, 1.000000000000000000, 0.8660254037844387076, 1.000000000000000000, 0.8660254037844387076, 1.000000000000000000, 0.8660254037844387076, 1.000000000000000000, 0.8660254037844387076, 1.000000000000000000, 0.8660254037844387076, 1.000000000000000000, 0.8660254037844387076, 1.000000000000000000, 0.8660254037844387076, 1.000000000000000000, 0.8660254037844387076, 1.000000000000000000, 0.8660254037844387076, 1.000000000000000000, 0.8660254037844387076, 1.000000000000000000, 0.8660254037844387076, 1.000000000000000000, 0.8660254037844387076, 1.000000000000000000, 0.8660254037844387076, 1.000000000000000000, 0.8660254037844387076, 1.000000000000000000, 0.8660254037844387076, 1.000000000000000000, 0.8660254037844387076, 1.000000000000000000, 0.8660254037844387076, 1.000000000000000000, 0.8660254037844387076, 1.000000000000000000, 0.8660254037844387076, 1.000000000000000000, 0.8660254037844387076, 1.000000000000000000, 0.8660254037844387076, 1.000000000000000000, 0.8660254037844387076, 1.000000000000000000, 0.8660254037844387076, 1.000000000000000000, 0.8660254037844387076, 1.000000000000000000, 0.8660254037844387076, 1.000000000000000000, 0.8660254037844387076, 1.000000000000000000, 0.8660254037844387076, 1.000000000000000000, 0.8660254037844387076, 1.000000000000000000, 0.8660254037844387076, 1.000000000000000000, 0.8660254037844387076, 1.000000000000000000, 0.8660254037844387076, 1.000000000000000000, 0.8660254037844387076, 1.000000000000000000, 0.8660254037844387076, 1.000000000000000000, 0.8660254037844387076, 1.000000000000000000, 0.8660254037844387076, 1.000000000000000000, 0.8660254037844387076, 1.000000000000000000, 0.8660254037844387076, 1.000000000000000000, 0.8660254037844387076, 1.000000000000000000, 0.8660254037844387076, 1.000000000000000000, 0.8660254037844387076, 1.000000000000000000, 0.8660254037844387076, 1.000000000000000000, 0.8660254037844387076, 1.000000000000000000, 0.8660254037844387076, 1.000000000000000000, 0.8660254037844387076, 1.000000000000000000, 0.8660254037844387076, 1.000000000000000000, 0.8660254037844387076, 1.000000000000000000, 0.8660254037844387076, 1.000000000000000000, 0.8660254037844387076, 1.000000000000000000, 0.8660254037844387076, 1.000000000000000000, 0.8660254037844387076, 1.000000000000000000, 0.8660254037844387076, 1.000000000000000000, 0.8660254037844387076, 1.000000000000000000, 0.8660254037844387076, 1.000000000000000000, 0.8660254037844387076, 1.000000000000000000, 0.8660254037844387076, 1.000000000000000000, 0.8660254037844387076, 1.000000000000000000, 0.8660254037844387076, 1.000000000000000000, 0.8660254037844387076, 1.000000000000000000, 0.8660254037844387076, 1.000000000000000000, 0.8660254037844387076, 1.000000000000000000, 0.8660254037844387076, 1.000000000000000000, 0.8660254037844387076, 1.000000000000000000, 0.8660254037844387076, 1.000000000000000000, 0.8660254037844387076, 1.000000000000000000, 0.8660254037844387076, 1.000000000000000000, 0.8660254037844387076, 1.000000000000000000, 0.8660254037844387076, 1.000000000000000000, 0.8660254037844387076, 1.000000000000000000, 0.8660254037844387076, 1.000000000000000000, 0.8660254037844387076, 1.000000000000000000, 0.8660254037844387076, 1.000000000000000000, 0.8660254037844387076, 1.000000000000000000, 0.8660254037844387076, 1.000000000000000000, 0.8660254037844387076, 1.000000000000000000, 0.8660254037844387076, 1.000000000000000000, 0.8660254037844387076, 1.000000000000000000, 0.8660254037844387076, 1.000000000000000000, 0.8660254037844387076, 1.000000000000000000, 0.8660254037844387076, 1.000000000000000000, 0.8660254037844387076, 1.000000000000000000, 0.8660254037844387076, 1.000000000000000000, 0.8660254037844387076, 1.000000000000000000, 0.8660254037844387076, 1.000000000000000000, 0.8660254037844387076, 1.000000000000000000, 0.8660254037844387076, 1.000000000000000000, 0.8660254037844387076, 1.000000000000000000, 0.8660254037844387076, 1.000000000000000000, 0.8660254037844387076, 1.000000000000000000, 0.8660254037844387076, 1.000000000000000000, 0.8660254037844387076, 1.000000000000000000, 0.8660254037844387076, 1.000000000000000000, 0.8660254037844387076, 1.000000000000000000, 0.8660254037844387076, 1.000000000000000000, 0.8660254037844387076, 1.000000000000000000, 0.8660254037844387076, 1.000000000000000000, 0.8660254037844387076, 1.000000000000000000, 0.8660254037844387076, 1.000000000000000000, 0.8660254037844387076, 1.000000000000000000, 0.8660254037844387076, 1.000000000000000000, 0.8660254037844387076, 1.000000000000000000, 0.8660254037844387076, 1.000000000000000000, 0.8660254037844387076, 1.000000000000000000, 0.8660254037844387076, 1.000000000000000000, 0.8660254037844387076, 1.000000000000000000, 0.8660254037844387076, 1.000000000000000000, 0.8660254037844387076, 1.000000000000000000, 0.8660254037844387076, 1.000000000000000000, 0.8660254037844387076, 1.000000000000000000, 0.8660254037844387076, 1.000000000000000000, 0.8660254037844387076, 1.000000000000000000, 0.9548848677736607726, 0.9401542295229587953 ) ) 
 REPRESENTATION_ITEM ( '' )  );
#20251=CARTESIAN_POINT ( 'NONE',  ( 30.65222614765988141, 7.209453229046475009, 160.3254497058415495 ) ) ;
#20252=CARTESIAN_POINT ( 'NONE',  ( 26.99999999999999645, -3.464101615137751278, -2.456249998770948295 ) ) ;
#20256=DIRECTION ( 'NONE',  ( 0.9961946980917462113, 0.000000000000000000, -0.08715574274765118534 ) ) ;
#20264=CARTESIAN_POINT ( 'NONE',  ( 34.02033052368495447, -5.407089921784855591, 163.0045950240894967 ) ) ;
#20265=CARTESIAN_POINT ( 'NONE',  ( 18.12178482187500350, -4.985214923628407568, -7.715624999385467753 ) ) ;
#20267=CARTESIAN_POINT ( 'NONE',  ( 37.52407102436108488, 7.646167579472024665E-16, 167.2340683412427040 ) ) ;
#20268=CARTESIAN_POINT ( 'NONE',  ( 28.12366095802104127, -5.196152422706638241, 165.8449570743377990 ) ) ;
#20279=LINE ( 'NONE', #31818, #26789 ) ;
#20281=CARTESIAN_POINT ( 'NONE',  ( 15.24356964375000167, -3.323476615752272600, -3.365624999385478322 ) ) ;
#20297=CARTESIAN_POINT ( 'NONE',  ( 20.99999999999999645, -6.928203230275506996, -0.3375000000000047962 ) ) ;
#20304=CARTESIAN_POINT ( 'NONE',  ( 31.33857762179763995, -7.209453229046475009, 168.1704829533140071 ) ) ;
#20306=CARTESIAN_POINT ( 'NONE',  ( 26.75643035624999655, 7.049594010296217766E-16, -0.8156249993854780556 ) ) ;
#20307=ADVANCED_FACE ( 'NONE', ( #6063 ), #20494, .T. ) ;
#20314=CARTESIAN_POINT ( 'NONE',  ( 20.00000000000024869, -5.916079783099657874, -7.999999999999998224 ) ) ;
#20320=CARTESIAN_POINT ( 'NONE',  ( 23.87821517812500005, -4.985214923628404016, -8.203124999385469351 ) ) ;
#20325=AXIS2_PLACEMENT_3D ( 'NONE', #17561, #3139, #106 ) ;
#20327=CARTESIAN_POINT ( 'NONE',  ( 31.27484498491342180, 7.209453229046482114, 167.4420155803344699 ) ) ;
#20332=ADVANCED_FACE ( 'NONE', ( #23327 ), #17459, .F. ) ;
#20335=CARTESIAN_POINT ( 'NONE',  ( 37.53224187524366329, 3.604726614523238837, 167.3274615941888044 ) ) ;
#20338=CARTESIAN_POINT ( 'NONE',  ( 26.99999999999940314, 3.464101615138096335, -1.481249998770923781 ) ) ;
#20344=ORIENTED_EDGE ( 'NONE', *, *, #27910, .T. ) ;
#20346=ADVANCED_FACE ( 'NONE', ( #17650 ), #5936, .T. ) ;
#20350=DIRECTION ( 'NONE',  ( 0.08715574274765150453, 0.000000000000000000, 0.9961946980917461003 ) ) ;
#20363=CARTESIAN_POINT ( 'NONE',  ( 30.61300606342344111, 7.209453229046475009, 159.8771620917002565 ) ) ;
#20364=CARTESIAN_POINT ( 'NONE',  ( 23.87821517812500005, -4.985214923628404016, -1.453124999385491112 ) ) ;
#20370=CARTESIAN_POINT ( 'NONE',  ( 15.24356964374999990, 0.000000000000000000, -5.090624999385479299 ) ) ;
#20379=CARTESIAN_POINT ( 'NONE',  ( 24.74941270219456158, -3.464101615137757051, 161.6982627647491881 ) ) ;
#20383=EDGE_CURVE ( 'NONE', #36284, #27062, #15139, .T. ) ;
#20384=CARTESIAN_POINT ( 'NONE',  ( 26.75643035624999655, -3.323476615752267271, -4.565624999385477167 ) ) ;
#20393=CARTESIAN_POINT ( 'NONE',  ( 36.93250142046140638, -3.604726614523238837, 160.4723968279450048 ) ) ;
#20402=CARTESIAN_POINT ( 'NONE',  ( 15.00000000000000000, 0.000000000000000000, -2.643749998770955401 ) ) ;
#20406=CARTESIAN_POINT ( 'NONE',  ( 26.99999999999999645, 7.347880794884117764E-16, -5.624999999999991118 ) ) ;
#20410=CARTESIAN_POINT ( 'NONE',  ( 24.99456971211191814, -3.604726614523240613, 167.2950684582310146 ) ) ;
#20412=CARTESIAN_POINT ( 'NONE',  ( 26.99999999999999645, 7.347880794884117764E-16, -1.068749998770962550 ) ) ;
#20419=CARTESIAN_POINT ( 'NONE',  ( 21.00000000000000000, -6.646953231504538984, -7.228124999385454608 ) ) ;
#20422=CARTESIAN_POINT ( 'NONE',  ( 28.04522078954815356, -5.196152422706638241, 164.9483818460552413 ) ) ;
#20427=CARTESIAN_POINT ( 'NONE',  ( 37.31166038496037629, 3.464101615137755275, 167.6008518709672614 ) ) ;
#20441=CARTESIAN_POINT ( 'NONE',  ( 28.24664800560418243, 5.407089921784862696, 168.6480295846443482 ) ) ;
#20442=CARTESIAN_POINT ( 'NONE',  ( 26.99999999999999645, 3.464101615137755275, -1.481249998770931109 ) ) ;
#20452=CARTESIAN_POINT ( 'NONE',  ( 27.62402916835064559, 5.407089921784856479, 161.5314637101514279 ) ) ;
#20453=CARTESIAN_POINT ( 'NONE',  ( 21.00000000000000000, 6.646953231504538984, -8.353124999385492799 ) ) ;
#20455=CARTESIAN_POINT ( 'NONE',  ( 34.25074851857407765, -5.407089921784861808, 165.6382847571695436 ) ) ;
#20456=CARTESIAN_POINT ( 'NONE',  ( 25.04683167421379508, 3.464101615137757051, 165.0977771707628960 ) ) ;
#20457=FACE_OUTER_BOUND ( 'NONE', #15834, .T. ) ;
#20462=CIRCLE ( 'NONE', #4105, 4.000000000000000888 ) ;
#20469=CARTESIAN_POINT ( 'NONE',  ( 15.24356964374999990, 0.000000000000000000, -5.203124999385494220 ) ) ;
#20479=( BOUNDED_CURVE ( )  B_SPLINE_CURVE ( 2, ( #29279, #17555, #26250, #23238, #34786, #9014, #12038 ),
 .UNSPECIFIED., .F., .F. ) 
 B_SPLINE_CURVE_WITH_KNOTS ( ( 3, 2, 2, 3 ),
 ( 0.6956521739130446802, 0.7028985507246381381, 0.7101449275362315960, 0.7173913043478249429 ),
 .UNSPECIFIED. ) 
 CURVE ( )  GEOMETRIC_REPRESENTATION_ITEM ( )  RATIONAL_B_SPLINE_CURVE ( ( 0.9999999999999774625, 0.8660254037844612451, 1.000000000000000000, 0.8660254037844387076, 1.000000000000000000, 0.8660254037844592467, 0.9999999999999794609 ) ) 
 REPRESENTATION_ITEM ( '' )  );
#20481=CARTESIAN_POINT ( 'NONE',  ( 25.00000000000004263, 0.000000000000000000, 49.82535622836640954 ) ) ;
#20492=CARTESIAN_POINT ( 'NONE',  ( 34.45175145028584041, -5.407089921784855591, 167.9357587796436064 ) ) ;
#20494=CYLINDRICAL_SURFACE ( 'NONE', #34529, 5.999999999999994671 ) ;
#20495=CARTESIAN_POINT ( 'NONE',  ( 20.99999999999999645, 0.000000000000000000, -8.000000000000000000 ) ) ;
#20496=CARTESIAN_POINT ( 'NONE',  ( 26.99999999999981171, 3.464101615137862300, -3.787500000000012523 ) ) ;
#20500=CARTESIAN_POINT ( 'NONE',  ( 37.22341519532091070, 3.464101615137966217, 166.5922047379251012 ) ) ;
#20504=VERTEX_POINT ( 'NONE', #20314 ) ;
#20509=CARTESIAN_POINT ( 'NONE',  ( 21.00000000000000000, -6.646953231504538984, -9.590624999385488181 ) ) ;
#20516=CARTESIAN_POINT ( 'NONE',  ( 37.44889919624123564, 3.604726614523243278, 166.3748504141385922 ) ) ;
#20519=EDGE_CURVE ( 'NONE', #33723, #23833, #17656, .T. ) ;
#20520=DIRECTION ( 'NONE',  ( 0.08715574274765150453, 0.000000000000000000, 0.9961946980917461003 ) ) ;
#20523=CARTESIAN_POINT ( 'NONE',  ( 31.39740774815230751, 7.209453229046475009, 168.8429143745260035 ) ) ;
#20530=VERTEX_POINT ( 'NONE', #8926 ) ;
#20536=DIRECTION ( 'NONE',  ( 0.9961946980917462113, 0.000000000000000000, -0.08715574274765118534 ) ) ;
#20538=CARTESIAN_POINT ( 'NONE',  ( 15.00000000000000000, 0.000000000000000000, -2.250000000000001776 ) ) ;
#20542=ORIENTED_EDGE ( 'NONE', *, *, #19180, .F. ) ;
#20547=CARTESIAN_POINT ( 'NONE',  ( 33.75886329544200493, 5.407089921784857367, 160.0160109298142288 ) ) ;
#20548=CARTESIAN_POINT ( 'NONE',  ( 23.87821517812500005, -4.985214923628404016, -2.353124999385475036 ) ) ;
#20553=CARTESIAN_POINT ( 'NONE',  ( 20.99999999999999645, 6.646953231504538984, -5.203124999385457805 ) ) ;
#20562=CARTESIAN_POINT ( 'NONE',  ( 36.88023945835949746, 3.464101615137755275, 162.6696881154131518 ) ) ;
#20566=CARTESIAN_POINT ( 'NONE',  ( 18.12178482187499640, 4.985214923628404904, -4.828124999385480010 ) ) ;
#20567=CARTESIAN_POINT ( 'NONE',  ( 27.00000000000041567, 3.464101615137513690, -0.6375000000000179412 ) ) ;
#20575=CARTESIAN_POINT ( 'NONE',  ( 24.36214585379926589, -3.604726614523244610, 160.0664306802028136 ) ) ;
#20584=CARTESIAN_POINT ( 'NONE',  ( 18.00000000000000000, 5.196152422706630247, -3.618749998770959486 ) ) ;
#20589=CARTESIAN_POINT ( 'NONE',  ( 26.99999999999999645, 3.464101615137755275, -7.837500000000007461 ) ) ;
#20594=CARTESIAN_POINT ( 'NONE',  ( 24.91612954363903043, -3.604726614523240613, 166.3984932299484569 ) ) ;
#20601=LINE ( 'NONE', #26453, #13384 ) ;
#20604=CARTESIAN_POINT ( 'NONE',  ( 15.24356964374999990, 3.323476615752268604, -5.578124999385491556 ) ) ;
#20608=ADVANCED_FACE ( 'NONE', ( #12507 ), #934, .T. ) ;
#20612=CARTESIAN_POINT ( 'NONE',  ( 33.70166733926387082, -5.407089921784861808, 159.3622581591915548 ) ) ;
#20625=CARTESIAN_POINT ( 'NONE',  ( 31.41211527974097706, -7.209453229046482114, 169.0110222298289671 ) ) ;
#20626=CARTESIAN_POINT ( 'NONE',  ( 23.99999999999999645, 5.196152422706631135, -1.443749998770949006 ) ) ;
#20634=CARTESIAN_POINT ( 'NONE',  ( 36.95541128647934670, 7.347880794884117764E-16, 163.5289060425172636 ) ) ;
#20635=DIRECTION ( 'NONE',  ( 1.000000000000000000, 0.000000000000000000, 0.000000000000000000 ) ) ;
#20636=VERTEX_POINT ( 'NONE', #12688 ) ;
#20637=CARTESIAN_POINT ( 'NONE',  ( 33.74578993402985816, -5.407089921784855591, 159.8665817251004739 ) ) ;
#20638=CARTESIAN_POINT ( 'NONE',  ( 23.87821517812499650, 4.985214923628404904, -7.940624999385470062 ) ) ;
#20639=CARTESIAN_POINT ( 'NONE',  ( 31.11796464796764994, 7.209453229046482114, 165.6488651237693261 ) ) ;
#20640=CARTESIAN_POINT ( 'NONE',  ( 24.96839150574091093, 3.464101615137757051, 164.2012019424803100 ) ) ;
#20652=CARTESIAN_POINT ( 'NONE',  ( 21.00000000000000000, -6.646953231504538984, -4.190624999385508254 ) ) ;
#20660=CARTESIAN_POINT ( 'NONE',  ( 36.87697111800645899, 7.347880794884117764E-16, 162.6323308142347059 ) ) ;
#20674=ORIENTED_EDGE ( 'NONE', *, *, #33601, .F. ) ;
#20675=CARTESIAN_POINT ( 'NONE',  ( 24.99130137175887612, 0.000000000000000000, 167.2577111570525972 ) ) ;
#20677=CARTESIAN_POINT ( 'NONE',  ( 15.24356964374999990, 3.323476615752268604, -1.528124999385498173 ) ) ;
#20679=( BOUNDED_CURVE ( )  B_SPLINE_CURVE ( 2, ( #5273, #36359, #7569, #11153, #7941, #22350, #1869 ),
 .UNSPECIFIED., .F., .F. ) 
 B_SPLINE_CURVE_WITH_KNOTS ( ( 3, 2, 2, 3 ),
 ( 0.2608695652173908530, 0.2681159420289850326, 0.2753623188405791011, 0.2826086956521732252 ),
 .UNSPECIFIED. ) 
 CURVE ( )  GEOMETRIC_REPRESENTATION_ITEM ( )  RATIONAL_B_SPLINE_CURVE ( ( 1.000000000000008216, 0.8660254037844304920, 1.000000000000000000, 0.8660254037844387076, 1.000000000000000000, 0.8660254037844510311, 0.9999999999999876765 ) ) 
 REPRESENTATION_ITEM ( '' )  );
#20680=CARTESIAN_POINT ( 'NONE',  ( 20.99999999999999645, -6.928203230275506996, -4.781249998770952914 ) ) ;
#20690=CARTESIAN_POINT ( 'NONE',  ( 23.87821517812500005, -4.985214923628404016, -9.553124999385486760 ) ) ;
#20697=CARTESIAN_POINT ( 'NONE',  ( 37.44563085588819717, 7.646167579472024665E-16, 166.3374931129601464 ) ) ;
#20705=CARTESIAN_POINT ( 'NONE',  ( 25.14491336835161306, 3.604726614523236616, 169.0135043124392951 ) ) ;
#20719=DIRECTION ( 'NONE',  ( 0.08715574274765150453, 0.000000000000000000, 0.9961946980917461003 ) ) ;
#20722=CARTESIAN_POINT ( 'NONE',  ( 37.38683221308021842, 7.347880794884117764E-16, 168.4600697980714017 ) ) ;
#20732=CARTESIAN_POINT ( 'NONE',  ( 24.43895185209563792, 3.604726614523236616, 160.9443272578961626 ) ) ;
#20733=CARTESIAN_POINT ( 'NONE',  ( 23.87821517812500005, -4.985214923628404016, -3.253124999385486937 ) ) ;
#20739=CARTESIAN_POINT ( 'NONE',  ( 26.75643035624999655, 7.049594010296217766E-16, -4.415624999385469707 ) ) ;
#20748=CARTESIAN_POINT ( 'NONE',  ( 33.69882328325508070, 5.196152422706631135, 160.7270745741280962 ) ) ;
#20752=CARTESIAN_POINT ( 'NONE',  ( 26.75643035624999655, -3.323476615752267271, -6.815624999385487826 ) ) ;
#20753=CARTESIAN_POINT ( 'NONE',  ( 15.00000000000010658, 3.464101615137812562, -2.287500000000008527 ) ) ;
#20756=EDGE_CURVE ( 'NONE', #13615, #33723, #24399, .T. ) ;
#20762=CARTESIAN_POINT ( 'NONE',  ( 27.57990657358465114, 5.407089921784862696, 161.0271401442424803 ) ) ;
#20774=ORIENTED_EDGE ( 'NONE', *, *, #35891, .T. ) ;
#20775=CARTESIAN_POINT ( 'NONE',  ( 21.00000000000000000, -6.928203230275506996, -7.987499999999996270 ) ) ;
#20779=CARTESIAN_POINT ( 'NONE',  ( 27.00000000000015632, 3.464101615137663348, -6.881249998770978316 ) ) ;
#20781=CARTESIAN_POINT ( 'NONE',  ( 37.52897353489062482, 7.646167579472015790E-16, 167.2901042930103586 ) ) ;
#20788=CARTESIAN_POINT ( 'NONE',  ( 24.58926402489574770, 0.000000000000000000, 159.8677550070055702 ) ) ;
#20790=CARTESIAN_POINT ( 'NONE',  ( 21.00000000000000000, -6.646953231504538984, -6.328124999385495997 ) ) ;
#20799=CARTESIAN_POINT ( 'NONE',  ( 33.75396078491245078, 5.407089921784862696, 159.9599749780466027 ) ) ;
#20813=CARTESIAN_POINT ( 'NONE',  ( 24.39973617568989184, 4.660121730947068386, -8.000000000000026645 ) ) ;
#20814=CARTESIAN_POINT ( 'NONE',  ( 37.48811928047766884, 3.604726614523243278, 166.8231380282798568 ) ) ;
#20815=CARTESIAN_POINT ( 'NONE',  ( 18.00000000000000355, -5.196152422706632912, -2.568749998770964105 ) ) ;
#20825=ORIENTED_EDGE ( 'NONE', *, *, #22396, .F. ) ;
#20826=CARTESIAN_POINT ( 'NONE',  ( 24.40626844856526745, -3.604726614523240613, 160.5707542461117612 ) ) ;
#20827=CARTESIAN_POINT ( 'NONE',  ( 18.12178482187500350, -4.985214923628407568, -9.515624999385464022 ) ) ;
#20829=CARTESIAN_POINT ( 'NONE',  ( 24.82951852428355011, 0.000000000000000000, 165.4085247487197989 ) ) ;
#20830=CARTESIAN_POINT ( 'NONE',  ( 28.08444087378459741, -5.196152422706638241, 165.3966694601965060 ) ) ;
#20831=CARTESIAN_POINT ( 'NONE',  ( 26.99999999999999645, 7.347880794884117764E-16, -6.918749998770956644 ) ) ;
#20836=ORIENTED_EDGE ( 'NONE', *, *, #35764, .T. ) ;
#20841=CARTESIAN_POINT ( 'NONE',  ( 18.12178482187500350, -4.985214923628407568, -3.778124999385484628 ) ) ;
#20844=AXIS2_PLACEMENT_3D ( 'NONE', #13171, #31900, #8235 ) ;
#20852=EDGE_CURVE ( 'NONE', #17354, #25471, #25543, .T. ) ;
#20856=EDGE_CURVE ( 'NONE', #4359, #6022, #8824, .T. ) ;
#20859=CARTESIAN_POINT ( 'NONE',  ( 37.21194452064604974, -3.604726614523235284, 163.6664460787016253 ) ) ;
#20864=CARTESIAN_POINT ( 'NONE',  ( 15.00000000000000000, 0.000000000000000000, -5.793749998770941545 ) ) ;
#20871=CARTESIAN_POINT ( 'NONE',  ( 37.37536153829788077, 3.604726614523238837, 165.5343111376236607 ) ) ;
#20872=CARTESIAN_POINT ( 'NONE',  ( 26.75643035624999655, -3.323476615752267715, -2.203124999385475569 ) ) ;
#20874=CARTESIAN_POINT ( 'NONE',  ( 18.00000000000000000, 5.196152422706630247, -3.675000000000011369 ) ) ;
#20876=CARTESIAN_POINT ( 'NONE',  ( 37.05999817766988258, -3.464101615137495926, 164.7243396790029522 ) ) ;
#20880=ORIENTED_EDGE ( 'NONE', *, *, #15675, .T. ) ;
#20883=CARTESIAN_POINT ( 'NONE',  ( 26.75643035624999655, 7.049594010296217766E-16, -1.715624999385462202 ) ) ;
#20885=CARTESIAN_POINT ( 'NONE',  ( 15.00000000000000178, -3.464101615137757051, -7.556249998770954157 ) ) ;
#20886=ORIENTED_EDGE ( 'NONE', *, *, #31697, .T. ) ;
#20889=CARTESIAN_POINT ( 'NONE',  ( 34.14616162727688931, 5.407089921784862696, 164.4428511194594478 ) ) ;
#20895=CARTESIAN_POINT ( 'NONE',  ( 37.03058311459962937, -3.464101615137506140, 164.3881239696213754 ) ) ;
#20896=CARTESIAN_POINT ( 'NONE',  ( 31.26013745332475224, -7.209453229046475009, 167.2739077250314779 ) ) ;
#20903=( BOUNDED_CURVE ( )  B_SPLINE_CURVE ( 2, ( #36967, #1544, #7617, #13116, #31656, #2655, #26335 ),
 .UNSPECIFIED., .F., .F. ) 
 B_SPLINE_CURVE_WITH_KNOTS ( ( 3, 2, 2, 3 ),
 ( 0.1956521739130434034, 0.2028985507246377218, 0.2101449275362319846, 0.2173913043478263030 ),
 .UNSPECIFIED. ) 
 CURVE ( )  GEOMETRIC_REPRESENTATION_ITEM ( )  RATIONAL_B_SPLINE_CURVE ( ( 1.000000000000001554, 0.8660254037844372643, 1.000000000000000000, 0.8660254037844387076, 1.000000000000000000, 0.8660254037844345998, 1.000000000000003997 ) ) 
 REPRESENTATION_ITEM ( '' )  );
#20908=EDGE_LOOP ( 'NONE', ( #31354, #20836, #30971, #14767 ) ) ;
#20917=CARTESIAN_POINT ( 'NONE',  ( 30.65467740297821919, -6.928203230275506996, 160.3534676823375378 ) ) ;
#20921=VERTEX_POINT ( 'NONE', #2429 ) ;
#20926=CARTESIAN_POINT ( 'NONE',  ( 21.00000000000000000, 6.646953231504538984, -4.865624999385484983 ) ) ;
#20934=ORIENTED_EDGE ( 'NONE', *, *, #35322, .T. ) ;
#20935=CARTESIAN_POINT ( 'NONE',  ( 15.24356964375000167, -3.323476615752272600, -5.053124999385469884 ) ) ;
#20943=CARTESIAN_POINT ( 'NONE',  ( 36.67760235647121903, -3.464101615137751278, 160.3535354423498234 ) ) ;
#20947=CARTESIAN_POINT ( 'NONE',  ( 15.24356964374999990, 0.000000000000000000, -7.903124999385474858 ) ) ;
#20955=VECTOR ( 'NONE', #33036, 1000.000000000000000 ) ;
#20957=CARTESIAN_POINT ( 'NONE',  ( 27.47531968228746990, -5.407089921784865361, 159.8317065065323845 ) ) ;
#20961=CARTESIAN_POINT ( 'NONE',  ( 20.99999999999999645, -6.928203230275506996, -2.081249998770946963 ) ) ;
#20963=CARTESIAN_POINT ( 'NONE',  ( 34.35575969410840003, 5.196152422706637353, 168.2358921097703046 ) ) ;
#20969=CARTESIAN_POINT ( 'NONE',  ( 18.00000000000000355, -5.196152422706632912, -6.225000000000008527 ) ) ;
#20970=( BOUNDED_CURVE ( )  B_SPLINE_CURVE ( 2, ( #23330, #18402, #20874, #3609, #29379, #20496, #32413 ),
 .UNSPECIFIED., .F., .F. ) 
 B_SPLINE_CURVE_WITH_KNOTS ( ( 3, 2, 2, 3 ),
 ( 0.3478260869565210078, 0.3550724637681153539, 0.3623188405797096445, 0.3695652173913039351 ),
 .UNSPECIFIED. ) 
 CURVE ( )  GEOMETRIC_REPRESENTATION_ITEM ( )  RATIONAL_B_SPLINE_CURVE ( ( 1.000000000000013323, 0.8660254037844252739, 1.000000000000000000, 0.8660254037844387076, 1.000000000000000000, 0.8660254037844459241, 0.9999999999999927836 ) ) 
 REPRESENTATION_ITEM ( '' )  );
#20974=CARTESIAN_POINT ( 'NONE',  ( 24.94881294716939379, 3.604726614523236616, 166.7720662417328299 ) ) ;
#20979=ORIENTED_EDGE ( 'NONE', *, *, #16382, .T. ) ;
#20983=CARTESIAN_POINT ( 'NONE',  ( 27.77068019989305370, -5.196152422706638241, 161.8103685470662469 ) ) ;
#20984=CARTESIAN_POINT ( 'NONE',  ( 18.12178482187499640, 4.985214923628404904, -6.965624999385466865 ) ) ;
#20988=CARTESIAN_POINT ( 'NONE',  ( 37.14170668649535401, 7.347880794884125653E-16, 165.6582722084640125 ) ) ;
#20991=CARTESIAN_POINT ( 'NONE',  ( 33.71474070067601048, 5.407089921784862696, 159.5116873639053097 ) ) ;
#21000=AXIS2_PLACEMENT_3D ( 'NONE', #5621, #19874, #14171 ) ;
#21004=CARTESIAN_POINT ( 'NONE',  ( 24.00000000000000000, -5.196152422706629359, -6.149999999999988809 ) ) ;
#21006=CARTESIAN_POINT ( 'NONE',  ( 37.37045902776835504, 3.604726614523243278, 165.4782751858559777 ) ) ;
#21017=CARTESIAN_POINT ( 'NONE',  ( 36.82628035898768815, 3.604726614523238837, 159.2582845396456719 ) ) ;
#21018=CARTESIAN_POINT ( 'NONE',  ( 26.75643035624999655, -3.323476615752267715, -9.403124999385470417 ) ) ;
#21020=CARTESIAN_POINT ( 'NONE',  ( 24.86873860851999041, 0.000000000000000000, 165.8568123628610920 ) ) ;
#21022=CARTESIAN_POINT ( 'NONE',  ( 27.95370725966311554, 5.196152422706636465, 163.9023774130589288 ) ) ;
#21028=ORIENTED_EDGE ( 'NONE', *, *, #1566, .T. ) ;
#21032=CARTESIAN_POINT ( 'NONE',  ( 18.12178482187499640, 4.985214923628404904, -3.478124999385490135 ) ) ;
#21047=CARTESIAN_POINT ( 'NONE',  ( 31.02481694790609268, -7.209453229046475009, 164.5841820401837765 ) ) ;
#21052=CARTESIAN_POINT ( 'NONE',  ( 26.99999999999999645, 7.347880794884117764E-16, -7.368749998770962151 ) ) ;
#21053=CARTESIAN_POINT ( 'NONE',  ( 29.48995970988985604, 6.148715791637016537, 159.4803054849043917 ) ) ;
#21055=CARTESIAN_POINT ( 'NONE',  ( 20.99999999999999645, 6.928203230275506996, -2.306249998770960818 ) ) ;
#21060=CARTESIAN_POINT ( 'NONE',  ( 34.42560472746153977, 5.407089921784857367, 167.6369003702161251 ) ) ;
#21061=CARTESIAN_POINT ( 'NONE',  ( 21.00000000000000000, -6.646953231504538984, -2.728124999385465266 ) ) ;
#21064=CARTESIAN_POINT ( 'NONE',  ( 24.90302469878729141, 0.000000000000000000, 163.4540559201358576 ) ) ;
#21066=CARTESIAN_POINT ( 'NONE',  ( 26.99999999999999645, 7.347880794884117764E-16, -7.368749998770962151 ) ) ;
#21067=CYLINDRICAL_SURFACE ( 'NONE', #11524, 6.000000000000001776 ) ;
#21074=ADVANCED_FACE ( 'NONE', ( #26110 ), #2243, .T. ) ;
#21075=CARTESIAN_POINT ( 'NONE',  ( 15.24356964374999990, 0.000000000000000000, -0.5906249993854750802 ) ) ;
#21078=CARTESIAN_POINT ( 'NONE',  ( 15.00000000000000000, 3.464101615137752166, -8.081249998770942966 ) ) ;
#21082=VECTOR ( 'NONE', #8080, 1000.000000000000000 ) ;
#21084=CARTESIAN_POINT ( 'NONE',  ( 24.82625018393050809, 3.604726614523240613, 165.3711674475413531 ) ) ;
#21089=CARTESIAN_POINT ( 'NONE',  ( 25.06974154023176382, 0.000000000000000000, 168.1542863853351548 ) ) ;
#21099=AXIS2_PLACEMENT_3D ( 'NONE', #29461, #17358, #26238 ) ;
#21108=CARTESIAN_POINT ( 'NONE',  ( 15.09967099808794266, 0.4797207149645432156, -8.000000000000000000 ) ) ;
#21117=CARTESIAN_POINT ( 'NONE',  ( 15.24356964374999990, 3.323476615752268604, -4.790624999385491023 ) ) ;
#21122=CARTESIAN_POINT ( 'NONE',  ( 18.12178482187499640, 4.985214923628404904, -5.165624999385470595 ) ) ;
#21129=CARTESIAN_POINT ( 'NONE',  ( 24.70692427760507570, 0.000000000000000000, 161.2126178494294493 ) ) ;
#21134=CARTESIAN_POINT ( 'NONE',  ( 23.87821517812500005, -4.985214923628404016, -6.403124999385473082 ) ) ;
#21135=CARTESIAN_POINT ( 'NONE',  ( 20.99999999999999645, 6.928203230275506996, -2.362500000000002043 ) ) ;
#21141=CARTESIAN_POINT ( 'NONE',  ( 36.75931086529713099, 7.347880794884117764E-16, 161.2874679718108553 ) ) ;
#21142=CARTESIAN_POINT ( 'NONE',  ( 24.39482925732963281, 3.604726614523240613, 160.4400036919872150 ) ) ;
#21145=CARTESIAN_POINT ( 'NONE',  ( 15.00000000000000000, 0.000000000000000000, -3.993749998770945719 ) ) ;
#21155=CARTESIAN_POINT ( 'NONE',  ( 21.00000000000000000, -6.928203230275506996, -7.087500000000004796 ) ) ;
#21156=CARTESIAN_POINT ( 'NONE',  ( 14.99999999999979039, -3.464101615137634038, -4.462499999999995026 ) ) ;
#21159=CARTESIAN_POINT ( 'NONE',  ( 34.22950430627932406, 5.407089921784857367, 165.3954622995096599 ) ) ;
#21163=VERTEX_POINT ( 'NONE', #25741 ) ;
#21169=CARTESIAN_POINT ( 'NONE',  ( 15.24356964374999990, 0.000000000000000000, -9.140624999385476457 ) ) ;
#21173=CARTESIAN_POINT ( 'NONE',  ( 26.99999999999999645, 7.347880794884117764E-16, -6.018749998770944742 ) ) ;
#21177=CARTESIAN_POINT ( 'NONE',  ( 25.14161354455898945, -3.464101615137757051, 166.1811389061620048 ) ) ;
#21183=CARTESIAN_POINT ( 'NONE',  ( 27.79682692271734012, 5.196152422706636465, 162.1092269564937851 ) ) ;
#21187=VERTEX_POINT ( 'NONE', #24029 ) ;
#21189=CARTESIAN_POINT ( 'NONE',  ( 18.00000000000000000, 5.196152422706630247, -7.725000000000009415 ) ) ;
#21192=CARTESIAN_POINT ( 'NONE',  ( 24.95044711734591658, -3.604726614523244610, 166.7907448923220954 ) ) ;
#21194=( BOUNDED_CURVE ( )  B_SPLINE_CURVE ( 2, ( #35959, #9627, #6780, #21204, #35389, #9813, #33124 ),
 .UNSPECIFIED., .F., .F. ) 
 B_SPLINE_CURVE_WITH_KNOTS ( ( 3, 2, 2, 3 ),
 ( 0.5217391304347814840, 0.5289855072463758301, 0.5362318840579701762, 0.5434782608695644113 ),
 .UNSPECIFIED. ) 
 CURVE ( )  GEOMETRIC_REPRESENTATION_ITEM ( )  RATIONAL_B_SPLINE_CURVE ( ( 1.000000000000020428, 0.8660254037844181685, 1.000000000000000000, 0.8660254037844387076, 1.000000000000000000, 0.8660254037844530295, 0.9999999999999856781 ) ) 
 REPRESENTATION_ITEM ( '' )  );
#21204=CARTESIAN_POINT ( 'NONE',  ( 20.99999999999999645, 6.928203230275506996, -5.512500000000003730 ) ) ;
#21205=CARTESIAN_POINT ( 'NONE',  ( 27.55866236128991176, -5.407089921784859143, 160.7843176865825967 ) ) ;
#21206=CARTESIAN_POINT ( 'NONE',  ( 15.00000000000000000, 0.000000000000000000, -0.9000000000000119016 ) ) ;
#21208=CARTESIAN_POINT ( 'NONE',  ( 34.36556471527461554, 5.196152422706631135, 168.3479640145299641 ) ) ;
#21209=CARTESIAN_POINT ( 'NONE',  ( 34.22460179574976991, 5.407089921784862696, 165.3394263477420054 ) ) ;
#21210=CARTESIAN_POINT ( 'NONE',  ( 33.98970557456826214, -5.196152422706635576, 164.0518743777849409 ) ) ;
#21215=ORIENTED_EDGE ( 'NONE', *, *, #12154, .T. ) ;
#21216=ORIENTED_EDGE ( 'NONE', *, *, #4481, .F. ) ;
#21221=CARTESIAN_POINT ( 'NONE',  ( 21.00000000000000000, -6.646953231504538984, -7.790624999385473259 ) ) ;
#21228=FACE_OUTER_BOUND ( 'NONE', #22029, .T. ) ;
#21232=MANIFOLD_SOLID_BREP ( 'Thread1', #14427 ) ;
#21235=CARTESIAN_POINT ( 'NONE',  ( 20.99999999999999645, 6.928203230275506996, -1.856249998770964638 ) ) ;
#21236=CARTESIAN_POINT ( 'NONE',  ( 31.00520690578787253, 7.209453229046475009, 164.3600382331131300 ) ) ;
#21243=CARTESIAN_POINT ( 'NONE',  ( 20.99999999999999645, -6.928203230275506996, -4.331249998770957177 ) ) ;
#21249=CARTESIAN_POINT ( 'NONE',  ( 28.13389026342440857, 5.407089921784856479, 167.3592026939881237 ) ) ;
#21250=CARTESIAN_POINT ( 'NONE',  ( 23.87821517812500005, -4.985214923628404016, -1.790624999385481697 ) ) ;
#21262=CARTESIAN_POINT ( 'NONE',  ( 23.87821517812500005, -4.985214923628404016, -0.4406249993854638447 ) ) ;
#21264=CARTESIAN_POINT ( 'NONE',  ( 15.00000000000000000, 3.464101615137752166, -7.181249998770951493 ) ) ;
#21265=( BOUNDED_CURVE ( )  B_SPLINE_CURVE ( 2, ( #13803, #22332, #5068, #18938, #4882, #21777, #2038 ),
 .UNSPECIFIED., .F., .F. ) 
 B_SPLINE_CURVE_WITH_KNOTS ( ( 3, 2, 2, 3 ),
 ( 0.08695652173913158423, 0.09420289855072500051, 0.1014492753623184029, 0.1086956521739118053 ),
 .UNSPECIFIED. ) 
 CURVE ( )  GEOMETRIC_REPRESENTATION_ITEM ( )  RATIONAL_B_SPLINE_CURVE ( ( 0.9999999999999786837, 0.8660254037844600239, 1.000000000000000000, 0.8660254037844387076, 1.000000000000000000, 0.8660254037844615782, 0.9999999999999771294 ) ) 
 REPRESENTATION_ITEM ( '' )  );
#21271=CARTESIAN_POINT ( 'NONE',  ( 30.96108431102187808, 7.209453229046482114, 163.8557146672041824 ) ) ;
#21272=AXIS2_PLACEMENT_3D ( 'NONE', #33004, #9699, #32435 ) ;
#21279=CARTESIAN_POINT ( 'NONE',  ( 37.44726502606470575, -3.604726614523235284, 166.3561717635493835 ) ) ;
#21292=CARTESIAN_POINT ( 'NONE',  ( 37.26917196037089042, 7.347880794884117764E-16, 167.1152069556475510 ) ) ;
#21299=CARTESIAN_POINT ( 'NONE',  ( 36.78872592836736288, 7.347880794884125653E-16, 161.6236836811924604 ) ) ;
#21307=CARTESIAN_POINT ( 'NONE',  ( 15.24356964374999990, 0.000000000000000000, -4.303124999385482319 ) ) ;
#21309=ORIENTED_EDGE ( 'NONE', *, *, #6809, .F. ) ;
#21316=CARTESIAN_POINT ( 'NONE',  ( 36.55994210376188391, -3.464101615137751278, 159.0086725999259727 ) ) ;
#21321=CARTESIAN_POINT ( 'NONE',  ( 15.24356964375000167, -3.323476615752272600, -6.965624999385507721 ) ) ;
#21326=CARTESIAN_POINT ( 'NONE',  ( 25.02068495149662297, 0.000000000000000000, 164.7989187625597367 ) ) ;
#21336=CARTESIAN_POINT ( 'NONE',  ( 18.00000000000000355, -5.196152422706632912, -2.118749998770957710 ) ) ;
#21343=EDGE_LOOP ( 'NONE', ( #34789, #17742, #7991, #30603 ) ) ;
#21344=CARTESIAN_POINT ( 'NONE',  ( 18.00000000000000000, 5.196152422706630247, -6.374999999999992006 ) ) ;
#21348=CARTESIAN_POINT ( 'NONE',  ( 24.83768937516614272, -3.604726614523240613, 165.5019180016658993 ) ) ;
#21351=ORIENTED_EDGE ( 'NONE', *, *, #35567, .T. ) ;
#21354=CARTESIAN_POINT ( 'NONE',  ( 20.99999999999999645, -6.646953231504538984, -1.378124999385478056 ) ) ;
#21355=CARTESIAN_POINT ( 'NONE',  ( 15.00000000000045297, -3.464101615138017287, -1.312499999999984457 ) ) ;
#21357=CARTESIAN_POINT ( 'NONE',  ( 21.00000000000000000, -6.646953231504538984, -9.478124999385466154 ) ) ;
#21360=( BOUNDED_CURVE ( )  B_SPLINE_CURVE ( 3, ( #2193, #22121, #33669, #36691 ),
 .UNSPECIFIED., .F., .F. ) 
 B_SPLINE_CURVE_WITH_KNOTS ( ( 4, 4 ),
 ( 0.000000000000000000, 1.570796326794937414 ),
 .UNSPECIFIED. ) 
 CURVE ( )  GEOMETRIC_REPRESENTATION_ITEM ( )  RATIONAL_B_SPLINE_CURVE ( ( 1.000000000000000000, 0.8047378541243555006, 0.8047378541243555006, 1.000000000000000000 ) ) 
 REPRESENTATION_ITEM ( '' )  );
#21365=CARTESIAN_POINT ( 'NONE',  ( 37.26917196037089042, 7.347880794884117764E-16, 167.1152069556475510 ) ) ;
#21370=CARTESIAN_POINT ( 'NONE',  ( 33.76745843056175289, 5.196152422706637353, 161.5115778976509944 ) ) ;
#21376=CARTESIAN_POINT ( 'NONE',  ( 23.99999999999999645, 5.196152422706631135, -7.800000000000001599 ) ) ;
#21378=CARTESIAN_POINT ( 'NONE',  ( 28.43742163191258499, -5.196152422706638241, 169.4312579874681148 ) ) ;
#21379=CARTESIAN_POINT ( 'NONE',  ( 28.05054758442196672, 5.407089921784862696, 166.4065915139379115 ) ) ;
#21392=CARTESIAN_POINT ( 'NONE',  ( 15.00000000000000000, 0.000000000000000000, 0.000000000000000000 ) ) ;
#21394=CARTESIAN_POINT ( 'NONE',  ( 24.55497793462844669, 0.000000000000000000, 162.2705114497308045 ) ) ;
#21395=CARTESIAN_POINT ( 'NONE',  ( 30.80175271875776843, -6.928203230275514990, 162.0345462341430505 ) ) ;
#21407=CARTESIAN_POINT ( 'NONE',  ( 26.75643035624999655, 7.049594010296217766E-16, -6.778124999385487293 ) ) ;
#21416=CARTESIAN_POINT ( 'NONE',  ( 25.21678537267883868, 0.000000000000000000, 167.0403568332661450 ) ) ;
#21420=ADVANCED_FACE ( 'NONE', ( #16527 ), #2108, .T. ) ;
#21422=CARTESIAN_POINT ( 'NONE',  ( 24.71349244175073778, 3.604726614523236616, 164.0823405568851570 ) ) ;
#21433=ORIENTED_EDGE ( 'NONE', *, *, #17603, .F. ) ;
#21434=CARTESIAN_POINT ( 'NONE',  ( 28.10774354060011504, -5.407089921784859143, 167.0603442845606139 ) ) ;
#21435=CARTESIAN_POINT ( 'NONE',  ( 18.12178482187500350, -4.985214923628407568, -2.765624999385457805 ) ) ;
#21437=CYLINDRICAL_SURFACE ( 'NONE', #11835, 6.000000000000001776 ) ;
#21449=CARTESIAN_POINT ( 'NONE',  ( 26.75643035624999655, 3.323476615752271712, -1.228124999385458160 ) ) ;
#21452=CARTESIAN_POINT ( 'NONE',  ( 18.00000000000000000, 5.196152422706630247, -9.468749998770952914 ) ) ;
#21459=CARTESIAN_POINT ( 'NONE',  ( 30.92186422678543778, 7.209453229046482114, 163.4074270530628894 ) ) ;
#21463=EDGE_CURVE ( 'NONE', #27062, #35303, #13870, .T. ) ;
#21467=CARTESIAN_POINT ( 'NONE',  ( 24.91612954363903043, -3.604726614523240613, 166.3984932299484569 ) ) ;
#21468=ORIENTED_EDGE ( 'NONE', *, *, #33807, .F. ) ;
#21469=CARTESIAN_POINT ( 'NONE',  ( 26.99999999999936051, -3.464101615138118984, -5.212500000000003020 ) ) ;
#21487=CARTESIAN_POINT ( 'NONE',  ( 28.32508817407707014, 5.407089921784862696, 169.5446048129269059 ) ) ;
#21496=CARTESIAN_POINT ( 'NONE',  ( 18.12178482187499640, 4.985214923628404904, -3.928124999385496086 ) ) ;
#21499=CARTESIAN_POINT ( 'NONE',  ( 20.99999999999999645, 6.646953231504538984, -7.453124999385467575 ) ) ;
#21502=EDGE_CURVE ( 'NONE', #33575, #34897, #10454, .T. ) ;
#21505=CARTESIAN_POINT ( 'NONE',  ( 30.57623723450533859, -6.928203230275506996, 159.4568924540549517 ) ) ;
#21509=CARTESIAN_POINT ( 'NONE',  ( 15.24356964374999990, 3.323476615752268604, -7.490624999385497418 ) ) ;
#21510=CYLINDRICAL_SURFACE ( 'NONE', #21642, 6.000000000000001776 ) ;
#21524=CARTESIAN_POINT ( 'NONE',  ( 25.36059234810526419, 3.464101615137711310, 168.6840780838932403 ) ) ;
#21535=CARTESIAN_POINT ( 'NONE',  ( 24.71676078210377625, 0.000000000000000000, 164.1196978580636028 ) ) ;
#21541=EDGE_LOOP ( 'NONE', ( #33365, #9000, #4018, #34568 ) ) ;
#21542=CARTESIAN_POINT ( 'NONE',  ( 15.24356964375000167, -3.323476615752272600, -1.453124999385472016 ) ) ;
#21544=CARTESIAN_POINT ( 'NONE',  ( 36.75931086529713099, 7.347880794884117764E-16, 161.2874679718108553 ) ) ;
#21545=CARTESIAN_POINT ( 'NONE',  ( 26.75643035624999655, -3.323476615752267715, -8.953124999385474680 ) ) ;
#21552=CARTESIAN_POINT ( 'NONE',  ( 34.19561101691670757, -5.196152422706629359, 166.4053843532510371 ) ) ;
#21558=CARTESIAN_POINT ( 'NONE',  ( 26.75643035624999655, 3.323476615752271268, -0.4406249993854897129 ) ) ;
#21564=LINE ( 'NONE', #33109, #34088 ) ;
#21566=CARTESIAN_POINT ( 'NONE',  ( 37.52080268400803931, -3.604726614523238837, 167.1967110400642866 ) ) ;
#21573=CARTESIAN_POINT ( 'NONE',  ( 33.71516498491316582, -5.196152422706635576, 160.9138610787959465 ) ) ;
#21579=CARTESIAN_POINT ( 'NONE',  ( 26.99999999999999645, 7.347880794884117764E-16, -6.018749998770944742 ) ) ;
#21581=CARTESIAN_POINT ( 'NONE',  ( 20.00041297495047843, 5.668978411116867733, -10.14010147226207614 ) ) ;
#21583=CARTESIAN_POINT ( 'NONE',  ( 24.59419801886489054, 0.000000000000000000, 162.7187990638720976 ) ) ;
#21584=CARTESIAN_POINT ( 'NONE',  ( 24.81804784950121601, -3.464101615137761048, 162.4827660882720295 ) ) ;
#21594=CARTESIAN_POINT ( 'NONE',  ( 15.24356964375000167, -3.323476615752272600, -6.965624999385507721 ) ) ;
#21598=CARTESIAN_POINT ( 'NONE',  ( 18.00000000000000355, -5.196152422706632912, -6.618749998770962151 ) ) ;
#21607=CARTESIAN_POINT ( 'NONE',  ( 24.83115269446006934, 3.604726614523236616, 165.4272033993090076 ) ) ;
#21609=CARTESIAN_POINT ( 'NONE',  ( 26.99999999999962341, -3.464101615137965773, -4.762500000000005507 ) ) ;
#21616=CARTESIAN_POINT ( 'NONE',  ( 30.96598682155142868, 7.209453229046475009, 163.9117506189718370 ) ) ;
#21617=CARTESIAN_POINT ( 'NONE',  ( 23.87821517812499650, 4.985214923628404904, -3.890624999385472460 ) ) ;
#21621=CARTESIAN_POINT ( 'NONE',  ( 28.35898146343970083, -5.196152422706638241, 168.5346827591855288 ) ) ;
#21631=CARTESIAN_POINT ( 'NONE',  ( 15.24356964375000167, -3.323476615752272600, -1.003124999385444527 ) ) ;
#21633=CARTESIAN_POINT ( 'NONE',  ( 26.99999999999999645, 7.347880794884117764E-16, -8.718749998770952914 ) ) ;
#21639=CARTESIAN_POINT ( 'NONE',  ( 24.66936984698473623, 3.604726614523240613, 163.5780169909762094 ) ) ;
#21642=AXIS2_PLACEMENT_3D ( 'NONE', #33054, #30212, #4237 ) ;
#21645=CARTESIAN_POINT ( 'NONE',  ( 36.63184559142159458, 7.347880794884125653E-16, 159.8305332246273167 ) ) ;
#21646=CARTESIAN_POINT ( 'NONE',  ( 25.03052145599531997, 0.000000000000000000, 167.7059987711938902 ) ) ;
#21656=ORIENTED_EDGE ( 'NONE', *, *, #5536, .F. ) ;
#21659=DIRECTION ( 'NONE',  ( 0.08715574274765150453, 0.000000000000000000, 0.9961946980917461003 ) ) ;
#21667=VERTEX_POINT ( 'NONE', #33397 ) ;
#21672=CARTESIAN_POINT ( 'NONE',  ( 26.75643035624999655, 7.049594010296217766E-16, -5.428124999385497418 ) ) ;
#21676=CARTESIAN_POINT ( 'NONE',  ( 26.75643035624999655, 7.049594010296217766E-16, -7.115624999385477878 ) ) ;
#21684=CARTESIAN_POINT ( 'NONE',  ( 27.68897169117423829, 5.196152422706630247, 160.8764360188296223 ) ) ;
#21689=CARTESIAN_POINT ( 'NONE',  ( 27.00000000000047251, 3.464101615137479495, -6.937499999999990230 ) ) ;
#21697=( BOUNDED_CURVE ( )  B_SPLINE_CURVE ( 2, ( #6715, #20753, #27363, #21135, #18287, #32299, #1015 ),
 .UNSPECIFIED., .F., .F. ) 
 B_SPLINE_CURVE_WITH_KNOTS ( ( 3, 2, 2, 3 ),
 ( 0.2173913043478263030, 0.2246376811594205936, 0.2318840579710149119, 0.2391304347826092025 ),
 .UNSPECIFIED. ) 
 CURVE ( )  GEOMETRIC_REPRESENTATION_ITEM ( )  RATIONAL_B_SPLINE_CURVE ( ( 0.9999999999999958922, 0.8660254037844428154, 1.000000000000000000, 0.8660254037844387076, 1.000000000000000000, 0.8660254037844294928, 1.000000000000009326 ) ) 
 REPRESENTATION_ITEM ( '' )  );
#21698=CYLINDRICAL_SURFACE ( 'NONE', #25246, 6.000000000000001776 ) ;
#21704=CARTESIAN_POINT ( 'NONE',  ( 28.12366095802104127, -5.196152422706638241, 165.8449570743377990 ) ) ;
#21713=CARTESIAN_POINT ( 'NONE',  ( 34.12043918868973691, 5.196152422706637353, 165.5461664249225748 ) ) ;
#21716=CARTESIAN_POINT ( 'NONE',  ( 24.72002912245681117, -3.604726614523240613, 164.1570551592420486 ) ) ;
#21723=VERTEX_POINT ( 'NONE', #2480 ) ;
#21725=CARTESIAN_POINT ( 'NONE',  ( 26.75643035624999655, 3.323476615752271268, -0.7781249993854945091 ) ) ;
#21727=CARTESIAN_POINT ( 'NONE',  ( 36.76257920564959392, 3.464101615138092782, 161.3248252729893579 ) ) ;
#21728=CARTESIAN_POINT ( 'NONE',  ( 18.12178482187500350, -4.985214923628407568, -7.715624999385467753 ) ) ;
#21731=CARTESIAN_POINT ( 'NONE',  ( 36.75604252494468227, -3.464101615137414214, 161.2501106706323242 ) ) ;
#21735=CARTESIAN_POINT ( 'NONE',  ( 34.15639093268026016, -5.196152422706629359, 165.9570967391097440 ) ) ;
#21741=CARTESIAN_POINT ( 'NONE',  ( 26.75643035624999655, 7.049594010296217766E-16, -1.378124999385471616 ) ) ;
#21747=DIRECTION ( 'NONE',  ( 0.08715574274765150453, 0.000000000000000000, 0.9961946980917461003 ) ) ;
#21749=CARTESIAN_POINT ( 'NONE',  ( 31.11796464796764994, 7.209453229046482114, 165.6488651237693261 ) ) ;
#21757=ADVANCED_FACE ( 'NONE', ( #191 ), #29182, .T. ) ;
#21760=CARTESIAN_POINT ( 'NONE',  ( 16.83757916490470663, -4.525028440652736350, -7.983280259209641905 ) ) ;
#21766=CARTESIAN_POINT ( 'NONE',  ( 21.00000000000000000, 6.928203230275506996, -2.812499999999997335 ) ) ;
#21767=CARTESIAN_POINT ( 'NONE',  ( 37.01420992928731835, 7.646167579472024665E-16, 161.4063293574060083 ) ) ;
#21768=CARTESIAN_POINT ( 'NONE',  ( 27.77068019989305370, -5.196152422706638241, 161.8103685470662469 ) ) ;
#21771=EDGE_CURVE ( 'NONE', #1229, #13971, #29486, .T. ) ;
#21777=CARTESIAN_POINT ( 'NONE',  ( 26.99999999999940314, 3.464101615138096335, -1.087499999999968825 ) ) ;
#21779=CARTESIAN_POINT ( 'NONE',  ( 21.00000000000000000, -6.646953231504538984, -7.340624999385477523 ) ) ;
#21788=EDGE_CURVE ( 'NONE', #13971, #21667, #20239, .T. ) ;
#21792=CARTESIAN_POINT ( 'NONE',  ( 30.84832656884210067, 7.209453229046475009, 162.5668877765479863 ) ) ;
#21795=CARTESIAN_POINT ( 'NONE',  ( 20.99999999999999645, -6.928203230275506996, -3.881249998770961440 ) ) ;
#21798=DIRECTION ( 'NONE',  ( 0.08715574274765150453, 0.000000000000000000, 0.9961946980917461003 ) ) ;
#21804=CARTESIAN_POINT ( 'NONE',  ( 37.13677269252619340, 7.646167579472015790E-16, 162.8072281515975135 ) ) ;
#21805=CARTESIAN_POINT ( 'NONE',  ( 15.24356964375000167, -3.323476615752272600, -5.053124999385469884 ) ) ;
#21807=CARTESIAN_POINT ( 'NONE',  ( 25.36386068845838082, 0.000000000000000000, 168.7214353850716293 ) ) ;
#21808=CARTESIAN_POINT ( 'NONE',  ( 36.66779733530574958, -3.464101615137326728, 160.2414635375900787 ) ) ;
#21812=VECTOR ( 'NONE', #977, 1000.000000000000000 ) ;
#21817=CARTESIAN_POINT ( 'NONE',  ( 21.00000000000000000, -6.646953231504538984, -4.078124999385484450 ) ) ;
#21820=CARTESIAN_POINT ( 'NONE',  ( 23.99999999999999645, 5.196152422706631135, -8.643749998770960730 ) ) ;
#21827=CARTESIAN_POINT ( 'NONE',  ( 24.51902619074504130, -3.604726614523244610, 161.8595811367679573 ) ) ;
#21834=EDGE_LOOP ( 'NONE', ( #14859, #17137, #6859, #18223 ) ) ;
#21844=DIRECTION ( 'NONE',  ( 0.000000000000000000, 0.000000000000000000, 1.000000000000000000 ) ) ;
#21849=CYLINDRICAL_SURFACE ( 'NONE', #25624, 5.999999999999994671 ) ;
#21858=CARTESIAN_POINT ( 'NONE',  ( 25.44230085693126497, 0.000000000000000000, 169.6180106133541869 ) ) ;
#21859=CARTESIAN_POINT ( 'NONE',  ( 26.75643035624999655, 7.049594010296217766E-16, -8.128124999385477167 ) ) ;
#21861=VERTEX_POINT ( 'NONE', #32745 ) ;
#21862=CARTESIAN_POINT ( 'NONE',  ( 26.75643035624999655, 7.049594010296217766E-16, -6.665624999385472371 ) ) ;
#21867=CARTESIAN_POINT ( 'NONE',  ( 27.57131143846490673, 5.196152422706630247, 159.5315731764057716 ) ) ;
#21875=DIRECTION ( 'NONE',  ( 0.08715574274765150453, 0.000000000000000000, 0.9961946980917461003 ) ) ;
#21886=CARTESIAN_POINT ( 'NONE',  ( 24.85726793373807908, -3.464101615138005741, 162.9310537024133225 ) ) ;
#21888=CARTESIAN_POINT ( 'NONE',  ( 26.99999999999999645, 7.347880794884117764E-16, -7.818749998770941012 ) ) ;
#21895=LINE ( 'NONE', #5002, #11145 ) ;
#21896=LINE ( 'NONE', #33444, #36209 ) ;
#21899=CARTESIAN_POINT ( 'NONE',  ( 34.17721086063072988, -5.407089921784855591, 164.7977454806546120 ) ) ;
#21900=( BOUNDED_CURVE ( )  B_SPLINE_CURVE ( 2, ( #15089, #23434, #6370, #2776, #37450, #31589, #17941 ),
 .UNSPECIFIED., .F., .F. ) 
 B_SPLINE_CURVE_WITH_KNOTS ( ( 3, 2, 2, 3 ),
 ( 0.5434782608695640782, 0.5507246376811584243, 0.5579710144927527704, 0.5652173913043470055 ),
 .UNSPECIFIED. ) 
 CURVE ( )  GEOMETRIC_REPRESENTATION_ITEM ( )  RATIONAL_B_SPLINE_CURVE ( ( 1.000000000000020428, 0.8660254037844181685, 1.000000000000000000, 0.8660254037844387076, 1.000000000000000000, 0.8660254037844530295, 0.9999999999999856781 ) ) 
 REPRESENTATION_ITEM ( '' )  );
#21901=CARTESIAN_POINT ( 'NONE',  ( 15.00000000000000000, 0.000000000000000000, -5.399999999999987921 ) ) ;
#21903=ORIENTED_EDGE ( 'NONE', *, *, #26608, .F. ) ;
#21907=CARTESIAN_POINT ( 'NONE',  ( 15.00000000000000178, -3.464101615137757051, -4.856249998770946874 ) ) ;
#21910=CARTESIAN_POINT ( 'NONE',  ( 21.00000000000000000, -6.646953231504538984, -9.028124999385470417 ) ) ;
#21918=CARTESIAN_POINT ( 'NONE',  ( 37.19073179189800271, 7.347880794884117764E-16, 166.2186317273649934 ) ) ;
#21925=CARTESIAN_POINT ( 'NONE',  ( 15.24356964374999990, 0.000000000000000000, -1.603124999385474592 ) ) ;
#21930=ORIENTED_EDGE ( 'NONE', *, *, #15239, .T. ) ;
#21931=CARTESIAN_POINT ( 'NONE',  ( 25.40308077269482112, 0.000000000000000000, 169.1697229992128939 ) ) ;
#21935=CARTESIAN_POINT ( 'NONE',  ( 30.98069435314010178, -7.209453229046482114, 164.0798584742748574 ) ) ;
#21946=CARTESIAN_POINT ( 'NONE',  ( 21.00000000000000355, 0.000000000000000000, 50.00000000000001421 ) ) ;
#21952=CARTESIAN_POINT ( 'NONE',  ( 24.00000000000000000, -5.196152422706629359, -1.200000000000006617 ) ) ;
#21953=CARTESIAN_POINT ( 'NONE',  ( 37.09265009776020605, 7.646167579472024665E-16, 162.3029045856885659 ) ) ;
#21954=CARTESIAN_POINT ( 'NONE',  ( 24.70038759679188800, -3.464101615137761048, 161.1379032458482072 ) ) ;
#21957=EDGE_CURVE ( 'NONE', #15760, #16220, #19031, .T. ) ;
#21963=DIRECTION ( 'NONE',  ( 0.000000000000000000, 0.000000000000000000, 1.000000000000000000 ) ) ;
#21965=CARTESIAN_POINT ( 'NONE',  ( 26.75643035624999655, 7.049594010296217766E-16, -5.878124999385475391 ) ) ;
#21980=CARTESIAN_POINT ( 'NONE',  ( 27.62402916835064559, 5.407089921784856479, 161.5314637101514279 ) ) ;
#21981=FACE_OUTER_BOUND ( 'NONE', #30461, .T. ) ;
#21992=CARTESIAN_POINT ( 'NONE',  ( 27.87242303518145548, -5.407089921784859143, 164.3706185997128841 ) ) ;
#21993=CARTESIAN_POINT ( 'NONE',  ( 21.00000000000000000, 6.646953231504538984, -5.653124999385485516 ) ) ;
#21995=CARTESIAN_POINT ( 'NONE',  ( 37.29858702344112231, 7.347880794884125653E-16, 167.4514226650291562 ) ) ;
#21996=CARTESIAN_POINT ( 'NONE',  ( 36.67106567565804198, 7.347880794884125653E-16, 160.2788208387686097 ) ) ;
#22004=CARTESIAN_POINT ( 'NONE',  ( 26.75643035624999655, 7.049594010296217766E-16, -4.865624999385476102 ) ) ;
#22007=CARTESIAN_POINT ( 'NONE',  ( 26.99999999999999645, 7.347880794884117764E-16, -9.618749998770963927 ) ) ;
#22013=CARTESIAN_POINT ( 'NONE',  ( 33.78010750773675852, -5.407089921784861808, 160.2588333874741124 ) ) ;
#22023=DIRECTION ( 'NONE',  ( 0.000000000000000000, 0.000000000000000000, 1.000000000000000000 ) ) ;
#22024=DIRECTION ( 'NONE',  ( 0.9961946980917461003, 0.000000000000000000, -0.08715574274765142126 ) ) ;
#22029=EDGE_LOOP ( 'NONE', ( #34517, #17885, #5942, #9864 ) ) ;
#22036=CARTESIAN_POINT ( 'NONE',  ( 20.99999999999999645, 0.000000000000000000, -8.000000000000000000 ) ) ;
#22038=CARTESIAN_POINT ( 'NONE',  ( 25.01414827068380475, -3.464101615137975543, 164.7242041589784947 ) ) ;
#22039=VECTOR ( 'NONE', #36882, 1000.000000000000000 ) ;
#22042=CARTESIAN_POINT ( 'NONE',  ( 37.14170668649535401, 7.347880794884125653E-16, 165.6582722084640125 ) ) ;
#22048=CARTESIAN_POINT ( 'NONE',  ( 18.12178482187499640, 4.985214923628404904, -6.628124999385476279 ) ) ;
#22050=ORIENTED_EDGE ( 'NONE', *, *, #18769, .T. ) ;
#22052=CARTESIAN_POINT ( 'NONE',  ( 37.60251119283397259, 7.646167579472024665E-16, 168.1306435695252901 ) ) ;
#22061=ADVANCED_FACE ( 'NONE', ( #30283 ), #4499, .T. ) ;
#22089=CARTESIAN_POINT ( 'NONE',  ( 37.29692136982500728, 3.604726614523238837, 164.6377359093410746 ) ) ;
#22092=EDGE_LOOP ( 'NONE', ( #8112, #18242, #25000, #18421 ) ) ;
#22094=EDGE_LOOP ( 'NONE', ( #24967, #13137, #377, #10008 ) ) ;
#22096=CARTESIAN_POINT ( 'NONE',  ( 18.00000000000000000, 5.196152422706630247, -4.968749998770949361 ) ) ;
#22097=CARTESIAN_POINT ( 'NONE',  ( 15.24356964375000167, -3.323476615752272600, -0.5531249993854806535 ) ) ;
#22098=CARTESIAN_POINT ( 'NONE',  ( 15.00000000000000000, 0.000000000000000000, -1.349999999999990097 ) ) ;
#22107=CARTESIAN_POINT ( 'NONE',  ( 37.03058311459920304, -3.464101615137751278, 164.3881239696214038 ) ) ;
#22112=CARTESIAN_POINT ( 'NONE',  ( 23.87821517812500005, -4.985214923628404016, -2.353124999385475036 ) ) ;
#22121=CARTESIAN_POINT ( 'NONE',  ( 17.00000000000002132, 2.343145750507694913, 50.17464377163449285 ) ) ;
#22122=CARTESIAN_POINT ( 'NONE',  ( 28.01132750018552287, 5.407089921784862696, 165.9583038997966185 ) ) ;
#22126=( BOUNDED_CURVE ( )  B_SPLINE_CURVE ( 2, ( #300, #29485, #29295, #34987, #3333 ),
 .UNSPECIFIED., .F., .F. ) 
 B_SPLINE_CURVE_WITH_KNOTS ( ( 3, 2, 3 ),
 ( 0.9565217391304334793, 0.9637681159420286026, 0.9662082966761268432 ),
 .UNSPECIFIED. ) 
 CURVE ( )  GEOMETRIC_REPRESENTATION_ITEM ( )  RATIONAL_B_SPLINE_CURVE ( ( 1.000000000000024647, 0.8660254037844140607, 1.000000000000000000, 0.9548847324609615050, 0.9401541411607547971 ) ) 
 REPRESENTATION_ITEM ( '' )  );
#22130=EDGE_CURVE ( 'NONE', #30675, #28137, #15699, .T. ) ;
#22139=CARTESIAN_POINT ( 'NONE',  ( 26.99999999999999645, 3.464101615137755275, -2.437499999999996003 ) ) ;
#22140=CARTESIAN_POINT ( 'NONE',  ( 24.74781001545762393, 3.604726614523240613, 164.4745922192587670 ) ) ;
#22141=CARTESIAN_POINT ( 'NONE',  ( 30.66448242393021673, 6.928203230275514990, 160.4655395846485249 ) ) ;
#22152=CARTESIAN_POINT ( 'NONE',  ( 15.24356964375000167, -3.323476615752272600, -9.665624999385482141 ) ) ;
#22167=CARTESIAN_POINT ( 'NONE',  ( 24.52066036092156054, 0.000000000000000000, 161.8782597873571660 ) ) ;
#22171=CARTESIAN_POINT ( 'NONE',  ( 37.29858702344112231, 7.347880794884125653E-16, 167.4514226650291562 ) ) ;
#22177=EDGE_LOOP ( 'NONE', ( #19948, #17103, #29439, #22281 ) ) ;
#22178=CARTESIAN_POINT ( 'NONE',  ( 31.08364707426076023, 7.209453229046475009, 165.2566134613956876 ) ) ;
#22179=CARTESIAN_POINT ( 'NONE',  ( 23.87821517812499650, 4.985214923628404904, -6.140624999385474680 ) ) ;
#22182=CARTESIAN_POINT ( 'NONE',  ( 28.31976137920325698, -5.196152422706638241, 168.0863951450442642 ) ) ;
#22185=CARTESIAN_POINT ( 'NONE',  ( 29.49159713443669162, 6.148716367659647020, 159.4989838507731008 ) ) ;
#22194=CARTESIAN_POINT ( 'NONE',  ( 15.24356964375000167, -3.323476615752272600, -5.053124999385469884 ) ) ;
#22197=CARTESIAN_POINT ( 'NONE',  ( 21.00000000000000000, -6.928203230275506996, -10.18124999877096570 ) ) ;
#22222=CARTESIAN_POINT ( 'NONE',  ( 24.61867908796596183, 0.000000000000000000, 160.2039707163872038 ) ) ;
#22226=CARTESIAN_POINT ( 'NONE',  ( 27.66282496834995186, -5.196152422706632912, 160.5775776094020557 ) ) ;
#22228=CARTESIAN_POINT ( 'NONE',  ( 15.00000000000000000, 0.000000000000000000, -8.550000000000002487 ) ) ;
#22235=CARTESIAN_POINT ( 'NONE',  ( 26.75643035624999655, 7.049594010296217766E-16, -7.678124999385471661 ) ) ;
#22237=EDGE_CURVE ( 'NONE', #33229, #17991, #35293, .T. ) ;
#22238=ORIENTED_EDGE ( 'NONE', *, *, #32869, .T. ) ;
#22243=CARTESIAN_POINT ( 'NONE',  ( 31.37289519550453321, -7.209453229046482114, 168.5627346156876740 ) ) ;
#22250=CARTESIAN_POINT ( 'NONE',  ( 24.82458453031440726, 0.000000000000000000, 162.5574806918533000 ) ) ;
#22269=VERTEX_POINT ( 'NONE', #611 ) ;
#22275=CARTESIAN_POINT ( 'NONE',  ( 27.63710252976279591, -5.407089921784859143, 161.6808929148651828 ) ) ;
#22276=CARTESIAN_POINT ( 'NONE',  ( 15.24356964375000167, -3.323476615752272600, -0.6656249993855035685 ) ) ;
#22281=ORIENTED_EDGE ( 'NONE', *, *, #10401, .T. ) ;
#22282=CARTESIAN_POINT ( 'NONE',  ( 26.99999999999999645, 7.347880794884117764E-16, -3.768749998770942966 ) ) ;
#22283=CARTESIAN_POINT ( 'NONE',  ( 23.87821517812500005, -4.985214923628404016, -3.590624999385477523 ) ) ;
#22291=CARTESIAN_POINT ( 'NONE',  ( 36.95541128647934670, 7.347880794884117764E-16, 163.5289060425172636 ) ) ;
#22295=CARTESIAN_POINT ( 'NONE',  ( 18.12178482187499640, 4.985214923628404904, -2.128124999385472282 ) ) ;
#22301=CARTESIAN_POINT ( 'NONE',  ( 36.83121435295620927, 3.464101615138126977, 162.1093285965122277 ) ) ;
#22304=DIRECTION ( 'NONE',  ( 0.08715574274765150453, 0.000000000000000000, 0.9961946980917461003 ) ) ;
#22305=CARTESIAN_POINT ( 'NONE',  ( 34.21152843433763024, -5.407089921784861808, 165.1899971430282505 ) ) ;
#22320=CARTESIAN_POINT ( 'NONE',  ( 15.00000000000000000, 0.000000000000000000, -2.700000000000008171 ) ) ;
#22321=CARTESIAN_POINT ( 'NONE',  ( 26.78253581145591511, -0.6185957445801392174, -8.000000000000005329 ) ) ;
#22322=CARTESIAN_POINT ( 'NONE',  ( 27.57990657358465114, 5.407089921784862696, 161.0271401442424803 ) ) ;
#22324=CARTESIAN_POINT ( 'NONE',  ( 24.66116751255544060, -3.464101615137761048, 160.6896156317069426 ) ) ;
#22329=VERTEX_POINT ( 'NONE', #804 ) ;
#22330=ORIENTED_EDGE ( 'NONE', *, *, #28590, .F. ) ;
#22332=CARTESIAN_POINT ( 'NONE',  ( 15.00000000000054712, 3.464101615138070134, -0.9375000000000270894 ) ) ;
#22334=CARTESIAN_POINT ( 'NONE',  ( 23.87821517812500005, -4.985214923628404016, -9.103124999385482141 ) ) ;
#22340=EDGE_CURVE ( 'NONE', #15182, #1464, #29618, .T. ) ;
#22348=CARTESIAN_POINT ( 'NONE',  ( 25.08605175844997248, 3.464101615137603396, 165.5460647849041607 ) ) ;
#22349=CARTESIAN_POINT ( 'NONE',  ( 36.90472052746056875, 3.604726614523238837, 160.1548597679282295 ) ) ;
#22350=CARTESIAN_POINT ( 'NONE',  ( 37.15478004801428824, 3.464101615137938683, 165.8077014144021177 ) ) ;
#22353=CARTESIAN_POINT ( 'NONE',  ( 36.68413903717654279, 3.464101615138184265, 160.4282500447067434 ) ) ;
#22361=CARTESIAN_POINT ( 'NONE',  ( 34.21643094486717729, -5.407089921784855591, 165.2460330947959051 ) ) ;
#22362=CARTESIAN_POINT ( 'NONE',  ( 23.87821517812499650, 4.985214923628404904, -4.340624999385478411 ) ) ;
#22365=CARTESIAN_POINT ( 'NONE',  ( 15.15508984909395451, -1.204559016176377728, -8.000000000000001776 ) ) ;
#22366=CARTESIAN_POINT ( 'NONE',  ( 25.36059234810534235, 3.464101615137757051, 168.6840780838931835 ) ) ;
#22370=( BOUNDED_CURVE ( )  B_SPLINE_CURVE ( 3, ( #10159, #4468, #22425, #33285 ),
 .UNSPECIFIED., .F., .T. ) 
 B_SPLINE_CURVE_WITH_KNOTS ( ( 4, 4 ),
 ( 0.000000000000000000, 3.141592653589793116 ),
 .UNSPECIFIED. ) 
 CURVE ( )  GEOMETRIC_REPRESENTATION_ITEM ( )  RATIONAL_B_SPLINE_CURVE ( ( 1.000000000000000000, 0.3333333333333333703, 0.3333333333333333703, 1.000000000000000000 ) ) 
 REPRESENTATION_ITEM ( '' )  );
#22377=CARTESIAN_POINT ( 'NONE',  ( 15.24356964374999990, 0.000000000000000000, -5.090624999385479299 ) ) ;
#22380=CARTESIAN_POINT ( 'NONE',  ( 21.00000000000000000, -6.646953231504538984, -2.390624999385460470 ) ) ;
#22394=CYLINDRICAL_SURFACE ( 'NONE', #5260, 6.000000000000001776 ) ;
#22396=EDGE_CURVE ( 'NONE', #4196, #30479, #18076, .T. ) ;
#22401=VERTEX_POINT ( 'NONE', #9536 ) ;
#22410=DIRECTION ( 'NONE',  ( 0.9961946980917462113, 0.000000000000000000, -0.08715574274765118534 ) ) ;
#22412=CARTESIAN_POINT ( 'NONE',  ( 15.00000000000000000, 0.000000000000000000, -9.899999999999991473 ) ) ;
#22418=CARTESIAN_POINT ( 'NONE',  ( 15.24356964375000167, -3.323476615752272600, -6.065624999385484273 ) ) ;
#22425=CARTESIAN_POINT ( 'NONE',  ( 27.00000000000001776, -11.99999999999999822, 49.73803434254939759 ) ) ;
#22427=CARTESIAN_POINT ( 'NONE',  ( 24.00000000000000000, -5.196152422706629359, -7.500000000000007105 ) ) ;
#22429=EDGE_CURVE ( 'NONE', #37490, #26027, #29407, .T. ) ;
#22441=CARTESIAN_POINT ( 'NONE',  ( 20.99999999999999645, 0.000000000000000000, -8.000000000000000000 ) ) ;
#22459=CARTESIAN_POINT ( 'NONE',  ( 24.63505227327785363, 3.604726614523236616, 163.1857653286025709 ) ) ;
#22460=CARTESIAN_POINT ( 'NONE',  ( 26.75643035624999655, 7.049594010296217766E-16, -0.9281249993854934210 ) ) ;
#22464=ORIENTED_EDGE ( 'NONE', *, *, #28651, .T. ) ;
#22465=CARTESIAN_POINT ( 'NONE',  ( 18.00000000000000355, -5.196152422706632912, -5.718749998770950249 ) ) ;
#22466=CARTESIAN_POINT ( 'NONE',  ( 20.99999999999999645, 6.646953231504538984, -1.603124999385460159 ) ) ;
#22478=CARTESIAN_POINT ( 'NONE',  ( 34.07795076420737246, -5.196152422706629359, 165.0605215108271864 ) ) ;
#22485=CARTESIAN_POINT ( 'NONE',  ( 20.99999999999999645, -6.646953231504538984, -1.490624999385500749 ) ) ;
#22493=CARTESIAN_POINT ( 'NONE',  ( 24.55824627498148160, -3.604726614523244610, 162.3078687509092788 ) ) ;
#22498=CARTESIAN_POINT ( 'NONE',  ( 33.68574992184294103, -5.196152422706629359, 160.5776453694143129 ) ) ;
#22508=CARTESIAN_POINT ( 'NONE',  ( 18.00000000000000355, -5.196152422706632912, -1.274999999999998357 ) ) ;
#22509=CARTESIAN_POINT ( 'NONE',  ( 26.71249821599011653, 0.8257047527043690494, -7.999999999999998224 ) ) ;
#22510=CARTESIAN_POINT ( 'NONE',  ( 33.79318086914889818, 5.407089921784862696, 160.4082625921878673 ) ) ;
#22512=CARTESIAN_POINT ( 'NONE',  ( 28.26462387754589045, -5.407089921784859143, 168.8534947411257576 ) ) ;
#22516=ORIENTED_EDGE ( 'NONE', *, *, #17525, .T. ) ;
#22518=VECTOR ( 'NONE', #15691, 1000.000000000000000 ) ;
#22520=CARTESIAN_POINT ( 'NONE',  ( 37.22014685496823461, 7.347880794884125653E-16, 166.5548474367465985 ) ) ;
#22522=CARTESIAN_POINT ( 'NONE',  ( 15.24356964374999990, 3.323476615752268604, -9.290624999385480365 ) ) ;
#22525=CARTESIAN_POINT ( 'NONE',  ( 15.02283181144952628, 7.347880794884122694E-16, 50.52293445648592751 ) ) ;
#22535=CARTESIAN_POINT ( 'NONE',  ( 36.94067227134398479, 7.646167579472015790E-16, 160.5657900808910767 ) ) ;
#22543=CARTESIAN_POINT ( 'NONE',  ( 15.00000000000000000, 0.000000000000000000, -0.8437499987709595750 ) ) ;
#22544=ORIENTED_EDGE ( 'NONE', *, *, #17498, .F. ) ;
#22545=CARTESIAN_POINT ( 'NONE',  ( 37.09755260828975310, 7.646167579472015790E-16, 162.3589405374562205 ) ) ;
#22546=CARTESIAN_POINT ( 'NONE',  ( 26.75643035624999655, -3.323476615752267715, -4.903124999385481964 ) ) ;
#22548=CARTESIAN_POINT ( 'NONE',  ( 34.45992230116843302, 5.407089921784862696, 168.0291520325897636 ) ) ;
#22549=CARTESIAN_POINT ( 'NONE',  ( 31.17434351900397971, 6.928203230275514990, 166.2932785684852490 ) ) ;
#22553=EDGE_CURVE ( 'NONE', #32257, #15602, #24111, .T. ) ;
#22556=ORIENTED_EDGE ( 'NONE', *, *, #29268, .F. ) ;
#22560=CARTESIAN_POINT ( 'NONE',  ( 23.87821517812500005, -4.985214923628404016, -4.490624999385461891 ) ) ;
#22563=CARTESIAN_POINT ( 'NONE',  ( 26.75643035624999655, 7.049594010296217766E-16, -2.278124999385483740 ) ) ;
#22569=( BOUNDED_CURVE ( )  B_SPLINE_CURVE ( 2, ( #17691, #35106, #29230, #37380, #34921, #11803, #46 ),
 .UNSPECIFIED., .F., .F. ) 
 B_SPLINE_CURVE_WITH_KNOTS ( ( 3, 2, 2, 3 ),
 ( 0.2173913043478257756, 0.2246376811594198997, 0.2318840579710139960, 0.2391304347826081200 ),
 .UNSPECIFIED. ) 
 CURVE ( )  GEOMETRIC_REPRESENTATION_ITEM ( )  RATIONAL_B_SPLINE_CURVE ( ( 1.000000000000005773, 0.8660254037844331565, 1.000000000000000000, 0.8660254037844387076, 1.000000000000000000, 0.8660254037844494768, 0.9999999999999892308 ) ) 
 REPRESENTATION_ITEM ( '' )  );
#22570=EDGE_CURVE ( 'NONE', #20178, #32003, #30712, .T. ) ;
#22577=EDGE_CURVE ( 'NONE', #18882, #21667, #30447, .T. ) ;
#22579=CARTESIAN_POINT ( 'NONE',  ( 21.00000000000000355, 0.000000000000000000, 50.00000000000001421 ) ) ;
#22587=( BOUNDED_CURVE ( )  B_SPLINE_CURVE ( 2, ( #14051, #25601, #34319, #188, #14416, #3032, #11754 ),
 .UNSPECIFIED., .F., .F. ) 
 B_SPLINE_CURVE_WITH_KNOTS ( ( 3, 2, 2, 3 ),
 ( 0.6086956521739120829, 0.6159420289855060959, 0.6231884057971003310, 0.6304347826086944551 ),
 .UNSPECIFIED. ) 
 CURVE ( )  GEOMETRIC_REPRESENTATION_ITEM ( )  RATIONAL_B_SPLINE_CURVE ( ( 1.000000000000018430, 0.8660254037844202779, 1.000000000000000000, 0.8660254037844387076, 1.000000000000000000, 0.8660254037844612451, 0.9999999999999774625 ) ) 
 REPRESENTATION_ITEM ( '' )  );
#22599=CARTESIAN_POINT ( 'NONE',  ( 15.00000000000000000, 3.464101615137752166, -9.937500000000000000 ) ) ;
#22600=ORIENTED_EDGE ( 'NONE', *, *, #28607, .T. ) ;
#22605=CARTESIAN_POINT ( 'NONE',  ( 21.00000000000000000, 6.646953231504538984, -6.215624999385504168 ) ) ;
#22613=CARTESIAN_POINT ( 'NONE',  ( 25.41288579386105440, 0.000000000000000000, 169.2817949039725818 ) ) ;
#22619=VERTEX_POINT ( 'NONE', #33917 ) ;
#22641=EDGE_LOOP ( 'NONE', ( #24968, #951, #36925, #32638 ) ) ;
#22648=CARTESIAN_POINT ( 'NONE',  ( 30.78949644248743311, -7.209453229046475009, 161.8944563553360467 ) ) ;
#22654=CARTESIAN_POINT ( 'NONE',  ( 26.99999999999999645, 3.464101615137755275, -4.631249998770964993 ) ) ;
#22655=CARTESIAN_POINT ( 'NONE',  ( 26.75643035624999655, 3.323476615752271268, -2.578124999385477345 ) ) ;
#22657=CARTESIAN_POINT ( 'NONE',  ( 20.99999999999999645, 6.928203230275506996, -6.412499999999995204 ) ) ;
#22659=CARTESIAN_POINT ( 'NONE',  ( 37.25609859885201303, -3.464101615137556767, 166.9657777497094173 ) ) ;
#22663=VECTOR ( 'NONE', #5205, 1000.000000000000000 ) ;
#22667=CARTESIAN_POINT ( 'NONE',  ( 36.91945954259593776, 3.464101615137755275, 163.1179757295544164 ) ) ;
#22671=CARTESIAN_POINT ( 'NONE',  ( 23.87821517812500005, -4.985214923628404016, -5.503124999385489602 ) ) ;
#22676=( BOUNDED_CURVE ( )  B_SPLINE_CURVE ( 2, ( #6777, #12466, #9436, #2994, #8872, #17787, #6020 ),
 .UNSPECIFIED., .F., .F. ) 
 B_SPLINE_CURVE_WITH_KNOTS ( ( 3, 2, 2, 3 ),
 ( 0.8695652173913032135, 0.8768115942028972265, 0.8840579710144913506, 0.8913043478260852526 ),
 .UNSPECIFIED. ) 
 CURVE ( )  GEOMETRIC_REPRESENTATION_ITEM ( )  RATIONAL_B_SPLINE_CURVE ( ( 1.000000000000020428, 0.8660254037844181685, 1.000000000000000000, 0.8660254037844387076, 1.000000000000000000, 0.8660254037844694608, 0.9999999999999692468 ) ) 
 REPRESENTATION_ITEM ( '' )  );
#22681=CARTESIAN_POINT ( 'NONE',  ( 27.77600699476686330, 5.407089921784862696, 163.2685782149489171 ) ) ;
#22684=EDGE_CURVE ( 'NONE', #21723, #23273, #28043, .T. ) ;
#22697=CARTESIAN_POINT ( 'NONE',  ( 26.99999999999999645, 7.347880794884117764E-16, -5.175000000000013145 ) ) ;
#22700=CARTESIAN_POINT ( 'NONE',  ( 33.83240095338533848, 5.407089921784862696, 160.8565502063291603 ) ) ;
#22702=CARTESIAN_POINT ( 'NONE',  ( 34.46482481169798717, 5.407089921784857367, 168.0851879843573897 ) ) ;
#22708=VERTEX_POINT ( 'NONE', #33320 ) ;
#22711=CARTESIAN_POINT ( 'NONE',  ( 36.72009078106068358, 7.347880794884117764E-16, 160.8391803576695622 ) ) ;
#22713=CARTESIAN_POINT ( 'NONE',  ( 21.00000000000000000, -6.646953231504538984, -8.690624999385464733 ) ) ;
#22716=CARTESIAN_POINT ( 'NONE',  ( 20.99999999999999645, 6.928203230275506996, -7.312499999999986677 ) ) ;
#22717=CARTESIAN_POINT ( 'NONE',  ( 30.74537384772143866, -7.209453229046482114, 161.3901327894271276 ) ) ;
#22725=CARTESIAN_POINT ( 'NONE',  ( 24.36378002397578868, 0.000000000000000000, 160.0851093307920223 ) ) ;
#22726=CARTESIAN_POINT ( 'NONE',  ( 23.99999999999999645, 5.196152422706631135, -0.5437499987709648597 ) ) ;
#22735=CARTESIAN_POINT ( 'NONE',  ( 30.80910648460564971, 7.209453229046475009, 162.1186001624066932 ) ) ;
#22736=CARTESIAN_POINT ( 'NONE',  ( 15.24356964374999990, 3.323476615752268604, -6.928124999385478766 ) ) ;
#22738=CARTESIAN_POINT ( 'NONE',  ( 37.44236251553516581, -3.604726614523238837, 166.3001358117817006 ) ) ;
#22739=CARTESIAN_POINT ( 'NONE',  ( 28.28054129496681313, -5.196152422706638241, 167.6381075309029711 ) ) ;
#22746=VERTEX_POINT ( 'NONE', #15895 ) ;
#22747=ORIENTED_EDGE ( 'NONE', *, *, #35157, .F. ) ;
#22752=CARTESIAN_POINT ( 'NONE',  ( 26.75643035624999655, 3.323476615752271712, -2.240624999385472549 ) ) ;
#22765=CARTESIAN_POINT ( 'NONE',  ( 25.45210587809749825, 0.000000000000000000, 169.7300825181138748 ) ) ;
#22775=CARTESIAN_POINT ( 'NONE',  ( 18.12178482187499640, 4.985214923628404904, -0.2156249993854608693 ) ) ;
#22782=CARTESIAN_POINT ( 'NONE',  ( 21.00000000000000000, 6.928203230275506996, -8.662499999999972999 ) ) ;
#22787=CARTESIAN_POINT ( 'NONE',  ( 18.12178482187500350, -4.985214923628407568, -10.07812499938548534 ) ) ;
#22793=CARTESIAN_POINT ( 'NONE',  ( 31.11796464796764994, 7.209453229046482114, 165.6488651237693261 ) ) ;
#22804=DIRECTION ( 'NONE',  ( 1.000000000000000000, 0.000000000000000000, 0.000000000000000000 ) ) ;
#22818=CARTESIAN_POINT ( 'NONE',  ( 20.99999999999999645, 6.928203230275506996, -5.456249998770962506 ) ) ;
#22823=ORIENTED_EDGE ( 'NONE', *, *, #33667, .T. ) ;
#22832=CARTESIAN_POINT ( 'NONE',  ( 36.93740393099094632, -3.604726614523235284, 160.5284327797126025 ) ) ;
#22833=CARTESIAN_POINT ( 'NONE',  ( 26.75643035624999655, 7.049594010296217766E-16, -0.4781249993854874702 ) ) ;
#22835=ORIENTED_EDGE ( 'NONE', *, *, #17058, .F. ) ;
#22837=ORIENTED_EDGE ( 'NONE', *, *, #1304, .F. ) ;
#22838=CARTESIAN_POINT ( 'NONE',  ( 23.99999999999999645, 5.196152422706631135, -6.843749998770965348 ) ) ;
#22839=CARTESIAN_POINT ( 'NONE',  ( 15.24356964375000167, -3.323476615752272600, -3.703124999385450700 ) ) ;
#22841=CARTESIAN_POINT ( 'NONE',  ( 30.59584727662355164, 6.928203230275506996, 159.6810362611256267 ) ) ;
#22849=CARTESIAN_POINT ( 'NONE',  ( 33.92107042726159705, -5.196152422706629359, 163.2673710542620427 ) ) ;
#22853=CARTESIAN_POINT ( 'NONE',  ( 23.87821517812499650, 4.985214923628404904, -3.553124999385481875 ) ) ;
#22857=ADVANCED_FACE ( 'NONE', ( #19494 ), #30669, .T. ) ;
#22862=CARTESIAN_POINT ( 'NONE',  ( 25.01527935017339033, 0.000000000000000000, 50.00000000000000000 ) ) ;
#22863=CARTESIAN_POINT ( 'NONE',  ( 37.01747826964035681, 3.604726614523243278, 161.4436866585844541 ) ) ;
#22874=ORIENTED_EDGE ( 'NONE', *, *, #32055, .T. ) ;
#22875=CARTESIAN_POINT ( 'NONE',  ( 26.99999999999999645, -3.464101615137751278, -3.862499999999976730 ) ) ;
#22876=CARTESIAN_POINT ( 'NONE',  ( 37.18092677073180141, 7.347880794884125653E-16, 166.1065598226053055 ) ) ;
#22877=CARTESIAN_POINT ( 'NONE',  ( 27.65834674205753529, 5.407089921784862696, 161.9237153725250664 ) ) ;
#22879=CARTESIAN_POINT ( 'NONE',  ( 34.54326498017087488, 5.407089921784857367, 168.9817632126399758 ) ) ;
#22890=CARTESIAN_POINT ( 'NONE',  ( 18.12178482187500350, -4.985214923628407568, -9.178124999385472549 ) ) ;
#22896=CARTESIAN_POINT ( 'NONE',  ( 33.95006120609467359, 5.407089921784862696, 162.2014130487530110 ) ) ;
#22904=EDGE_LOOP ( 'NONE', ( #2725, #16014, #1778, #12239 ) ) ;
#22909=CARTESIAN_POINT ( 'NONE',  ( 24.39973176785919406, 3.604726614523236616, 160.4960396437548411 ) ) ;
#22911=CARTESIAN_POINT ( 'NONE',  ( 15.00000000000000000, 3.464101615137752166, -3.581249998770953624 ) ) ;
#22915=CARTESIAN_POINT ( 'NONE',  ( 21.00000000000000355, 0.000000000000000000, 50.00000000000001421 ) ) ;
#22916=( BOUNDED_CURVE ( )  B_SPLINE_CURVE ( 2, ( #8296, #17012, #2594, #25719, #28739, #2778, #34616 ),
 .UNSPECIFIED., .F., .F. ) 
 B_SPLINE_CURVE_WITH_KNOTS ( ( 3, 2, 2, 3 ),
 ( 0.4347826086956526059, 0.4420289855072469520, 0.4492753623188412426, 0.4565217391304355332 ),
 .UNSPECIFIED. ) 
 CURVE ( )  GEOMETRIC_REPRESENTATION_ITEM ( )  RATIONAL_B_SPLINE_CURVE ( ( 0.9999999999999917843, 0.8660254037844469233, 1.000000000000000000, 0.8660254037844387076, 1.000000000000000000, 0.8660254037844243857, 1.000000000000014433 ) ) 
 REPRESENTATION_ITEM ( '' )  );
#22920=EDGE_LOOP ( 'NONE', ( #243, #30344, #25717, #27581 ) ) ;
#22921=CARTESIAN_POINT ( 'NONE',  ( 30.88754665307854452, 7.209453229046475009, 163.0151753906892793 ) ) ;
#22922=CARTESIAN_POINT ( 'NONE',  ( 21.00000000000000000, 6.646953231504538984, -7.453124999385469351 ) ) ;
#22924=CARTESIAN_POINT ( 'NONE',  ( 31.35328515338631306, 7.209453229046482114, 168.3385908086170843 ) ) ;
#22925=CARTESIAN_POINT ( 'NONE',  ( 34.10736582727759725, -5.196152422706635576, 165.3967372202087915 ) ) ;
#22938=CARTESIAN_POINT ( 'NONE',  ( 15.24356964374999990, 0.000000000000000000, -1.603124999385474592 ) ) ;
#22948=EDGE_CURVE ( 'NONE', #21187, #18882, #24134, .T. ) ;
#22950=CARTESIAN_POINT ( 'NONE',  ( 36.79853094953357129, 7.347880794884117764E-16, 161.7357555859521199 ) ) ;
#22951=CARTESIAN_POINT ( 'NONE',  ( 27.99292734389955939, 5.196152422706636465, 164.3506650272002219 ) ) ;
#22954=CARTESIAN_POINT ( 'NONE',  ( 36.90638618107669799, 7.347880794884125653E-16, 162.9685465236163111 ) ) ;
#22959=CARTESIAN_POINT ( 'NONE',  ( 20.99999999999999645, 0.000000000000000000, -8.000000000000000000 ) ) ;
#22961=DIRECTION ( 'NONE',  ( 0.000000000000000000, 0.000000000000000000, 1.000000000000000000 ) ) ;
#22962=CARTESIAN_POINT ( 'NONE',  ( 15.00000000000000000, 0.000000000000000000, -4.950000000000009948 ) ) ;
#22963=CYLINDRICAL_SURFACE ( 'NONE', #26964, 5.999999999999994671 ) ;
#22969=ORIENTED_EDGE ( 'NONE', *, *, #2939, .F. ) ;
#22974=CARTESIAN_POINT ( 'NONE',  ( 23.87821517812499650, 4.985214923628404904, -9.403124999385475746 ) ) ;
#22979=CARTESIAN_POINT ( 'NONE',  ( 24.98313052087628350, 3.604726614523240613, 167.1643179041065252 ) ) ;
#22981=CARTESIAN_POINT ( 'NONE',  ( 24.70365593725145104, 3.464101615137415102, 161.1752605482510035 ) ) ;
#22985=CARTESIAN_POINT ( 'NONE',  ( 28.35571312319377313, 5.196152422706630247, 168.4973254592314618 ) ) ;
#22986=ORIENTED_EDGE ( 'NONE', *, *, #25649, .T. ) ;
#22988=CARTESIAN_POINT ( 'NONE',  ( 20.99999999999999645, -6.928203230275506996, -7.087500000000004796 ) ) ;
#22998=CARTESIAN_POINT ( 'NONE',  ( 37.26590362001809353, -3.464101615137614054, 167.0778496544690768 ) ) ;
#23012=CARTESIAN_POINT ( 'NONE',  ( 30.69144623189632526, 7.209453229046475009, 160.7737373199828426 ) ) ;
#23013=CARTESIAN_POINT ( 'NONE',  ( 18.12178482187500350, -4.985214923628407568, -1.528124999385482852 ) ) ;
#23021=CARTESIAN_POINT ( 'NONE',  ( 21.00000000000000000, 6.928203230275506996, -6.356249998770953979 ) ) ;
#23022=CARTESIAN_POINT ( 'NONE',  ( 23.87821517812499650, 4.985214923628404904, -3.890624999385472460 ) ) ;
#23031=CARTESIAN_POINT ( 'NONE',  ( 24.78209610572492494, 3.464101615137752166, 162.0718357765335611 ) ) ;
#23036=CARTESIAN_POINT ( 'NONE',  ( 18.12178482187500350, -4.985214923628407568, -4.228124999385491023 ) ) ;
#23046=CARTESIAN_POINT ( 'NONE',  ( 30.80420397407610622, 7.209453229046482114, 162.0625642106390671 ) ) ;
#23058=CARTESIAN_POINT ( 'NONE',  ( 21.00000000000000000, 6.928203230275506996, -4.162500000000017408 ) ) ;
#23060=CARTESIAN_POINT ( 'NONE',  ( 36.81484116775207127, -3.604726614523238837, 159.1275339855211257 ) ) ;
#23062=CARTESIAN_POINT ( 'NONE',  ( 28.32999068460662428, 5.407089921784856479, 169.6006407646945604 ) ) ;
#23072=CARTESIAN_POINT ( 'NONE',  ( 20.99999999999999645, -6.928203230275506996, -5.231249998770948650 ) ) ;
#23077=CARTESIAN_POINT ( 'NONE',  ( 27.71064018770612947, -5.407089921784865361, 162.5214321913800859 ) ) ;
#23082=FACE_OUTER_BOUND ( 'NONE', #32609, .T. ) ;
#23090=CARTESIAN_POINT ( 'NONE',  ( 37.60251119283397259, 7.646167579472024665E-16, 168.1306435695252901 ) ) ;
#23091=CARTESIAN_POINT ( 'NONE',  ( 15.00000000000000178, -3.464101615137757051, -3.056249998770964371 ) ) ;
#23093=CARTESIAN_POINT ( 'NONE',  ( 20.99999999999999645, 0.000000000000000000, -8.000000000000000000 ) ) ;
#23102=CARTESIAN_POINT ( 'NONE',  ( 24.52066036092156054, 0.000000000000000000, 161.8782597873571660 ) ) ;
#23103=CARTESIAN_POINT ( 'NONE',  ( 18.12178482187500350, -4.985214923628407568, -7.265624999385461358 ) ) ;
#23105=CARTESIAN_POINT ( 'NONE',  ( 28.12898775289485442, 5.407089921784862696, 167.3031667422204691 ) ) ;
#23106=CARTESIAN_POINT ( 'NONE',  ( 25.28215217963245465, 3.464101615137757051, 167.7875028556105974 ) ) ;
#23111=APPLICATION_CONTEXT ( 'automotive_design' ) ;
#23113=ORIENTED_EDGE ( 'NONE', *, *, #17058, .T. ) ;
#23121=CARTESIAN_POINT ( 'NONE',  ( 26.75643035624999655, -3.323476615752267715, -3.215624999385490401 ) ) ;
#23127=ADVANCED_FACE ( 'NONE', ( #8469 ), #14159, .T. ) ;
#23132=( BOUNDED_CURVE ( )  B_SPLINE_CURVE ( 2, ( #30238, #27018, #1043, #1417, #24180, #12995, #24551 ),
 .UNSPECIFIED., .F., .F. ) 
 B_SPLINE_CURVE_WITH_KNOTS ( ( 3, 2, 2, 3 ),
 ( 0.04347826086956516761, 0.05072463768115921534, 0.05797101449275325613, 0.06521739130434729692 ),
 .UNSPECIFIED. ) 
 CURVE ( )  GEOMETRIC_REPRESENTATION_ITEM ( )  RATIONAL_B_SPLINE_CURVE ( ( 1.000000000000000888, 0.8660254037844378194, 1.000000000000000000, 0.8660254037844387076, 1.000000000000000000, 0.8660254037844484776, 0.9999999999999902300 ) ) 
 REPRESENTATION_ITEM ( '' )  );
#23141=CARTESIAN_POINT ( 'NONE',  ( 26.99999999999999645, 7.347880794884117764E-16, -4.668749998770954868 ) ) ;
#23143=ORIENTED_EDGE ( 'NONE', *, *, #6466, .F. ) ;
#23144=CARTESIAN_POINT ( 'NONE',  ( 25.14491336835161306, 3.604726614523236616, 169.0135043124392951 ) ) ;
#23149=CARTESIAN_POINT ( 'NONE',  ( 15.00000000000000000, 0.000000000000000000, -2.700000000000008171 ) ) ;
#23152=CARTESIAN_POINT ( 'NONE',  ( 21.00000000000000355, 0.000000000000000000, 50.00000000000001421 ) ) ;
#23156=VERTEX_POINT ( 'NONE', #28733 ) ;
#23160=CARTESIAN_POINT ( 'NONE',  ( 15.24356964374999990, 0.000000000000000000, -9.253124999385493155 ) ) ;
#23162=ADVANCED_FACE ( 'NONE', ( #2772 ), #8653, .T. ) ;
#23166=CARTESIAN_POINT ( 'NONE',  ( 24.90795869275643426, 0.000000000000000000, 166.3050999770023850 ) ) ;
#23172=CARTESIAN_POINT ( 'NONE',  ( 25.10896162446820412, 0.000000000000000000, 168.6025739994764479 ) ) ;
#23173=VERTEX_POINT ( 'NONE', #5425 ) ;
#23185=CARTESIAN_POINT ( 'NONE',  ( 25.29849388150488210, -3.464101615137825441, 167.9742893627271485 ) ) ;
#23192=CARTESIAN_POINT ( 'NONE',  ( 30.80175271875777199, -6.928203230275514990, 162.0345462341430505 ) ) ;
#23201=CARTESIAN_POINT ( 'NONE',  ( 15.24356964374999990, 3.323476615752268604, -2.540624999385480809 ) ) ;
#23207=CARTESIAN_POINT ( 'NONE',  ( 20.99999999999999645, -6.646953231504538984, -4.528124999385448213 ) ) ;
#23208=CARTESIAN_POINT ( 'NONE',  ( 30.62526233969377998, 6.928203230275514990, 160.0172519705072318 ) ) ;
#23212=EDGE_CURVE ( 'NONE', #23833, #21861, #29174, .T. ) ;
#23216=CARTESIAN_POINT ( 'NONE',  ( 27.78048522105927987, -5.196152422706632912, 161.9224404518259064 ) ) ;
#23220=CARTESIAN_POINT ( 'NONE',  ( 26.75643035624999655, 7.049594010296217766E-16, -3.628124999385473615 ) ) ;
#23229=CARTESIAN_POINT ( 'NONE',  ( 36.97825818540390941, 3.604726614523243278, 160.9953990444431611 ) ) ;
#23238=CARTESIAN_POINT ( 'NONE',  ( 20.99999999999999645, 6.928203230275506996, -7.706249998770941190 ) ) ;
#23243=CARTESIAN_POINT ( 'NONE',  ( 21.00000000000000000, 6.928203230275506996, -5.512500000000003730 ) ) ;
#23245=DIRECTION ( 'NONE',  ( 0.08715574274765150453, 0.000000000000000000, 0.9961946980917461003 ) ) ;
#23246=CARTESIAN_POINT ( 'NONE',  ( 15.00000000000000000, 0.000000000000000000, -6.693749998770953447 ) ) ;
#23248=CARTESIAN_POINT ( 'NONE',  ( 25.03378979634835488, -3.604726614523240613, 167.7433560723723076 ) ) ;
#23250=CARTESIAN_POINT ( 'NONE',  ( 23.99999999999999645, 5.196152422706631135, -0.9937499987709430549 ) ) ;
#23255=CARTESIAN_POINT ( 'NONE',  ( 24.99999999999999289, 0.000000000000000000, 49.65004534589634488 ) ) ;
#23258=CARTESIAN_POINT ( 'NONE',  ( 26.75643035624999655, 3.323476615752271712, -7.078124999385466687 ) ) ;
#23260=CARTESIAN_POINT ( 'NONE',  ( 20.00041244883536606, 5.668978318349186196, -10.25260146540740003 ) ) ;
#23264=CARTESIAN_POINT ( 'NONE',  ( 37.39010055343325689, 3.464101615137755275, 168.4974270992498475 ) ) ;
#23273=VERTEX_POINT ( 'NONE', #31955 ) ;
#23278=CARTESIAN_POINT ( 'NONE',  ( 28.25972136701633630, -5.407089921784865361, 168.7974587893581315 ) ) ;
#23279=CARTESIAN_POINT ( 'NONE',  ( 21.00000000000000000, 6.928203230275506996, -2.756249998770956111 ) ) ;
#23288=ORIENTED_EDGE ( 'NONE', *, *, #14244, .F. ) ;
#23289=CARTESIAN_POINT ( 'NONE',  ( 30.90715669519676467, -7.209453229046475009, 163.2393191977599258 ) ) ;
#23290=CARTESIAN_POINT ( 'NONE',  ( 21.00000000000000000, 6.646953231504538984, -7.903124999385464200 ) ) ;
#23292=CARTESIAN_POINT ( 'NONE',  ( 37.37045902776835504, 3.604726614523243278, 165.4782751858560061 ) ) ;
#23293=CARTESIAN_POINT ( 'NONE',  ( 25.28542051998549667, 0.000000000000000000, 167.8248601567890432 ) ) ;
#23305=CARTESIAN_POINT ( 'NONE',  ( 26.75643035624999655, 3.323476615752271712, -4.040624999385487470 ) ) ;
#23316=CYLINDRICAL_SURFACE ( 'NONE', #1636, 6.000000000000001776 ) ;
#23319=CARTESIAN_POINT ( 'NONE',  ( 24.96839150574053434, 3.464101615137542112, 164.2012019424803100 ) ) ;
#23325=CARTESIAN_POINT ( 'NONE',  ( 25.14818170870464797, 0.000000000000000000, 169.0508616136177409 ) ) ;
#23327=FACE_OUTER_BOUND ( 'NONE', #5754, .T. ) ;
#23330=CARTESIAN_POINT ( 'NONE',  ( 15.00000000000000000, 0.000000000000000000, -3.599999999999992095 ) ) ;
#23341=CARTESIAN_POINT ( 'NONE',  ( 26.75643035624999655, -3.323476615752267715, -9.965624999385457983 ) ) ;
#23346=CARTESIAN_POINT ( 'NONE',  ( 31.21601485855876135, -7.209453229046482114, 166.7695841591225587 ) ) ;
#23347=VECTOR ( 'NONE', #30998, 1000.000000000000000 ) ;
#23351=FACE_OUTER_BOUND ( 'NONE', #36983, .T. ) ;
#23354=CARTESIAN_POINT ( 'NONE',  ( 37.64990212795299840, 3.604726614523238837, 168.6723244366126551 ) ) ;
#23369=DIRECTION ( 'NONE',  ( 0.9961946980917462113, 0.000000000000000000, -0.08715574274765118534 ) ) ;
#23372=CARTESIAN_POINT ( 'NONE',  ( 37.30839204460733782, 7.347880794884117764E-16, 167.5634945697888440 ) ) ;
#23382=CARTESIAN_POINT ( 'NONE',  ( 27.48022219281702405, -5.407089921784859143, 159.8877424583000391 ) ) ;
#23383=CARTESIAN_POINT ( 'NONE',  ( 26.75643035624999655, -3.323476615752267715, -2.765624999385494220 ) ) ;
#23386=EDGE_LOOP ( 'NONE', ( #16126, #35261, #20165, #32798 ) ) ;
#23388=ORIENTED_EDGE ( 'NONE', *, *, #27471, .F. ) ;
#23389=CARTESIAN_POINT ( 'NONE',  ( 15.24356964375000167, -3.323476615752272600, -4.153124999385478411 ) ) ;
#23391=( BOUNDED_CURVE ( )  B_SPLINE_CURVE ( 2, ( #20104, #35049, #22951, #11931, #14598, #8722, #8905 ),
 .UNSPECIFIED., .F., .F. ) 
 B_SPLINE_CURVE_WITH_KNOTS ( ( 3, 2, 2, 3 ),
 ( 0.5217391304347818171, 0.5289855072463759411, 0.5362318840579700652, 0.5434782608695640782 ),
 .UNSPECIFIED. ) 
 CURVE ( )  GEOMETRIC_REPRESENTATION_ITEM ( )  RATIONAL_B_SPLINE_CURVE ( ( 1.000000000000014433, 0.8660254037844243857, 1.000000000000000000, 0.8660254037844387076, 1.000000000000000000, 0.8660254037844592467, 0.9999999999999794609 ) ) 
 REPRESENTATION_ITEM ( '' )  );
#23398=CARTESIAN_POINT ( 'NONE',  ( 30.75272761356932705, 6.928203230275506996, 161.4741867176907988 ) ) ;
#23402=CARTESIAN_POINT ( 'NONE',  ( 15.24356964374999990, 3.323476615752268604, -3.440624999385503813 ) ) ;
#23403=CARTESIAN_POINT ( 'NONE',  ( 26.99999999999999645, 7.347880794884117764E-16, -0.6750000000000089262 ) ) ;
#23410=CARTESIAN_POINT ( 'NONE',  ( 18.00000000000000000, 5.196152422706630247, -5.868749998770961263 ) ) ;
#23411=CARTESIAN_POINT ( 'NONE',  ( 24.47653776615555898, 0.000000000000000000, 161.3739362214482469 ) ) ;
#23424=CARTESIAN_POINT ( 'NONE',  ( 18.00000000000000000, 5.196152422706630247, -7.725000000000009415 ) ) ;
#23428=CARTESIAN_POINT ( 'NONE',  ( 37.36882485759181804, -3.604726614523235284, 165.4595965352667690 ) ) ;
#23433=ORIENTED_EDGE ( 'NONE', *, *, #36224, .F. ) ;
#23434=CARTESIAN_POINT ( 'NONE',  ( 36.94233792496062563, -3.464101615137448409, 163.3794768365791015 ) ) ;
#23437=CARTESIAN_POINT ( 'NONE',  ( 26.75643035624999655, 7.049594010296217766E-16, -7.565624999385455851 ) ) ;
#23444=CARTESIAN_POINT ( 'NONE',  ( 27.51453976652391376, -5.407089921784865361, 160.2799941206736776 ) ) ;
#23456=CARTESIAN_POINT ( 'NONE',  ( 15.00000000000000000, 0.000000000000000000, -1.293749998770965526 ) ) ;
#23457=CARTESIAN_POINT ( 'NONE',  ( 37.64173127707041289, 7.646167579472024665E-16, 168.5789311836665831 ) ) ;
#23458=CARTESIAN_POINT ( 'NONE',  ( 15.00000000000000178, -3.464101615137757051, -1.706249998770944964 ) ) ;
#23463=DIRECTION ( 'NONE',  ( 0.9961946980917462113, 0.000000000000000000, -0.08715574274765118534 ) ) ;
#23467=CARTESIAN_POINT ( 'NONE',  ( 20.99999999999999645, 0.000000000000000000, -8.000000000000000000 ) ) ;
#23469=CARTESIAN_POINT ( 'NONE',  ( 24.40300010821222898, 0.000000000000000000, 160.5333969449332869 ) ) ;
#23470=CARTESIAN_POINT ( 'NONE',  ( 23.87821517812500005, -4.985214923628404016, -8.540624999385460825 ) ) ;
#23472=CARTESIAN_POINT ( 'NONE',  ( 31.01991443737654208, -7.209453229046482114, 164.5281460884161504 ) ) ;
#23473=CARTESIAN_POINT ( 'NONE',  ( 36.94887460566616966, 3.464101615137759271, 163.4541914389360215 ) ) ;
#23481=ORIENTED_EDGE ( 'NONE', *, *, #22553, .T. ) ;
#23485=EDGE_CURVE ( 'NONE', #4869, #7912, #35710, .T. ) ;
#23486=CARTESIAN_POINT ( 'NONE',  ( 26.75643035624999655, 7.049594010296217766E-16, -3.628124999385473615 ) ) ;
#23500=CARTESIAN_POINT ( 'NONE',  ( 15.00000000000031797, 3.464101615137936019, -7.181249998770955045 ) ) ;
#23501=CARTESIAN_POINT ( 'NONE',  ( 36.67106567565804198, 7.347880794884125653E-16, 160.2788208387686097 ) ) ;
#23506=CARTESIAN_POINT ( 'NONE',  ( 26.99999999999999645, 7.347880794884117764E-16, -0.2250000000000029754 ) ) ;
#23514=CARTESIAN_POINT ( 'NONE',  ( 37.64990212795299129, 3.604726614523238837, 168.6723244366126551 ) ) ;
#23516=CARTESIAN_POINT ( 'NONE',  ( 18.12178482187500350, -4.985214923628407568, -1.415624999385467486 ) ) ;
#23528=CARTESIAN_POINT ( 'NONE',  ( 15.24356964374999990, 0.000000000000000000, -8.353124999385480365 ) ) ;
#23536=CARTESIAN_POINT ( 'NONE',  ( 31.15718473220409379, 7.209453229046482114, 166.0971527379105908 ) ) ;
#23541=EDGE_CURVE ( 'NONE', #34897, #18997, #36339, .T. ) ;
#23543=CARTESIAN_POINT ( 'NONE',  ( 25.06317337608639306, -3.464101615137925805, 165.2845636778794187 ) ) ;
#23544=CARTESIAN_POINT ( 'NONE',  ( 28.32999068460662428, 5.407089921784856479, 169.6006407646945604 ) ) ;
#23546=CARTESIAN_POINT ( 'NONE',  ( 25.32464060422194052, 0.000000000000000000, 168.2731477709303363 ) ) ;
#23551=( BOUNDED_CURVE ( )  B_SPLINE_CURVE ( 2, ( #26514, #15534, #32579, #544, #15343, #26897, #21416 ),
 .UNSPECIFIED., .F., .F. ) 
 B_SPLINE_CURVE_WITH_KNOTS ( ( 3, 2, 2, 3 ),
 ( 0.2391304347826081200, 0.2463768115942023829, 0.2536231884057966179, 0.2608695652173908530 ),
 .UNSPECIFIED. ) 
 CURVE ( )  GEOMETRIC_REPRESENTATION_ITEM ( )  RATIONAL_B_SPLINE_CURVE ( ( 1.000000000000010658, 0.8660254037844279384, 1.000000000000000000, 0.8660254037844387076, 1.000000000000000000, 0.8660254037844469233, 0.9999999999999917843 ) ) 
 REPRESENTATION_ITEM ( '' )  );
#23554=ORIENTED_EDGE ( 'NONE', *, *, #20519, .F. ) ;
#23562=CARTESIAN_POINT ( 'NONE',  ( 31.41946904558886544, 6.928203230275506996, 169.0950761580926383 ) ) ;
#23566=ORIENTED_EDGE ( 'NONE', *, *, #14456, .T. ) ;
#23571=CARTESIAN_POINT ( 'NONE',  ( 36.90472052746056875, 3.604726614523238837, 160.1548597679282295 ) ) ;
#23572=CARTESIAN_POINT ( 'NONE',  ( 26.75643035624999655, 7.049594010296217766E-16, -1.378124999385471616 ) ) ;
#23578=CARTESIAN_POINT ( 'NONE',  ( 23.87821517812499650, 4.985214923628404904, -5.240624999385462779 ) ) ;
#23579=CARTESIAN_POINT ( 'NONE',  ( 37.02404643378602600, 7.347880794884125653E-16, 164.3134093660401618 ) ) ;
#23586=CARTESIAN_POINT ( 'NONE',  ( 27.72819177541068214, 5.196152422706630247, 161.3247236329709153 ) ) ;
#23590=CARTESIAN_POINT ( 'NONE',  ( 15.24356964374999990, 0.000000000000000000, -7.453124999385495997 ) ) ;
#23591=CARTESIAN_POINT ( 'NONE',  ( 26.99999999999999289, 0.000000000000000000, -8.000000000000000000 ) ) ;
#23598=CARTESIAN_POINT ( 'NONE',  ( 24.43731768191911513, 0.000000000000000000, 160.9256486073069539 ) ) ;
#23610=CARTESIAN_POINT ( 'NONE',  ( 21.00000000000000000, 6.928203230275506996, -8.212500000000009237 ) ) ;
#23616=CARTESIAN_POINT ( 'NONE',  ( 28.13389026342440857, 5.407089921784856479, 167.3592026939881237 ) ) ;
#23621=EDGE_LOOP ( 'NONE', ( #35446, #416, #1419, #6986, #24555, #17230, #22050, #16774, #19631, #1591, #12597, #30380, #20774, #5823, #8860, #22238, #28568, #20934, #34295, #30576, #19166, #16498, #1283, #3332, #33684, #14685, #32550, #27929, #6701, #30149, #25388, #1558, #32845, #24184, #13686, #33388, #33086, #23566, #33126, #37400, #18308, #3755, #11679, #7964, #33768, #22516, #13159, #32130 ) ) ;
#23624=ADVANCED_FACE ( 'NONE', ( #24449 ), #1876, .T. ) ;
#23627=CARTESIAN_POINT ( 'NONE',  ( 18.12178482187500350, -4.985214923628407568, -6.365624999385477878 ) ) ;
#23628=AXIS2_PLACEMENT_3D ( 'NONE', #608, #18647, #1372 ) ;
#23636=CARTESIAN_POINT ( 'NONE',  ( 33.74088742350031822, -5.407089921784861808, 159.8105457733328478 ) ) ;
#23649=CARTESIAN_POINT ( 'NONE',  ( 22.74267999994772538, 5.498826287438556726, -8.000000000000001776 ) ) ;
#23650=CARTESIAN_POINT ( 'NONE',  ( 25.10079077358561150, 3.604726614523240613, 168.5091807465304043 ) ) ;
#23651=CARTESIAN_POINT ( 'NONE',  ( 21.00000000000000000, -6.928203230275506996, -2.531249998770942700 ) ) ;
#23660=CARTESIAN_POINT ( 'NONE',  ( 36.81974367828161121, -3.604726614523235284, 159.1835699372888087 ) ) ;
#23661=CARTESIAN_POINT ( 'NONE',  ( 18.12178482187499640, 4.985214923628404904, -9.215624999385468641 ) ) ;
#23663=CARTESIAN_POINT ( 'NONE',  ( 24.79029844004710625, 0.000000000000000000, 164.9602371345785343 ) ) ;
#23664=CARTESIAN_POINT ( 'NONE',  ( 34.02892565880470954, -5.196152422706635576, 164.5001619919262055 ) ) ;
#23675=CARTESIAN_POINT ( 'NONE',  ( 18.12178482187500350, -4.985214923628407568, -5.128124999385475391 ) ) ;
#23684=DIRECTION ( 'NONE',  ( 0.9961946980917461003, 0.000000000000000000, -0.08715574274765142126 ) ) ;
#23688=DIRECTION ( 'NONE',  ( 0.08715574274765150453, 0.000000000000000000, 0.9961946980917461003 ) ) ;
#23689=CARTESIAN_POINT ( 'NONE',  ( 37.10082094864278446, 3.604726614523238837, 162.3962978386346663 ) ) ;
#23702=ORIENTED_EDGE ( 'NONE', *, *, #15057, .F. ) ;
#23704=CARTESIAN_POINT ( 'NONE',  ( 24.94881294716940090, 3.604726614523236616, 166.7720662417328583 ) ) ;
#23705=CARTESIAN_POINT ( 'NONE',  ( 23.87821517812500005, -4.985214923628404016, -4.040624999385455496 ) ) ;
#23709=CARTESIAN_POINT ( 'NONE',  ( 37.10902328307243181, -3.464101615137552326, 165.2846991979039046 ) ) ;
#23717=CARTESIAN_POINT ( 'NONE',  ( 18.12178482187499640, 4.985214923628404904, -1.115624999385472771 ) ) ;
#23720=CARTESIAN_POINT ( 'NONE',  ( 15.00000000000000000, 0.000000000000000000, -8.043749998770943321 ) ) ;
#23726=CARTESIAN_POINT ( 'NONE',  ( 31.05913452161298949, -7.209453229046482114, 164.9764337025573866 ) ) ;
#23732=CARTESIAN_POINT ( 'NONE',  ( 34.22950430627932406, 5.407089921784857367, 165.3954622995096599 ) ) ;
#23751=CARTESIAN_POINT ( 'NONE',  ( 30.82136276087599214, 6.928203230275514990, 162.2586900412136686 ) ) ;
#23760=CARTESIAN_POINT ( 'NONE',  ( 18.12178482187500350, -4.985214923628407568, -2.878124999385472726 ) ) ;
#23765=CARTESIAN_POINT ( 'NONE',  ( 15.24356964374999990, 0.000000000000000000, -4.190624999385467397 ) ) ;
#23775=CARTESIAN_POINT ( 'NONE',  ( 33.80341017455227615, -5.196152422706629359, 161.9225082118381920 ) ) ;
#23780=CARTESIAN_POINT ( 'NONE',  ( 26.75643035624999655, -3.323476615752267271, -7.715624999385478411 ) ) ;
#23784=CARTESIAN_POINT ( 'NONE',  ( 26.99999999999985789, -3.464101615137830770, -0.6562499987709674576 ) ) ;
#23788=CARTESIAN_POINT ( 'NONE',  ( 24.40136593803570975, -3.604726614523244610, 160.5147182943441067 ) ) ;
#23796=( BOUNDED_CURVE ( )  B_SPLINE_CURVE ( 2, ( #487, #12053, #3526, #32515, #24003, #671, #18134 ),
 .UNSPECIFIED., .F., .F. ) 
 B_SPLINE_CURVE_WITH_KNOTS ( ( 3, 2, 2, 3 ),
 ( 0.2826086956521750015, 0.2898550724637684040, 0.2971014492753618064, 0.3043478260869552088 ),
 .UNSPECIFIED. ) 
 CURVE ( )  GEOMETRIC_REPRESENTATION_ITEM ( )  RATIONAL_B_SPLINE_CURVE ( ( 0.9999999999999794609, 0.8660254037844592467, 1.000000000000000000, 0.8660254037844387076, 1.000000000000000000, 0.8660254037844633546, 0.9999999999999753530 ) ) 
 REPRESENTATION_ITEM ( '' )  );
#23801=CARTESIAN_POINT ( 'NONE',  ( 26.99999999999999645, 3.464101615137755275, -6.037499999999993427 ) ) ;
#23805=CARTESIAN_POINT ( 'NONE',  ( 37.37536153829788077, 3.604726614523238837, 165.5343111376236607 ) ) ;
#23811=CARTESIAN_POINT ( 'NONE',  ( 26.99999999999999645, 7.347880794884117764E-16, -2.475000000000004974 ) ) ;
#23815=CARTESIAN_POINT ( 'NONE',  ( 21.00000000000000000, 6.646953231504538984, -6.553124999385445903 ) ) ;
#23821=DIRECTION ( 'NONE',  ( 0.9961946980917462113, 0.000000000000000000, -0.08715574274765118534 ) ) ;
#23822=CARTESIAN_POINT ( 'NONE',  ( 37.38356387272718706, -3.464101615137751278, 168.4227124968929559 ) ) ;
#23826=VECTOR ( 'NONE', #20719, 1000.000000000000000 ) ;
#23828=CARTESIAN_POINT ( 'NONE',  ( 18.12178482187500350, -4.985214923628407568, -0.6281249993854709501 ) ) ;
#23832=EDGE_CURVE ( 'NONE', #20636, #6128, #2806, .T. ) ;
#23833=VERTEX_POINT ( 'NONE', #22543 ) ;
#23837=CARTESIAN_POINT ( 'NONE',  ( 37.48158259977161322, -3.604726614523238837, 166.7484234259230220 ) ) ;
#23839=( BOUNDED_CURVE ( )  B_SPLINE_CURVE ( 2, ( #25503, #2190, #19468, #25318, #25691, #28897, #26057 ),
 .UNSPECIFIED., .F., .F. ) 
 B_SPLINE_CURVE_WITH_KNOTS ( ( 3, 2, 2, 3 ),
 ( 0.6304347826086960094, 0.6376811594202902445, 0.6449275362318845906, 0.6521739130434789367 ),
 .UNSPECIFIED. ) 
 CURVE ( )  GEOMETRIC_REPRESENTATION_ITEM ( )  RATIONAL_B_SPLINE_CURVE ( ( 0.9999999999999938938, 0.8660254037844448138, 1.000000000000000000, 0.8660254037844387076, 1.000000000000000000, 0.8660254037844263841, 1.000000000000012212 ) ) 
 REPRESENTATION_ITEM ( '' )  );
#23852=CARTESIAN_POINT ( 'NONE',  ( 36.90472052746056875, 3.604726614523238837, 160.1548597679282295 ) ) ;
#23853=CARTESIAN_POINT ( 'NONE',  ( 26.99999999999999645, 7.347880794884117764E-16, -0.6750000000000089262 ) ) ;
#23855=CARTESIAN_POINT ( 'NONE',  ( 34.14616162727688931, 5.407089921784862696, 164.4428511194594478 ) ) ;
#23856=CARTESIAN_POINT ( 'NONE',  ( 27.88834045260238526, -5.196152422706638241, 163.1552313894900976 ) ) ;
#23862=ORIENTED_EDGE ( 'NONE', *, *, #36066, .T. ) ;
#23866=CARTESIAN_POINT ( 'NONE',  ( 21.00000000000000000, 6.646953231504538984, -4.415624999385457272 ) ) ;
#23874=AXIS2_PLACEMENT_3D ( 'NONE', #28699, #8988, #14674 ) ;
#23883=CARTESIAN_POINT ( 'NONE',  ( 27.93778984224218931, 5.407089921784856479, 165.1177646232817153 ) ) ;
#23887=CARTESIAN_POINT ( 'NONE',  ( 26.99999999999999645, 7.347880794884117764E-16, -7.424999999999987388 ) ) ;
#23895=CARTESIAN_POINT ( 'NONE',  ( 37.45053336641773711, 7.646167579472015790E-16, 166.3935290647278009 ) ) ;
#23896=CARTESIAN_POINT ( 'NONE',  ( 21.00000000000000000, 6.646953231504538984, -2.053124999385488092 ) ) ;
#23898=DIRECTION ( 'NONE',  ( 0.08715574274765150453, 0.000000000000000000, 0.9961946980917461003 ) ) ;
#23900=CARTESIAN_POINT ( 'NONE',  ( 18.00000000000000355, -5.196152422706632912, -7.518749998770946519 ) ) ;
#23908=CARTESIAN_POINT ( 'NONE',  ( 18.12178482187500350, -4.985214923628407568, -0.9656249993854615354 ) ) ;
#23910=CARTESIAN_POINT ( 'NONE',  ( 24.00000000000000000, -5.196152422706629359, -7.893749998770960730 ) ) ;
#23912=CARTESIAN_POINT ( 'NONE',  ( 20.99999999999999645, 0.000000000000000000, -8.000000000000000000 ) ) ;
#23917=CARTESIAN_POINT ( 'NONE',  ( 34.13308826586474254, -5.407089921784861808, 164.2934219147456929 ) ) ;
#23920=( NAMED_UNIT ( * ) PLANE_ANGLE_UNIT ( ) SI_UNIT ( $, .RADIAN. ) );
#23924=CARTESIAN_POINT ( 'NONE',  ( 37.41458162253433528, 3.604726614523238837, 165.9825987517649253 ) ) ;
#23933=VERTEX_POINT ( 'NONE', #28220 ) ;
#23940=CYLINDRICAL_SURFACE ( 'NONE', #14410, 5.999999999999994671 ) ;
#23941=CARTESIAN_POINT ( 'NONE',  ( 25.17923094205850276, 3.604726614523240613, 169.4057559748129336 ) ) ;
#23945=VERTEX_POINT ( 'NONE', #19713 ) ;
#23951=CARTESIAN_POINT ( 'NONE',  ( 23.87821517812500005, -4.985214923628404016, -4.603124999385476812 ) ) ;
#23957=CARTESIAN_POINT ( 'NONE',  ( 18.12178482187499640, 4.985214923628404904, -6.065624999385454963 ) ) ;
#23965=CARTESIAN_POINT ( 'NONE',  ( 27.66282496834995186, -5.196152422706632912, 160.5775776094020557 ) ) ;
#23969=EDGE_CURVE ( 'NONE', #20636, #13931, #22676, .T. ) ;
#23970=CARTESIAN_POINT ( 'NONE',  ( 23.87821517812500005, -4.985214923628404016, -7.303124999385484983 ) ) ;
#23977=MECHANICAL_DESIGN_GEOMETRIC_PRESENTATION_REPRESENTATION('',(#26392),#10659);
#23979=CARTESIAN_POINT ( 'NONE',  ( 30.64732363713033081, 7.209453229046482114, 160.2694137540738950 ) ) ;
#23992=CARTESIAN_POINT ( 'NONE',  ( 26.99999999999999645, 3.464101615137755275, -6.937499999999985789 ) ) ;
#23993=CARTESIAN_POINT ( 'NONE',  ( 18.00000000000000355, -5.196152422706632912, -4.425000000000012257 ) ) ;
#23995=CARTESIAN_POINT ( 'NONE',  ( 31.12286715849720409, 7.209453229046475009, 165.7049010755369807 ) ) ;
#24003=CARTESIAN_POINT ( 'NONE',  ( 18.00000000000000355, -5.196152422706632912, -3.468749998770948029 ) ) ;
#24005=CARTESIAN_POINT ( 'NONE',  ( 23.87821517812499650, 4.985214923628404904, -6.590624999385480187 ) ) ;
#24013=CARTESIAN_POINT ( 'NONE',  ( 28.39493320743021698, 5.196152422706630247, 168.9456130733727548 ) ) ;
#24025=CARTESIAN_POINT ( 'NONE',  ( 15.00000000000000000, 0.000000000000000000, -6.299999999999999822 ) ) ;
#24027=CARTESIAN_POINT ( 'NONE',  ( 31.21601485855876135, -7.209453229046482114, 166.7695841591225587 ) ) ;
#24029=CARTESIAN_POINT ( 'NONE',  ( 29.51984228635672380, 5.908847293266075162, 159.3365288790247121 ) ) ;
#24038=CARTESIAN_POINT ( 'NONE',  ( 33.70656984979341786, -5.407089921784855591, 159.4182941109592093 ) ) ;
#24039=CARTESIAN_POINT ( 'NONE',  ( 23.87821517812499650, 4.985214923628404904, -9.290624999385460825 ) ) ;
#24041=CARTESIAN_POINT ( 'NONE',  ( 24.95044711734591658, -3.604726614523244610, 166.7907448923220954 ) ) ;
#24043=CARTESIAN_POINT ( 'NONE',  ( 34.00277893598041601, 5.196152422706637353, 164.2013035824986957 ) ) ;
#24053=CARTESIAN_POINT ( 'NONE',  ( 23.87821517812500005, -4.985214923628404016, -5.503124999385489602 ) ) ;
#24064=CARTESIAN_POINT ( 'NONE',  ( 18.00000000000000355, -5.196152422706632912, -3.074999999999994404 ) ) ;
#24067=CARTESIAN_POINT ( 'NONE',  ( 14.99999999999954348, 3.464101615137491930, -1.781249998770933374 ) ) ;
#24068=CARTESIAN_POINT ( 'NONE',  ( 31.04442699002431993, 7.209453229046475009, 164.8083258472544230 ) ) ;
#24079=VERTEX_POINT ( 'NONE', #17976 ) ;
#24080=CARTESIAN_POINT ( 'NONE',  ( 31.29935753756119965, -7.209453229046475009, 167.7221953391727709 ) ) ;
#24081=CARTESIAN_POINT ( 'NONE',  ( 15.24356964375000167, -3.323476615752272600, -2.353124999385463489 ) ) ;
#24084=LINE ( 'NONE', #29380, #1538 ) ;
#24093=CARTESIAN_POINT ( 'NONE',  ( 26.75643035624999655, 3.323476615752271712, -2.578124999385477345 ) ) ;
#24095=EDGE_CURVE ( 'NONE', #1464, #31223, #35941, .T. ) ;
#24096=CARTESIAN_POINT ( 'NONE',  ( 26.99999999999999645, 7.347880794884117764E-16, -8.268749998770946519 ) ) ;
#24100=ORIENTED_EDGE ( 'NONE', *, *, #19130, .T. ) ;
#24104=CARTESIAN_POINT ( 'NONE',  ( 27.81522707900330715, 5.407089921784862696, 163.7168658290902101 ) ) ;
#24109=CARTESIAN_POINT ( 'NONE',  ( 26.99999999999999289, 0.000000000000000000, -8.000000000000000000 ) ) ;
#24111=( BOUNDED_CURVE ( )  B_SPLINE_CURVE ( 2, ( #16122, #992, #12568, #34101, #28230, #31263, #4732 ),
 .UNSPECIFIED., .F., .F. ) 
 B_SPLINE_CURVE_WITH_KNOTS ( ( 3, 2, 2, 3 ),
 ( 0.4347826086956515512, 0.4420289855072456753, 0.4492753623188397993, 0.4565217391304338679 ),
 .UNSPECIFIED. ) 
 CURVE ( )  GEOMETRIC_REPRESENTATION_ITEM ( )  RATIONAL_B_SPLINE_CURVE ( ( 1.000000000000011102, 0.8660254037844272723, 1.000000000000000000, 0.8660254037844387076, 1.000000000000000000, 0.8660254037844551389, 0.9999999999999835687 ) ) 
 REPRESENTATION_ITEM ( '' )  );
#24113=CARTESIAN_POINT ( 'NONE',  ( 37.33614145406145468, 3.604726614523238837, 165.0860235234823392 ) ) ;
#24115=CARTESIAN_POINT ( 'NONE',  ( 25.32790894457507846, -3.464101615137821888, 168.3105050721087537 ) ) ;
#24130=DIRECTION ( 'NONE',  ( 1.000000000000000000, 0.000000000000000000, 0.000000000000000000 ) ) ;
#24134=B_SPLINE_CURVE_WITH_KNOTS ( 'NONE', 3,
 ( #10566, #5062, #24784, #19119 ),
 .UNSPECIFIED., .F., .F.,
 ( 4, 4 ),
 ( 0.000000000000000000, 1.000000000000000000 ),
 .UNSPECIFIED. ) ;
#24135=DIRECTION ( 'NONE',  ( 0.000000000000000000, 0.000000000000000000, 1.000000000000000000 ) ) ;
#24141=CARTESIAN_POINT ( 'NONE',  ( 26.75643035624999655, 3.323476615752271712, -4.040624999385487470 ) ) ;
#24144=CARTESIAN_POINT ( 'NONE',  ( 26.99999999999999645, 7.347880794884117764E-16, -6.975000000000008527 ) ) ;
#24149=CARTESIAN_POINT ( 'NONE',  ( 24.63175244948523002, -3.464101615137757051, 160.3533999223253375 ) ) ;
#24153=CARTESIAN_POINT ( 'NONE',  ( 26.75643035624999655, 7.049594010296217766E-16, -6.778124999385487293 ) ) ;
#24161=CARTESIAN_POINT ( 'NONE',  ( 33.70166733926387082, -5.407089921784861808, 159.3622581591915548 ) ) ;
#24165=CARTESIAN_POINT ( 'NONE',  ( 24.58926402489574770, 0.000000000000000000, 159.8677550070055702 ) ) ;
#24166=CARTESIAN_POINT ( 'NONE',  ( 26.99999999999958078, -3.464101615137992862, -1.106249998770966636 ) ) ;
#24175=CARTESIAN_POINT ( 'NONE',  ( 24.00000000000000000, -5.196152422706629359, -7.500000000000007105 ) ) ;
#24179=CARTESIAN_POINT ( 'NONE',  ( 37.21521286099908110, 7.646167579472015790E-16, 163.7038033798800711 ) ) ;
#24180=CARTESIAN_POINT ( 'NONE',  ( 34.39497977834484743, 5.196152422706637353, 168.6841797239115976 ) ) ;
#24184=ORIENTED_EDGE ( 'NONE', *, *, #14345, .T. ) ;
#24186=DIRECTION ( 'NONE',  ( 0.000000000000000000, 0.000000000000000000, 1.000000000000000000 ) ) ;
#24187=CARTESIAN_POINT ( 'NONE',  ( 29.54925929127992745, 5.908847637349538218, 159.6727443940304738 ) ) ;
#24188=LINE ( 'NONE', #6183, #772 ) ;
#24189=CARTESIAN_POINT ( 'NONE',  ( 18.12178482187499640, 4.985214923628404904, -8.315624999385457627 ) ) ;
#24192=CARTESIAN_POINT ( 'NONE',  ( 24.78863278643148149, -3.464101615138032830, 162.1465503788903959 ) ) ;
#24193=EDGE_CURVE ( 'NONE', #24223, #31540, #18352, .T. ) ;
#24197=CARTESIAN_POINT ( 'NONE',  ( 25.33444562538816669, 0.000000000000000000, 168.3852196756899957 ) ) ;
#24201=ADVANCED_FACE ( 'NONE', ( #29901 ), #27059, .F. ) ;
#24202=CARTESIAN_POINT ( 'NONE',  ( 18.12178482187499640, 4.985214923628404904, -0.3281249993854762348 ) ) ;
#24208=CARTESIAN_POINT ( 'NONE',  ( 20.99999999999999645, -6.928203230275506996, -6.187500000000013323 ) ) ;
#24210=CARTESIAN_POINT ( 'NONE',  ( 31.29445502703164905, -7.209453229046482114, 167.6661593874051164 ) ) ;
#24223=VERTEX_POINT ( 'NONE', #12655 ) ;
#24225=CARTESIAN_POINT ( 'NONE',  ( 21.00000000000000000, 6.646953231504538984, -9.253124999385450522 ) ) ;
#24228=EDGE_CURVE ( 'NONE', #27974, #9824, #27621, .T. ) ;
#24229=CARTESIAN_POINT ( 'NONE',  ( 24.75434669616370442, -3.604726614523244610, 164.5493068216156303 ) ) ;
#24230=CARTESIAN_POINT ( 'NONE',  ( 27.99292734389955939, 5.196152422706636465, 164.3506650272002219 ) ) ;
#24238=CARTESIAN_POINT ( 'NONE',  ( 24.98146486726017912, 0.000000000000000000, 164.3506311484184437 ) ) ;
#24239=EDGE_CURVE ( 'NONE', #8675, #22401, #2289, .T. ) ;
#24241=CARTESIAN_POINT ( 'NONE',  ( 26.75643035624999655, 3.323476615752271712, -6.290624999385498128 ) ) ;
#24246=CARTESIAN_POINT ( 'NONE',  ( 24.93243976185750554, 0.000000000000000000, 163.7902716295174912 ) ) ;
#24258=CARTESIAN_POINT ( 'NONE',  ( 30.96598682155142868, 7.209453229046475009, 163.9117506189718370 ) ) ;
#24269=CARTESIAN_POINT ( 'NONE',  ( 31.24052741120653209, 7.209453229046475009, 167.0497639179608313 ) ) ;
#24270=CARTESIAN_POINT ( 'NONE',  ( 18.12178482187500350, -4.985214923628407568, -3.215624999385463312 ) ) ;
#24273=DIRECTION ( 'NONE',  ( 0.9961946980917462113, 0.000000000000000000, -0.08715574274765118534 ) ) ;
#24283=CARTESIAN_POINT ( 'NONE',  ( 21.00000000000000000, 6.646953231504538984, -2.503124999385450966 ) ) ;
#24285=CARTESIAN_POINT ( 'NONE',  ( 19.95811728174978228, 5.908847637349563087, -10.39322646479281254 ) ) ;
#24293=CARTESIAN_POINT ( 'NONE',  ( 34.05464809739185483, -5.407089921784861808, 163.3968466864631068 ) ) ;
#24300=CARTESIAN_POINT ( 'NONE',  ( 24.94881294716939379, 3.604726614523236616, 166.7720662417328299 ) ) ;
#24316=FACE_OUTER_BOUND ( 'NONE', #8980, .T. ) ;
#24319=EDGE_CURVE ( 'NONE', #16861, #5932, #6066, .T. ) ;
#24328=CARTESIAN_POINT ( 'NONE',  ( 26.75643035624999655, 3.323476615752271712, -3.590624999385491734 ) ) ;
#24332=CARTESIAN_POINT ( 'NONE',  ( 26.75643035624999655, -3.323476615752267271, -7.603124999385488358 ) ) ;
#24338=AXIS2_PLACEMENT_3D ( 'NONE', #12080, #26481, #23463 ) ;
#24339=CARTESIAN_POINT ( 'NONE',  ( 36.56647878446795374, 3.464101615137755275, 159.0833872022828359 ) ) ;
#24343=CARTESIAN_POINT ( 'NONE',  ( 23.87821517812499650, 4.985214923628404904, -5.803124999385484095 ) ) ;
#24351=( BOUNDED_CURVE ( )  B_SPLINE_CURVE ( 2, ( #32888, #36101, #7307, #30430, #16030, #6939, #8241 ),
 .UNSPECIFIED., .F., .F. ) 
 B_SPLINE_CURVE_WITH_KNOTS ( ( 3, 2, 2, 3 ),
 ( 0.1739130434782605039, 0.1811594202898547945, 0.1884057971014491129, 0.1956521739130434034 ),
 .UNSPECIFIED. ) 
 CURVE ( )  GEOMETRIC_REPRESENTATION_ITEM ( )  RATIONAL_B_SPLINE_CURVE ( ( 1.000000000000006661, 0.8660254037844320463, 1.000000000000000000, 0.8660254037844387076, 1.000000000000000000, 0.8660254037844402619, 0.9999999999999984457 ) ) 
 REPRESENTATION_ITEM ( '' )  );
#24367=CARTESIAN_POINT ( 'NONE',  ( 27.91164311941789933, -5.407089921784859143, 164.8189062138541772 ) ) ;
#24368=DIRECTION ( 'NONE',  ( 0.1742906073607703166, -0.9846942592428442609, 0.000000000000000000 ) ) ;
#24373=EDGE_LOOP ( 'NONE', ( #2080, #32140, #26628, #35021 ) ) ;
#24375=CARTESIAN_POINT ( 'NONE',  ( 15.24356964374999990, 3.323476615752268604, -0.6281249993854746139 ) ) ;
#24378=CARTESIAN_POINT ( 'NONE',  ( 26.75643035624999655, 3.323476615752271712, -7.978124999385458160 ) ) ;
#24385=CARTESIAN_POINT ( 'NONE',  ( 28.23805287048444512, 5.196152422706630247, 167.1524626168076111 ) ) ;
#24389=CARTESIAN_POINT ( 'NONE',  ( 20.99999999999999645, 6.646953231504538984, -0.3656249993854637226 ) ) ;
#24393=ORIENTED_EDGE ( 'NONE', *, *, #30257, .F. ) ;
#24397=CARTESIAN_POINT ( 'NONE',  ( 34.40762885551985306, -5.407089921784861808, 167.4314352137346873 ) ) ;
#24399=( BOUNDED_CURVE ( )  B_SPLINE_CURVE ( 2, ( #32214, #17830, #36361, #36174, #24626, #1309, #33158 ),
 .UNSPECIFIED., .F., .F. ) 
 B_SPLINE_CURVE_WITH_KNOTS ( ( 3, 2, 2, 3 ),
 ( 0.06521739130434869858, 0.07246376811594300305, 0.07971014492753727976, 0.08695652173913158423 ),
 .UNSPECIFIED. ) 
 CURVE ( )  GEOMETRIC_REPRESENTATION_ITEM ( )  RATIONAL_B_SPLINE_CURVE ( ( 0.9999999999999837907, 0.8660254037844549169, 1.000000000000000000, 0.8660254037844387076, 1.000000000000000000, 0.8660254037844173913, 1.000000000000021316 ) ) 
 REPRESENTATION_ITEM ( '' )  );
#24410=ORIENTED_EDGE ( 'NONE', *, *, #6809, .T. ) ;
#24412=VERTEX_POINT ( 'NONE', #3980 ) ;
#24413=CARTESIAN_POINT ( 'NONE',  ( 21.00000000000000000, 6.928203230275506996, -1.012500000000014388 ) ) ;
#24416=CARTESIAN_POINT ( 'NONE',  ( 24.59746635921792901, -3.604726614523244610, 162.7561563650505434 ) ) ;
#24417=CARTESIAN_POINT ( 'NONE',  ( 36.74950584413092258, 7.347880794884125653E-16, 161.1753960670511674 ) ) ;
#24423=EDGE_LOOP ( 'NONE', ( #14249, #4944, #15567, #10051 ) ) ;
#24428=CARTESIAN_POINT ( 'NONE',  ( 23.87821517812499650, 4.985214923628404904, -6.703124999385495997 ) ) ;
#24431=CARTESIAN_POINT ( 'NONE',  ( 27.00000000000015632, -3.464101615137659351, -6.506249998770940124 ) ) ;
#24440=VECTOR ( 'NONE', #28499, 1000.000000000000000 ) ;
#24442=CARTESIAN_POINT ( 'NONE',  ( 34.17721086063072988, -5.407089921784855591, 164.7977454806546120 ) ) ;
#24449=FACE_OUTER_BOUND ( 'NONE', #4293, .T. ) ;
#24452=CARTESIAN_POINT ( 'NONE',  ( 34.26872439051576436, 5.407089921784857367, 165.8437499136509814 ) ) ;
#24453=CARTESIAN_POINT ( 'NONE',  ( 15.24356964374999990, 0.000000000000000000, -3.740624999385461003 ) ) ;
#24458=CARTESIAN_POINT ( 'NONE',  ( 23.99999999999999645, 5.196152422706631135, -3.243749998770945275 ) ) ;
#24469=CARTESIAN_POINT ( 'NONE',  ( 23.87821517812499650, 4.985214923628404904, -1.640624999385470462 ) ) ;
#24472=CARTESIAN_POINT ( 'NONE',  ( 23.87821517812500005, -4.985214923628404016, -0.5531249993854792102 ) ) ;
#24475=EDGE_LOOP ( 'NONE', ( #25631, #16134, #12481, #29245 ) ) ;
#24478=CARTESIAN_POINT ( 'NONE',  ( 37.16782192588006239, -3.604726614523238837, 163.1621225127927062 ) ) ;
#24481=PRESENTATION_STYLE_ASSIGNMENT (( #27692 ) ) ;
#24482=CARTESIAN_POINT ( 'NONE',  ( 15.02283181144952628, 7.347880794884122694E-16, 50.52293445648592751 ) ) ;
#24485=CARTESIAN_POINT ( 'NONE',  ( 37.33287311370841621, 7.646167579472015790E-16, 165.0486662223039218 ) ) ;
#24499=LINE ( 'NONE', #7072, #623 ) ;
#24506=VERTEX_POINT ( 'NONE', #14803 ) ;
#24511=CARTESIAN_POINT ( 'NONE',  ( 21.00000000000000000, 6.646953231504538984, -3.965624999385493510 ) ) ;
#24514=CARTESIAN_POINT ( 'NONE',  ( 20.99999999999999645, -6.646953231504538984, -6.328124999385495109 ) ) ;
#24519=CARTESIAN_POINT ( 'NONE',  ( 24.58926402489574770, 0.000000000000000000, 159.8677550070055702 ) ) ;
#24524=EDGE_CURVE ( 'NONE', #7551, #31196, #24084, .T. ) ;
#24528=LINE ( 'NONE', #30777, #18374 ) ;
#24549=CARTESIAN_POINT ( 'NONE',  ( 37.25116460488249004, -3.604726614523235284, 164.1147336928429468 ) ) ;
#24551=CARTESIAN_POINT ( 'NONE',  ( 37.37702719191401002, 7.347880794884125653E-16, 168.3479978933117422 ) ) ;
#24555=ORIENTED_EDGE ( 'NONE', *, *, #36792, .T. ) ;
#24556=EDGE_LOOP ( 'NONE', ( #20542, #15266, #30008, #8784 ) ) ;
#24557=CARTESIAN_POINT ( 'NONE',  ( 15.00000000000000000, 0.000000000000000000, -4.893749998770957177 ) ) ;
#24560=CARTESIAN_POINT ( 'NONE',  ( 20.99999999999999645, 0.000000000000000000, -8.000000000000000000 ) ) ;
#24561=CARTESIAN_POINT ( 'NONE',  ( 26.75643035624999655, 3.323476615752271712, -8.878124999385482496 ) ) ;
#24566=CARTESIAN_POINT ( 'NONE',  ( 34.23483110115314787, -5.196152422706629359, 166.8536719673923017 ) ) ;
#24572=( BOUNDED_CURVE ( )  B_SPLINE_CURVE ( 2, ( #26006, #11421, #20146, #22988, #34538, #14083, #8577 ),
 .UNSPECIFIED., .F., .F. ) 
 B_SPLINE_CURVE_WITH_KNOTS ( ( 3, 2, 2, 3 ),
 ( 0.6739130434782618639, 0.6811594202898562100, 0.6884057971014503341, 0.6956521739130446802 ),
 .UNSPECIFIED. ) 
 CURVE ( )  GEOMETRIC_REPRESENTATION_ITEM ( )  RATIONAL_B_SPLINE_CURVE ( ( 0.9999999999999815703, 0.8660254037844571373, 1.000000000000000000, 0.8660254037844387076, 1.000000000000000000, 0.8660254037844161701, 1.000000000000022649 ) ) 
 REPRESENTATION_ITEM ( '' )  );
#24573=CARTESIAN_POINT ( 'NONE',  ( 36.74950584413092258, 7.347880794884125653E-16, 161.1753960670511674 ) ) ;
#24578=CARTESIAN_POINT ( 'NONE',  ( 24.74614436184151955, 0.000000000000000000, 161.6609054635707423 ) ) ;
#24580=LINE ( 'NONE', #9616, #26541 ) ;
#24581=CARTESIAN_POINT ( 'NONE',  ( 24.82625018393050809, 3.604726614523240613, 165.3711674475413531 ) ) ;
#24588=CARTESIAN_POINT ( 'NONE',  ( 36.70701741954223252, -3.464101615137295642, 160.6897511517313717 ) ) ;
#24596=CARTESIAN_POINT ( 'NONE',  ( 21.00000000000000000, 6.928203230275506996, -2.362500000000001155 ) ) ;
#24598=CARTESIAN_POINT ( 'NONE',  ( 30.96108431102187808, 7.209453229046482114, 163.8557146672041824 ) ) ;
#24599=CARTESIAN_POINT ( 'NONE',  ( 30.82136276087599214, 6.928203230275514990, 162.2586900412136686 ) ) ;
#24606=ORIENTED_EDGE ( 'NONE', *, *, #31239, .T. ) ;
#24610=CARTESIAN_POINT ( 'NONE',  ( 26.75643035624999655, 3.323476615752271712, -7.190624999385489602 ) ) ;
#24624=CARTESIAN_POINT ( 'NONE',  ( 24.52392870127459545, -3.604726614523240613, 161.9156170885356403 ) ) ;
#24626=CARTESIAN_POINT ( 'NONE',  ( 18.00000000000000355, -5.196152422706632912, -0.8249999999999924061 ) ) ;
#24628=CARTESIAN_POINT ( 'NONE',  ( 29.49486714975617474, 6.148716665048037378, 159.5363409456820136 ) ) ;
#24633=VERTEX_POINT ( 'NONE', #29572 ) ;
#24634=CARTESIAN_POINT ( 'NONE',  ( 27.95086320365434318, -5.407089921784859143, 165.2671938279954702 ) ) ;
#24635=CARTESIAN_POINT ( 'NONE',  ( 15.24356964374999990, 0.000000000000000000, -5.090624999385479299 ) ) ;
#24637=CARTESIAN_POINT ( 'NONE',  ( 25.44230085693126497, 0.000000000000000000, 169.6180106133541869 ) ) ;
#24647=CARTESIAN_POINT ( 'NONE',  ( 15.24356964374999990, 3.323476615752268604, -3.778124999385444660 ) ) ;
#24649=CARTESIAN_POINT ( 'NONE',  ( 18.00000000000000355, -5.196152422706632912, -8.868749998770963927 ) ) ;
#24656=CARTESIAN_POINT ( 'NONE',  ( 24.55824627498148160, -3.604726614523244610, 162.3078687509092788 ) ) ;
#24670=FACE_OUTER_BOUND ( 'NONE', #7223, .T. ) ;
#24684=ORIENTED_EDGE ( 'NONE', *, *, #14588, .F. ) ;
#24690=CARTESIAN_POINT ( 'NONE',  ( 15.24356964374999990, 3.323476615752268604, -7.490624999385497418 ) ) ;
#24694=CARTESIAN_POINT ( 'NONE',  ( 18.12178482187500350, -4.985214923628407568, -6.815624999385455851 ) ) ;
#24697=CARTESIAN_POINT ( 'NONE',  ( 34.45992230116843302, 5.407089921784862696, 168.0291520325897636 ) ) ;
#24700=CARTESIAN_POINT ( 'NONE',  ( 24.62848410913218800, 0.000000000000000000, 160.3160426211468348 ) ) ;
#24721=CARTESIAN_POINT ( 'NONE',  ( 25.10239346032281560, -3.464101615137910262, 165.7328512920207402 ) ) ;
#24731=CARTESIAN_POINT ( 'NONE',  ( 30.90715669519676467, -7.209453229046475009, 163.2393191977598974 ) ) ;
#24736=ORIENTED_EDGE ( 'NONE', *, *, #10404, .F. ) ;
#24739=CARTESIAN_POINT ( 'NONE',  ( 15.00000000000000000, 0.000000000000000000, -4.443749998770951670 ) ) ;
#24740=CARTESIAN_POINT ( 'NONE',  ( 26.75643035624999655, -3.323476615752267271, -1.303124999385484095 ) ) ;
#24743=CARTESIAN_POINT ( 'NONE',  ( 23.87821517812500005, -4.985214923628404016, -9.890624999385478233 ) ) ;
#24750=CARTESIAN_POINT ( 'NONE',  ( 25.17429694808935992, 3.464101615137752166, 166.5547119179464346 ) ) ;
#24754=CARTESIAN_POINT ( 'NONE',  ( 26.75643035624999655, 3.323476615752271268, -0.8906249993854854496 ) ) ;
#24763=CARTESIAN_POINT ( 'NONE',  ( 31.05913452161298949, -7.209453229046482114, 164.9764337025573866 ) ) ;
#24767=( BOUNDED_CURVE ( )  B_SPLINE_CURVE ( 2, ( #9290, #9848, #32216, #7019, #1311, #26907, #20864 ),
 .UNSPECIFIED., .F., .F. ) 
 B_SPLINE_CURVE_WITH_KNOTS ( ( 3, 2, 2, 3 ),
 ( 0.5000000000000013323, 0.5072463768115947902, 0.5144927536231880261, 0.5217391304347814840 ),
 .UNSPECIFIED. ) 
 CURVE ( )  GEOMETRIC_REPRESENTATION_ITEM ( )  RATIONAL_B_SPLINE_CURVE ( ( 0.9999999999999753530, 0.8660254037844633546, 1.000000000000000000, 0.8660254037844387076, 1.000000000000000000, 0.8660254037844592467, 0.9999999999999794609 ) ) 
 REPRESENTATION_ITEM ( '' )  );
#24772=DIRECTION ( 'NONE',  ( 0.9961946980917462113, 0.000000000000000000, -0.08715574274765118534 ) ) ;
#24774=DIRECTION ( 'NONE',  ( 0.000000000000000000, 0.000000000000000000, 1.000000000000000000 ) ) ;
#24780=CARTESIAN_POINT ( 'NONE',  ( 26.99999999999999645, 7.347880794884117764E-16, -1.574999999999993072 ) ) ;
#24781=CARTESIAN_POINT ( 'NONE',  ( 37.12860184164362209, -3.604726614523238837, 162.7138348986514131 ) ) ;
#24782=CARTESIAN_POINT ( 'NONE',  ( 24.73307100032225136, 3.464101615137757051, 161.5114762576325802 ) ) ;
#24784=CARTESIAN_POINT ( 'NONE',  ( 29.49992229830193935, 6.068759932216713615, 159.4323797615155058 ) ) ;
#24785=ADVANCED_FACE ( 'NONE', ( #7771 ), #33973, .F. ) ;
#24789=ORIENTED_EDGE ( 'NONE', *, *, #21788, .T. ) ;
#24791=CARTESIAN_POINT ( 'NONE',  ( 18.00000000000000355, -5.196152422706632912, -3.975000000000006306 ) ) ;
#24793=CARTESIAN_POINT ( 'NONE',  ( 26.75643035624999655, 3.323476615752271712, -7.640624999385485339 ) ) ;
#24795=( BOUNDED_CURVE ( )  B_SPLINE_CURVE ( 2, ( #11270, #28324, #28690, #22841, #34388, #19999, #31543 ),
 .UNSPECIFIED., .F., .F. ) 
 B_SPLINE_CURVE_WITH_KNOTS ( ( 3, 2, 2, 3 ),
 ( 0.9130434782608709554, 0.9202898550724650795, 0.9275362318840590925, 0.9347826086956532166 ),
 .UNSPECIFIED. ) 
 CURVE ( )  GEOMETRIC_REPRESENTATION_ITEM ( )  RATIONAL_B_SPLINE_CURVE ( ( 0.9999999999999733546, 0.8660254037844653530, 1.000000000000000000, 0.8660254037844387076, 1.000000000000000000, 0.8660254037844202779, 1.000000000000018430 ) ) 
 REPRESENTATION_ITEM ( '' )  );
#24797=CARTESIAN_POINT ( 'NONE',  ( 31.36063891923419789, -6.928203230275506996, 168.4226447368806987 ) ) ;
#24806=CARTESIAN_POINT ( 'NONE',  ( 27.70246933682352974, 5.407089921784856479, 162.4280389384339855 ) ) ;
#24807=CARTESIAN_POINT ( 'NONE',  ( 15.00000000000000000, 0.000000000000000000, -0.8437499987709595750 ) ) ;
#24818=CARTESIAN_POINT ( 'NONE',  ( 27.99008328789078703, -5.407089921784859143, 165.7154814421367348 ) ) ;
#24819=CARTESIAN_POINT ( 'NONE',  ( 15.24356964374999990, 3.323476615752268604, -4.678124999385468108 ) ) ;
#24821=CARTESIAN_POINT ( 'NONE',  ( 28.46356835473687852, 5.196152422706636465, 169.7301163968956530 ) ) ;
#24829=( BOUNDED_CURVE ( )  B_SPLINE_CURVE ( 2, ( #27005, #21524, #27377, #18869, #1407, #9575, #18686 ),
 .UNSPECIFIED., .F., .F. ) 
 B_SPLINE_CURVE_WITH_KNOTS ( ( 3, 2, 2, 3 ),
 ( 0.1304347826086954820, 0.1376811594202895228, 0.1449275362318835914, 0.1521739130434776321 ),
 .UNSPECIFIED. ) 
 CURVE ( )  GEOMETRIC_REPRESENTATION_ITEM ( )  RATIONAL_B_SPLINE_CURVE ( ( 1.000000000000002887, 0.8660254037844354880, 1.000000000000000000, 0.8660254037844387076, 1.000000000000000000, 0.8660254037844504760, 0.9999999999999882316 ) ) 
 REPRESENTATION_ITEM ( '' )  );
#24832=CARTESIAN_POINT ( 'NONE',  ( 21.00000000000000000, -6.646953231504538984, -4.528124999385448213 ) ) ;
#24835=CARTESIAN_POINT ( 'NONE',  ( 18.00000000000000355, -5.196152422706632912, -9.318749998770941900 ) ) ;
#24843=CARTESIAN_POINT ( 'NONE',  ( 27.61912665782109499, 5.407089921784862696, 161.4754277583837734 ) ) ;
#24867=CARTESIAN_POINT ( 'NONE',  ( 14.99999999999989697, -3.464101615137695767, -2.212500000000015454 ) ) ;
#24872=CARTESIAN_POINT ( 'NONE',  ( 21.00000000000000000, -6.928203230275506996, -9.337499999999982592 ) ) ;
#24878=CARTESIAN_POINT ( 'NONE',  ( 21.00000000000000000, -6.646953231504538984, -6.440624999385486049 ) ) ;
#24883=CARTESIAN_POINT ( 'NONE',  ( 23.87821517812500005, -4.985214923628404016, -7.190624999385470062 ) ) ;
#24892=EDGE_CURVE ( 'NONE', #16979, #15602, #32842, .T. ) ;
#24906=CARTESIAN_POINT ( 'NONE',  ( 15.00000000000000000, 0.000000000000000000, -5.343749998770963572 ) ) ;
#24912=LINE ( 'NONE', #36464, #5079 ) ;
#24916=CARTESIAN_POINT ( 'NONE',  ( 37.17272443640959523, -3.604726614523235284, 163.2181584645603323 ) ) ;
#24917=CARTESIAN_POINT ( 'NONE',  ( 27.92756053683882911, -5.196152422706638241, 163.6035190036313622 ) ) ;
#24923=CARTESIAN_POINT ( 'NONE',  ( 15.00000000000000178, -3.464101615137757051, -3.956249998770955845 ) ) ;
#24924=CARTESIAN_POINT ( 'NONE',  ( 18.12178482187499640, 4.985214923628404904, -0.2156249993854608693 ) ) ;
#24926=CARTESIAN_POINT ( 'NONE',  ( 26.99999999999999645, 7.347880794884117764E-16, -4.725000000000006750 ) ) ;
#24927=CARTESIAN_POINT ( 'NONE',  ( 23.87821517812499650, 4.985214923628404904, -8.840624999385482852 ) ) ;
#24933=CARTESIAN_POINT ( 'NONE',  ( 37.07307153918868181, 7.347880794884117764E-16, 164.8737688849411143 ) ) ;
#24937=CARTESIAN_POINT ( 'NONE',  ( 18.12178482187499640, 4.985214923628404904, -1.678124999385494087 ) ) ;
#24944=CARTESIAN_POINT ( 'NONE',  ( 37.07633987954135080, 3.464101615137969770, 164.9111261861195885 ) ) ;
#24945=CARTESIAN_POINT ( 'NONE',  ( 27.85444716323975101, 5.407089921784862696, 164.1651534432314747 ) ) ;
#24952=CARTESIAN_POINT ( 'NONE',  ( 24.73633934067528983, 0.000000000000000000, 161.5488335588110544 ) ) ;
#24960=CARTESIAN_POINT ( 'NONE',  ( 15.00000000000000178, -3.464101615137757051, -2.212500000000014122 ) ) ;
#24961=CARTESIAN_POINT ( 'NONE',  ( 30.92186422678543423, 7.209453229046482114, 163.4074270530628894 ) ) ;
#24962=CARTESIAN_POINT ( 'NONE',  ( 36.79199426872038714, 3.464101615137759271, 161.6610409823708778 ) ) ;
#24967=ORIENTED_EDGE ( 'NONE', *, *, #17548, .F. ) ;
#24968=ORIENTED_EDGE ( 'NONE', *, *, #10058, .F. ) ;
#24972=CARTESIAN_POINT ( 'NONE',  ( 26.75643035624999655, -3.323476615752267715, -9.065624999385498484 ) ) ;
#24975=CARTESIAN_POINT ( 'NONE',  ( 25.37693404997770230, -3.464101615137787693, 168.8708645910097346 ) ) ;
#24978=VECTOR ( 'NONE', #14026, 1000.000000000000000 ) ;
#24988=CARTESIAN_POINT ( 'NONE',  ( 30.73066631613276556, 7.209453229046475009, 161.2220249341241072 ) ) ;
#24989=CARTESIAN_POINT ( 'NONE',  ( 26.99999999999999645, 7.347880794884117764E-16, -1.068749998770962550 ) ) ;
#24998=CARTESIAN_POINT ( 'NONE',  ( 15.24356964374999990, 0.000000000000000000, -0.1406249993854691294 ) ) ;
#25000=ORIENTED_EDGE ( 'NONE', *, *, #14263, .T. ) ;
#25001=CARTESIAN_POINT ( 'NONE',  ( 37.25116460488249004, -3.604726614523235284, 164.1147336928428899 ) ) ;
#25002=CARTESIAN_POINT ( 'NONE',  ( 26.75643035624999655, 7.049594010296217766E-16, -5.765624999385460470 ) ) ;
#25004=CARTESIAN_POINT ( 'NONE',  ( 19.32307722456181409, 5.539345343143609490, -8.000000000000000000 ) ) ;
#25005=CARTESIAN_POINT ( 'NONE',  ( 25.40634911304786314, -3.464101615137761048, 169.2070803003913397 ) ) ;
#25017=CARTESIAN_POINT ( 'NONE',  ( 26.75643035624999655, 7.049594010296217766E-16, -3.515624999385458249 ) ) ;
#25020=CARTESIAN_POINT ( 'NONE',  ( 18.00000000000000000, 5.196152422706630247, -8.568749998770941900 ) ) ;
#25042=VERTEX_POINT ( 'NONE', #21858 ) ;
#25050=CARTESIAN_POINT ( 'NONE',  ( 20.99999999999999645, -6.928203230275506996, -5.737500000000017586 ) ) ;
#25052=CARTESIAN_POINT ( 'NONE',  ( 28.00600070531170971, -5.196152422706638241, 164.5000942319139483 ) ) ;
#25056=CARTESIAN_POINT ( 'NONE',  ( 23.99999999999999645, 5.196152422706631135, -8.699999999999985079 ) ) ;
#25062=CARTESIAN_POINT ( 'NONE',  ( 23.87821517812500005, -4.985214923628404016, -6.853124999385479477 ) ) ;
#25086=EDGE_LOOP ( 'NONE', ( #4849, #7241, #29672, #17281 ) ) ;
#25093=CARTESIAN_POINT ( 'NONE',  ( 31.08609832957909092, -6.928203230275506996, 165.2846314378917043 ) ) ;
#25102=CARTESIAN_POINT ( 'NONE',  ( 37.06160086440634416, 3.604726614523238837, 161.9480102244933732 ) ) ;
#25103=CARTESIAN_POINT ( 'NONE',  ( 23.87821517812500005, -4.985214923628404016, -0.5531249993854792102 ) ) ;
#25106=ORIENTED_EDGE ( 'NONE', *, *, #29738, .F. ) ;
#25110=CARTESIAN_POINT ( 'NONE',  ( 18.00000000000000355, -5.196152422706632912, -4.368749998770960374 ) ) ;
#25111=CARTESIAN_POINT ( 'NONE',  ( 26.75643035624999655, -3.323476615752267271, -3.553124999385494753 ) ) ;
#25118=ADVANCED_FACE ( 'NONE', ( #14718 ), #14904, .T. ) ;
#25120=( BOUNDED_CURVE ( )  B_SPLINE_CURVE ( 2, ( #2114, #10276, #36791, #28081, #13310, #30751, #13494 ),
 .UNSPECIFIED., .F., .F. ) 
 B_SPLINE_CURVE_WITH_KNOTS ( ( 3, 2, 2, 3 ),
 ( 0.1086956521739118053, 0.1159420289855061098, 0.1231884057971004143, 0.1304347826086947049 ),
 .UNSPECIFIED. ) 
 CURVE ( )  GEOMETRIC_REPRESENTATION_ITEM ( )  RATIONAL_B_SPLINE_CURVE ( ( 1.000000000000022871, 0.8660254037844159480, 1.000000000000000000, 0.8660254037844387076, 1.000000000000000000, 0.8660254037844561381, 0.9999999999999825695 ) ) 
 REPRESENTATION_ITEM ( '' )  );
#25122=CARTESIAN_POINT ( 'NONE',  ( 28.04195244930222586, 5.196152422706630247, 164.9110245461011743 ) ) ;
#25127=CARTESIAN_POINT ( 'NONE',  ( 15.24356964375000167, -3.323476615752272600, -2.915624999385482141 ) ) ;
#25132=ORIENTED_EDGE ( 'NONE', *, *, #12154, .F. ) ;
#25133=CARTESIAN_POINT ( 'NONE',  ( 36.82794601260381029, 7.347880794884125653E-16, 162.0719712953337250 ) ) ;
#25136=AXIS2_PLACEMENT_3D ( 'NONE', #35999, #10036, #10595 ) ;
#25138=CARTESIAN_POINT ( 'NONE',  ( 24.71185827157421855, 0.000000000000000000, 164.0636619062959483 ) ) ;
#25148=FACE_OUTER_BOUND ( 'NONE', #35812, .T. ) ;
#25151=CARTESIAN_POINT ( 'NONE',  ( 15.00000000000000000, 0.000000000000000000, -6.243749998770947940 ) ) ;
#25153=CARTESIAN_POINT ( 'NONE',  ( 23.99999999999999645, 5.196152422706631135, -2.400000000000013234 ) ) ;
#25154=CARTESIAN_POINT ( 'NONE',  ( 22.62369653919286350, -5.721836169135973371, -7.999999999999998224 ) ) ;
#25155=CARTESIAN_POINT ( 'NONE',  ( 24.35887751344623098, 0.000000000000000000, 160.0290733790243962 ) ) ;
#25157=CARTESIAN_POINT ( 'NONE',  ( 36.63511393177462594, 3.464101615137759271, 159.8678905258057341 ) ) ;
#25168=CARTESIAN_POINT ( 'NONE',  ( 23.87821517812500005, -4.985214923628404016, -10.00312499938549315 ) ) ;
#25170=EDGE_CURVE ( 'NONE', #4445, #12908, #12160, .T. ) ;
#25173=CARTESIAN_POINT ( 'NONE',  ( 25.37366570962461054, 0.000000000000000000, 168.8335072898312887 ) ) ;
#25176=CARTESIAN_POINT ( 'NONE',  ( 34.08121910445329661, 5.196152422706637353, 165.0978788107812818 ) ) ;
#25182=CARTESIAN_POINT ( 'NONE',  ( 25.08932009880328096, 0.000000000000000000, 165.5834220860826349 ) ) ;
#25183=CARTESIAN_POINT ( 'NONE',  ( 24.59910052939444824, 0.000000000000000000, 162.7748350156397521 ) ) ;
#25186=CARTESIAN_POINT ( 'NONE',  ( 33.59750473220383071, -5.196152422706635576, 159.5689982363720674 ) ) ;
#25187=CARTESIAN_POINT ( 'NONE',  ( 30.71350752933288675, 6.928203230275506996, 161.0258991035495058 ) ) ;
#25189=CARTESIAN_POINT ( 'NONE',  ( 25.20698035151260896, 0.000000000000000000, 166.9282849285064856 ) ) ;
#25195=CARTESIAN_POINT ( 'NONE',  ( 27.91164311941789933, -5.407089921784859143, 164.8189062138541772 ) ) ;
#25196=CARTESIAN_POINT ( 'NONE',  ( 15.24356964374999990, 3.323476615752268604, -5.578124999385491556 ) ) ;
#25198=CARTESIAN_POINT ( 'NONE',  ( 15.26092559546365734, -1.672032278976862685, -8.000000000000001776 ) ) ;
#25199=CARTESIAN_POINT ( 'NONE',  ( 34.39497977834484743, 5.196152422706637353, 168.6841797239115976 ) ) ;
#25208=AXIS2_PLACEMENT_3D ( 'NONE', #36073, #10300, #4236 ) ;
#25211=CARTESIAN_POINT ( 'NONE',  ( 26.75643035624999655, -3.323476615752267715, -4.003124999385458516 ) ) ;
#25214=CARTESIAN_POINT ( 'NONE',  ( 26.75643035624999655, 7.049594010296217766E-16, -1.378124999385471616 ) ) ;
#25227=CARTESIAN_POINT ( 'NONE',  ( 15.00000000000053468, -3.464101615138063472, -5.362499999999978506 ) ) ;
#25231=CARTESIAN_POINT ( 'NONE',  ( 25.36386068845838082, 0.000000000000000000, 168.7214353850716293 ) ) ;
#25238=CARTESIAN_POINT ( 'NONE',  ( 26.99999999999999645, 7.347880794884117764E-16, -2.925000000000010925 ) ) ;
#25240=ADVANCED_FACE ( 'NONE', ( #32142 ), #29296, .F. ) ;
#25241=CARTESIAN_POINT ( 'NONE',  ( 26.60793733450167053, 1.299049382686714882, -8.000000000000000000 ) ) ;
#25242=CARTESIAN_POINT ( 'NONE',  ( 24.66770419336863185, 0.000000000000000000, 160.7643302352881278 ) ) ;
#25244=CARTESIAN_POINT ( 'NONE',  ( 15.00000000000000000, 3.464101615137752166, -9.487500000000004263 ) ) ;
#25245=ORIENTED_EDGE ( 'NONE', *, *, #534, .T. ) ;
#25246=AXIS2_PLACEMENT_3D ( 'NONE', #19420, #16197, #33063 ) ;
#25251=CARTESIAN_POINT ( 'NONE',  ( 15.24356964374999990, 3.323476615752268604, -6.590624999385473970 ) ) ;
#25253=EDGE_CURVE ( 'NONE', #23933, #26829, #23796, .T. ) ;
#25254=EDGE_LOOP ( 'NONE', ( #29031, #22600, #23481, #6547 ) ) ;
#25255=UNCERTAINTY_MEASURE_WITH_UNIT (LENGTH_MEASURE( 1.000000000000000082E-05 ), #1171, 'distance_accuracy_value', 'NONE');
#25257=AXIS2_PLACEMENT_3D ( 'NONE', #30063, #4098, #15669 ) ;
#25259=CARTESIAN_POINT ( 'NONE',  ( 37.64173127707041289, 7.646167579472024665E-16, 168.5789311836665831 ) ) ;
#25265=CARTESIAN_POINT ( 'NONE',  ( 15.00000000000000000, 0.000000000000000000, -3.543749998770939769 ) ) ;
#25277=CARTESIAN_POINT ( 'NONE',  ( 15.00000000000000355, 7.347880794884112834E-16, -8.000000000000000000 ) ) ;
#25291=CARTESIAN_POINT ( 'NONE',  ( 30.73066631613276556, 7.209453229046475009, 161.2220249341241072 ) ) ;
#25295=VERTEX_POINT ( 'NONE', #12623 ) ;
#25297=CARTESIAN_POINT ( 'NONE',  ( 15.00000000000000000, 3.464101615137752166, -4.481249998770945098 ) ) ;
#25298=CARTESIAN_POINT ( 'NONE',  ( 20.99999999999999645, 6.646953231504538984, -2.503124999385450966 ) ) ;
#25300=CARTESIAN_POINT ( 'NONE',  ( 26.97716818855048260, 0.000000000000000000, 49.47706554351410801 ) ) ;
#25307=CARTESIAN_POINT ( 'NONE',  ( 28.12039261777511356, 5.196152422706630247, 165.8075997743837604 ) ) ;
#25311=CARTESIAN_POINT ( 'NONE',  ( 18.12178482187500350, -4.985214923628407568, -1.078124999385476901 ) ) ;
#25318=CARTESIAN_POINT ( 'NONE',  ( 20.99999999999999645, -6.928203230275506996, -6.637499999999977085 ) ) ;
#25323=CARTESIAN_POINT ( 'NONE',  ( 31.01991443737654564, -7.209453229046482114, 164.5281460884161220 ) ) ;
#25328=CARTESIAN_POINT ( 'NONE',  ( 36.68087069682425039, 7.347880794884117764E-16, 160.3908927435282692 ) ) ;
#25333=AXIS2_PLACEMENT_3D ( 'NONE', #20495, #5881, #32034 ) ;
#25339=CARTESIAN_POINT ( 'NONE',  ( 24.00000000000000000, -5.196152422706629359, -3.450000000000008615 ) ) ;
#25340=CARTESIAN_POINT ( 'NONE',  ( 26.77152063323770292, 0.3446893914122488023, -7.999999999999996447 ) ) ;
#25341=CARTESIAN_POINT ( 'NONE',  ( 24.51248951003896437, 3.604726614523240613, 161.7848665344110657 ) ) ;
#25343=CARTESIAN_POINT ( 'NONE',  ( 24.65789917220240213, 0.000000000000000000, 160.6522583305284968 ) ) ;
#25349=VERTEX_POINT ( 'NONE', #24187 ) ;
#25353=CARTESIAN_POINT ( 'NONE',  ( 26.75643035624999655, -3.323476615752267715, -9.965624999385457983 ) ) ;
#25354=EDGE_CURVE ( 'NONE', #29149, #31332, #15830, .T. ) ;
#25366=CARTESIAN_POINT ( 'NONE',  ( 24.51739202056851852, 3.604726614523236616, 161.8409024861786918 ) ) ;
#25370=CARTESIAN_POINT ( 'NONE',  ( 33.69882328325508070, 5.196152422706631135, 160.7270745741280962 ) ) ;
#25377=CARTESIAN_POINT ( 'NONE',  ( 27.75476278247212747, -5.407089921784859143, 163.0257557572890335 ) ) ;
#25378=CARTESIAN_POINT ( 'NONE',  ( 26.75643035624999655, 7.049594010296217766E-16, -4.865624999385476102 ) ) ;
#25381=CARTESIAN_POINT ( 'NONE',  ( 28.08976766865841057, 5.407089921784862696, 166.8548791280792045 ) ) ;
#25382=CARTESIAN_POINT ( 'NONE',  ( 37.22014685496823461, 7.347880794884125653E-16, 166.5548474367465985 ) ) ;
#25388=ORIENTED_EDGE ( 'NONE', *, *, #20852, .T. ) ;
#25393=CARTESIAN_POINT ( 'NONE',  ( 26.75643035624999655, 3.323476615752271712, -4.828124999385488003 ) ) ;
#25396=CARTESIAN_POINT ( 'NONE',  ( 26.75643035624999655, 3.323476615752271712, -0.8906249993854854496 ) ) ;
#25414=DIRECTION ( 'NONE',  ( 0.08715574274765150453, 0.000000000000000000, 0.9961946980917461003 ) ) ;
#25419=ORIENTED_EDGE ( 'NONE', *, *, #2636, .T. ) ;
#25429=CARTESIAN_POINT ( 'NONE',  ( 26.99999999999999645, -3.464101615137751278, -8.362499999999997158 ) ) ;
#25430=ORIENTED_EDGE ( 'NONE', *, *, #10791, .F. ) ;
#25435=CARTESIAN_POINT ( 'NONE',  ( 23.87821517812499650, 4.985214923628404904, -6.253124999385489602 ) ) ;
#25439=CARTESIAN_POINT ( 'NONE',  ( 37.52733936471412335, 3.604726614523243278, 167.2714256424211499 ) ) ;
#25442=CARTESIAN_POINT ( 'NONE',  ( 36.64165061258780298, 7.347880794884117764E-16, 159.9426051293869477 ) ) ;
#25447=ORIENTED_EDGE ( 'NONE', *, *, #22948, .T. ) ;
#25449=CARTESIAN_POINT ( 'NONE',  ( 26.99999999999999645, 7.347880794884117764E-16, -0.6187499987709565996 ) ) ;
#25464=CARTESIAN_POINT ( 'NONE',  ( 24.92917142150405496, 3.464101615137512358, 163.7529143283390454 ) ) ;
#25471=VERTEX_POINT ( 'NONE', #30627 ) ;
#25476=CARTESIAN_POINT ( 'NONE',  ( 24.63832061363088854, 0.000000000000000000, 163.2231226297810451 ) ) ;
#25482=CARTESIAN_POINT ( 'NONE',  ( 21.00000000000000000, 6.928203230275506996, -5.906249998770959131 ) ) ;
#25483=CARTESIAN_POINT ( 'NONE',  ( 15.24356964375000167, -3.323476615752272600, -3.253124999385454519 ) ) ;
#25493=CARTESIAN_POINT ( 'NONE',  ( 31.06648828746087077, 6.928203230275506996, 165.0604876308210862 ) ) ;
#25497=CARTESIAN_POINT ( 'NONE',  ( 15.24356964374999990, 0.000000000000000000, -3.853124999385476812 ) ) ;
#25503=CARTESIAN_POINT ( 'NONE',  ( 26.99999999999999645, 7.347880794884117764E-16, -6.525000000000003020 ) ) ;
#25506=CARTESIAN_POINT ( 'NONE',  ( 31.10570837169731107, 6.928203230275506996, 165.5087752449623224 ) ) ;
#25507=CARTESIAN_POINT ( 'NONE',  ( 24.67590652769081316, -3.604726614523244610, 163.6527315933331295 ) ) ;
#25511=DIRECTION ( 'NONE',  ( 0.000000000000000000, 0.000000000000000000, 1.000000000000000000 ) ) ;
#25521=CARTESIAN_POINT ( 'NONE',  ( 18.00000000000000355, -5.196152422706632912, -4.874999999999990230 ) ) ;
#25522=CARTESIAN_POINT ( 'NONE',  ( 28.03214742813599969, 5.196152422706636465, 164.7989526413415149 ) ) ;
#25524=CARTESIAN_POINT ( 'NONE',  ( 30.74537384772143866, -7.209453229046482114, 161.3901327894271276 ) ) ;
#25526=CARTESIAN_POINT ( 'NONE',  ( 31.39740774815230751, 7.209453229046475009, 168.8429143745260035 ) ) ;
#25534=CYLINDRICAL_SURFACE ( 'NONE', #5341, 6.000000000000001776 ) ;
#25536=CARTESIAN_POINT ( 'NONE',  ( 18.12178482187499640, 4.985214923628404904, -8.428124999385472549 ) ) ;
#25540=CARTESIAN_POINT ( 'NONE',  ( 33.89776776044609363, -5.407089921784861808, 161.6036962298979915 ) ) ;
#25543=( BOUNDED_CURVE ( )  B_SPLINE_CURVE ( 2, ( #7571, #2059, #33529, #19146, #4713, #33347, #16107 ),
 .UNSPECIFIED., .F., .F. ) 
 B_SPLINE_CURVE_WITH_KNOTS ( ( 3, 2, 2, 3 ),
 ( 0.6304347826086944551, 0.6376811594202886901, 0.6449275362318830362, 0.6521739130434773823 ),
 .UNSPECIFIED. ) 
 CURVE ( )  GEOMETRIC_REPRESENTATION_ITEM ( )  RATIONAL_B_SPLINE_CURVE ( ( 1.000000000000022649, 0.8660254037844161701, 1.000000000000000000, 0.8660254037844387076, 1.000000000000000000, 0.8660254037844551389, 0.9999999999999835687 ) ) 
 REPRESENTATION_ITEM ( '' )  );
#25551=CARTESIAN_POINT ( 'NONE',  ( 25.21845102629493951, 3.604726614523240613, 169.8540435889542550 ) ) ;
#25562=CARTESIAN_POINT ( 'NONE',  ( 24.68080903822037442, -3.604726614523240613, 163.7087675451007556 ) ) ;
#25563=CARTESIAN_POINT ( 'NONE',  ( 23.87821517812499650, 4.985214923628404904, -6.590624999385480187 ) ) ;
#25565=CARTESIAN_POINT ( 'NONE',  ( 34.30304196422265761, 5.407089921784862696, 166.2360015760246199 ) ) ;
#25566=CARTESIAN_POINT ( 'NONE',  ( 25.24620043574905282, 0.000000000000000000, 167.3765725426477502 ) ) ;
#25572=ORIENTED_EDGE ( 'NONE', *, *, #33252, .T. ) ;
#25577=VECTOR ( 'NONE', #1234, 1000.000000000000000 ) ;
#25580=CARTESIAN_POINT ( 'NONE',  ( 21.00000000000000000, -6.646953231504538984, -1.490624999385501193 ) ) ;
#25592=DIRECTION ( 'NONE',  ( 0.000000000000000000, 0.000000000000000000, 1.000000000000000000 ) ) ;
#25593=CARTESIAN_POINT ( 'NONE',  ( 26.99999999999999645, 7.347880794884117764E-16, -5.568749998770966769 ) ) ;
#25601=CARTESIAN_POINT ( 'NONE',  ( 24.89975635843378399, 3.464101615137476831, 163.4166986189574970 ) ) ;
#25607=CARTESIAN_POINT ( 'NONE',  ( 21.00000000000000355, 0.000000000000000000, 50.00000000000001421 ) ) ;
#25617=CARTESIAN_POINT ( 'NONE',  ( 26.75643035624999655, 3.323476615752271712, -9.440624999385470062 ) ) ;
#25623=CARTESIAN_POINT ( 'NONE',  ( 24.98639886122932197, 0.000000000000000000, 167.2016752052849426 ) ) ;
#25624=AXIS2_PLACEMENT_3D ( 'NONE', #22036, #12939, #30375 ) ;
#25631=ORIENTED_EDGE ( 'NONE', *, *, #594, .F. ) ;
#25641=DIRECTION ( 'NONE',  ( 1.000000000000000000, 0.000000000000000000, 0.000000000000000000 ) ) ;
#25646=CARTESIAN_POINT ( 'NONE',  ( 31.45868912971818432, 0.000000000000000000, 169.5433637710095809 ) ) ;
#25649=EDGE_CURVE ( 'NONE', #27232, #5916, #17268, .T. ) ;
#25657=EDGE_LOOP ( 'NONE', ( #19355, #34955, #13049, #4987, #14903 ) ) ;
#25660=CARTESIAN_POINT ( 'NONE',  ( 30.86793661096031727, -7.209453229046475009, 162.7910315836186328 ) ) ;
#25661=CARTESIAN_POINT ( 'NONE',  ( 21.00000000000000000, 6.646953231504538984, -0.3656249993854637226 ) ) ;
#25666=CARTESIAN_POINT ( 'NONE',  ( 15.00000000000000000, 3.464101615137752166, -7.631249998770947229 ) ) ;
#25667=CARTESIAN_POINT ( 'NONE',  ( 18.12178482187499640, 4.985214923628404904, -1.565624999385478722 ) ) ;
#25681=CARTESIAN_POINT ( 'NONE',  ( 31.04687824534265417, -6.928203230275506996, 164.8363438237504397 ) ) ;
#25686=CARTESIAN_POINT ( 'NONE',  ( 18.12178482187500350, -4.985214923628407568, -3.328124999385479121 ) ) ;
#25687=FACE_OUTER_BOUND ( 'NONE', #28829, .T. ) ;
#25691=CARTESIAN_POINT ( 'NONE',  ( 18.00000000000000355, -5.196152422706632912, -6.674999999999986500 ) ) ;
#25694=CARTESIAN_POINT ( 'NONE',  ( 27.65834674205753529, 5.407089921784862696, 161.9237153725250664 ) ) ;
#25707=CARTESIAN_POINT ( 'NONE',  ( 21.00000000000000000, -6.928203230275506996, -4.837499999999994138 ) ) ;
#25709=CARTESIAN_POINT ( 'NONE',  ( 36.89328133622495898, -3.604726614523238837, 160.0241092138036834 ) ) ;
#25711=CARTESIAN_POINT ( 'NONE',  ( 25.11222996482124259, -3.604726614523240613, 168.6399313006548653 ) ) ;
#25714=CARTESIAN_POINT ( 'NONE',  ( 20.99999999999999645, 0.000000000000000000, -8.000000000000000000 ) ) ;
#25717=ORIENTED_EDGE ( 'NONE', *, *, #34391, .T. ) ;
#25719=CARTESIAN_POINT ( 'NONE',  ( 20.99999999999999645, 6.928203230275506996, -5.006249998770934795 ) ) ;
#25721=EDGE_CURVE ( 'NONE', #36284, #1170, #26040, .T. ) ;
#25722=CARTESIAN_POINT ( 'NONE',  ( 23.87821517812499650, 4.985214923628404904, -8.503124999385491378 ) ) ;
#25726=CARTESIAN_POINT ( 'NONE',  ( 37.01094158893428698, -3.604726614523238837, 161.3689720562275340 ) ) ;
#25730=FILL_AREA_STYLE_COLOUR ( '', #18412 ) ;
#25738=CARTESIAN_POINT ( 'NONE',  ( 36.85896376251805151, -3.604726614523235284, 159.6318575514300449 ) ) ;
#25739=CARTESIAN_POINT ( 'NONE',  ( 15.00000000000000178, -3.464101615137757051, -2.156249998770940923 ) ) ;
#25741=CARTESIAN_POINT ( 'NONE',  ( 36.94560626531313829, 7.347880794884125653E-16, 163.4168341377576041 ) ) ;
#25747=CARTESIAN_POINT ( 'NONE',  ( 30.82871652672388052, -7.209453229046475009, 162.3427439694773398 ) ) ;
#25748=CARTESIAN_POINT ( 'NONE',  ( 18.12178482187499640, 4.985214923628404904, -7.865624999385478766 ) ) ;
#25750=CARTESIAN_POINT ( 'NONE',  ( 37.56002276824448671, -3.604726614523238837, 167.6449986542055797 ) ) ;
#25751=CARTESIAN_POINT ( 'NONE',  ( 28.16288104225748512, -5.196152422706638241, 166.2932446884790920 ) ) ;
#25758=ORIENTED_EDGE ( 'NONE', *, *, #15239, .F. ) ;
#25763=( BOUNDED_CURVE ( )  B_SPLINE_CURVE ( 2, ( #11499, #14530, #11681, #26086, #8657, #31771, #9216 ),
 .UNSPECIFIED., .F., .T. ) 
 B_SPLINE_CURVE_WITH_KNOTS ( ( 3, 2, 2, 3 ),
 ( 0.8913043478260880281, 0.8985507246376823742, 0.9057971014492767203, 0.9130434782608709554 ),
 .UNSPECIFIED. ) 
 CURVE ( )  GEOMETRIC_REPRESENTATION_ITEM ( )  RATIONAL_B_SPLINE_CURVE ( ( 0.9999999999999794609, 0.8660254037844592467, 1.000000000000000000, 0.8660254037844387076, 1.000000000000000000, 0.8660254037844120623, 1.000000000000026645 ) ) 
 REPRESENTATION_ITEM ( '' )  );
#25765=CARTESIAN_POINT ( 'NONE',  ( 15.24356964374999990, 3.323476615752268604, -2.090624999385484628 ) ) ;
#25770=CARTESIAN_POINT ( 'NONE',  ( 33.88185034302515675, -5.196152422706629359, 162.8190834401207496 ) ) ;
#25781=CARTESIAN_POINT ( 'NONE',  ( 26.99999999999985789, -3.464101615137830770, -0.2625000000000126121 ) ) ;
#25785=CARTESIAN_POINT ( 'NONE',  ( 24.65789917220240213, 0.000000000000000000, 160.6522583305284968 ) ) ;
#25787=CARTESIAN_POINT ( 'NONE',  ( 34.50404489593442747, 5.407089921784857367, 168.5334755984986828 ) ) ;
#25794=CARTESIAN_POINT ( 'NONE',  ( 37.41624727615045742, 7.347880794884125653E-16, 168.7962855074530069 ) ) ;
#25802=CARTESIAN_POINT ( 'NONE',  ( 15.24356964375000167, -3.323476615752272600, -9.665624999385482141 ) ) ;
#25804=EDGE_CURVE ( 'NONE', #28136, #4445, #24795, .T. ) ;
#25806=ORIENTED_EDGE ( 'NONE', *, *, #12248, .F. ) ;
#25809=CARTESIAN_POINT ( 'NONE',  ( 34.21152843433763024, -5.407089921784861808, 165.1899971430282505 ) ) ;
#25814=VECTOR ( 'NONE', #26650, 1000.000000000000000 ) ;
#25818=CARTESIAN_POINT ( 'NONE',  ( 25.15145004905768644, -3.604726614523240613, 169.0882189147961583 ) ) ;
#25832=DIRECTION ( 'NONE',  ( 0.08715574274765143514, 0.000000000000000000, 0.9961946980917462113 ) ) ;
#25847=CARTESIAN_POINT ( 'NONE',  ( 33.98111043944852128, -5.407089921784855591, 162.5563074099482037 ) ) ;
#25848=CARTESIAN_POINT ( 'NONE',  ( 23.87821517812499650, 4.985214923628404904, -2.653124999385497951 ) ) ;
#25852=VERTEX_POINT ( 'NONE', #23579 ) ;
#25854=CARTESIAN_POINT ( 'NONE',  ( 26.99999999999999645, 7.347880794884117764E-16, -6.918749998770956644 ) ) ;
#25855=CARTESIAN_POINT ( 'NONE',  ( 15.24356964375000167, -3.323476615752272600, -2.803124999385491201 ) ) ;
#25863=CARTESIAN_POINT ( 'NONE',  ( 33.85570362020085611, 5.196152422706631135, 162.5202250306932399 ) ) ;
#25867=EDGE_CURVE ( 'NONE', #26175, #4359, #17052, .T. ) ;
#25868=CARTESIAN_POINT ( 'NONE',  ( 15.24356964374999990, 0.000000000000000000, -4.753124999385488714 ) ) ;
#25878=CARTESIAN_POINT ( 'NONE',  ( 33.87162103762178589, 5.407089921784862696, 161.3048378204704534 ) ) ;
#25882=CARTESIAN_POINT ( 'NONE',  ( 23.99999999999999645, 5.196152422706631135, -4.200000000000009059 ) ) ;
#25884=DIRECTION ( 'NONE',  ( 1.000000000000000000, 0.000000000000000000, 0.000000000000000000 ) ) ;
#25887=CARTESIAN_POINT ( 'NONE',  ( 23.99999999999999645, 5.196152422706631135, -3.693749998770950782 ) ) ;
#25891=CARTESIAN_POINT ( 'NONE',  ( 15.00000000000000000, 0.000000000000000000, -4.500000000000003553 ) ) ;
#25894=CARTESIAN_POINT ( 'NONE',  ( 24.43404934156608022, 3.604726614523240613, 160.8882913061285080 ) ) ;
#25896=CARTESIAN_POINT ( 'NONE',  ( 27.61379986294728184, -5.196152422706638241, 160.0172180905011032 ) ) ;
#25900=ORIENTED_EDGE ( 'NONE', *, *, #6322, .T. ) ;
#25902=CARTESIAN_POINT ( 'NONE',  ( 23.34314575050770202, -3.999999999999897859, 49.79500130984166617 ) ) ;
#25908=CARTESIAN_POINT ( 'NONE',  ( 31.45868912971819142, 0.000000000000000000, 169.5433637710095809 ) ) ;
#25913=CARTESIAN_POINT ( 'NONE',  ( 36.93903810116746911, 3.604726614523243278, 160.5471114303018680 ) ) ;
#25920=ORIENTED_EDGE ( 'NONE', *, *, #1357, .F. ) ;
#25926=CARTESIAN_POINT ( 'NONE',  ( 25.22171936664797798, 0.000000000000000000, 169.8914008901326724 ) ) ;
#25927=CARTESIAN_POINT ( 'NONE',  ( 24.00000000000000000, -5.196152422706629359, -2.943749998770950338 ) ) ;
#25937=CARTESIAN_POINT ( 'NONE',  ( 33.98111043944852128, -5.407089921784855591, 162.5563074099482037 ) ) ;
#25938=CARTESIAN_POINT ( 'NONE',  ( 18.12178482187499640, 4.985214923628404904, -7.415624999385473259 ) ) ;
#25940=CARTESIAN_POINT ( 'NONE',  ( 37.60577953318700395, 3.604726614523243278, 168.1680008707037075 ) ) ;
#25941=CARTESIAN_POINT ( 'NONE',  ( 34.23809944139907202, 5.196152422706637353, 166.8910292673464539 ) ) ;
#25948=ORIENTED_EDGE ( 'NONE', *, *, #34391, .F. ) ;
#25951=CARTESIAN_POINT ( 'NONE',  ( 24.00000000000000000, -5.196152422706629359, -2.549999999999996714 ) ) ;
#25953=CARTESIAN_POINT ( 'NONE',  ( 18.12178482187499640, 4.985214923628404904, -2.578124999385478233 ) ) ;
#25971=EDGE_LOOP ( 'NONE', ( #4224, #10890, #7311, #25758 ) ) ;
#25972=CARTESIAN_POINT ( 'NONE',  ( 37.56819361912707222, 7.646167579472015790E-16, 167.7383919071516516 ) ) ;
#25984=ORIENTED_EDGE ( 'NONE', *, *, #24228, .F. ) ;
#25989=CARTESIAN_POINT ( 'NONE',  ( 18.12178482187500350, -4.985214923628407568, -8.728124999385494576 ) ) ;
#25995=CARTESIAN_POINT ( 'NONE',  ( 31.17679477432231394, -7.209453229046482114, 166.3212965449812657 ) ) ;
#26006=CARTESIAN_POINT ( 'NONE',  ( 26.99999999999999645, 7.347880794884117764E-16, -6.975000000000008527 ) ) ;
#26017=CARTESIAN_POINT ( 'NONE',  ( 28.29034631613303929, -5.196152422706632912, 167.7501794356626306 ) ) ;
#26019=DIRECTION ( 'NONE',  ( 0.08715574274765150453, 0.000000000000000000, 0.9961946980917461003 ) ) ;
#26022=CARTESIAN_POINT ( 'NONE',  ( 33.79360515338605353, -5.196152422706635576, 161.8104363070785041 ) ) ;
#26027=VERTEX_POINT ( 'NONE', #5322 ) ;
#26030=CARTESIAN_POINT ( 'NONE',  ( 27.51944227705346790, -5.407089921784859143, 160.3360300724413321 ) ) ;
#26031=CARTESIAN_POINT ( 'NONE',  ( 23.87821517812499650, 4.985214923628404904, -3.103124999385475924 ) ) ;
#26037=ORIENTED_EDGE ( 'NONE', *, *, #4718, .T. ) ;
#26038=CARTESIAN_POINT ( 'NONE',  ( 26.99999999999999645, 7.347880794884117764E-16, -7.368749998770962151 ) ) ;
#26039=CARTESIAN_POINT ( 'NONE',  ( 20.99999999999999645, 6.646953231504538984, -6.103124999385481253 ) ) ;
#26040=LINE ( 'NONE', #31730, #23347 ) ;
#26041=( BOUNDED_CURVE ( )  B_SPLINE_CURVE ( 3, ( #20481, #6051, #14227, #182 ),
 .UNSPECIFIED., .F., .F. ) 
 B_SPLINE_CURVE_WITH_KNOTS ( ( 4, 4 ),
 ( 3.141592653589793116, 4.712388980384648818 ),
 .UNSPECIFIED. ) 
 CURVE ( )  GEOMETRIC_REPRESENTATION_ITEM ( )  RATIONAL_B_SPLINE_CURVE ( ( 1.000000000000000000, 0.8047378541243747074, 0.8047378541243747074, 1.000000000000000000 ) ) 
 REPRESENTATION_ITEM ( '' )  );
#26048=CARTESIAN_POINT ( 'NONE',  ( 33.76419009031582874, -5.196152422706629359, 161.4742205976968989 ) ) ;
#26052=CARTESIAN_POINT ( 'NONE',  ( 20.99999999999999645, 6.646953231504538984, -5.315624999385481608 ) ) ;
#26057=CARTESIAN_POINT ( 'NONE',  ( 15.00000000000000000, 0.000000000000000000, -6.750000000000006217 ) ) ;
#26061=CARTESIAN_POINT ( 'NONE',  ( 33.83240095338533848, 5.407089921784862696, 160.8565502063291603 ) ) ;
#26076=CARTESIAN_POINT ( 'NONE',  ( 15.00000000000000000, 3.464101615137752166, -4.087499999999990585 ) ) ;
#26080=CARTESIAN_POINT ( 'NONE',  ( 37.45380170677077558, 3.604726614523238837, 166.4308863659062183 ) ) ;
#26082=CARTESIAN_POINT ( 'NONE',  ( 15.00000000000027711, 3.464101615137910706, -0.8812499987709506710 ) ) ;
#26086=CARTESIAN_POINT ( 'NONE',  ( 30.61545731874177534, -6.928203230275506996, 159.9051800681962732 ) ) ;
#26088=DIRECTION ( 'NONE',  ( 0.08715574274765150453, 0.000000000000000000, 0.9961946980917461003 ) ) ;
#26089=CARTESIAN_POINT ( 'NONE',  ( 26.75643035624999655, -3.323476615752267715, -6.703124999385464911 ) ) ;
#26091=CARTESIAN_POINT ( 'NONE',  ( 24.00000000000000000, -5.196152422706629359, -5.193749998770952558 ) ) ;
#26096=CARTESIAN_POINT ( 'NONE',  ( 25.37039736927157563, 3.464101615137752166, 168.7961499886528713 ) ) ;
#26100=CARTESIAN_POINT ( 'NONE',  ( 21.00000000000000355, 0.000000000000000000, 50.00000000000001421 ) ) ;
#26107=CARTESIAN_POINT ( 'NONE',  ( 38.17292378879935200, 7.686353184319896670, 158.6719570163914170 ) ) ;
#26108=CARTESIAN_POINT ( 'NONE',  ( 24.00000000000000000, -5.196152422706629359, -2.493749998770944387 ) ) ;
#26110=FACE_OUTER_BOUND ( 'NONE', #2901, .T. ) ;
#26118=CARTESIAN_POINT ( 'NONE',  ( 36.94067227134398479, 7.646167579472015790E-16, 160.5657900808910767 ) ) ;
#26119=CARTESIAN_POINT ( 'NONE',  ( 18.12178482187500350, -4.985214923628407568, -8.165624999385473259 ) ) ;
#26121=CARTESIAN_POINT ( 'NONE',  ( 24.98966720158235688, -3.604726614523244610, 167.2390325064633885 ) ) ;
#26122=CARTESIAN_POINT ( 'NONE',  ( 34.12043918868973691, 5.196152422706637353, 165.5461664249225748 ) ) ;
#26134=CARTESIAN_POINT ( 'NONE',  ( 15.24356964375000167, -3.323476615752272600, -4.715624999385497063 ) ) ;
#26143=CARTESIAN_POINT ( 'NONE',  ( 36.87370277765395343, -3.464101615137444412, 162.5949735130561749 ) ) ;
#26148=DIRECTION ( 'NONE',  ( 0.9961946980917462113, 0.000000000000000000, -0.08715574274765118534 ) ) ;
#26152=CARTESIAN_POINT ( 'NONE',  ( 36.90965452142909697, 3.464101615138126977, 163.0059038247948422 ) ) ;
#26157=VERTEX_POINT ( 'NONE', #5685 ) ;
#26160=CARTESIAN_POINT ( 'NONE',  ( 21.00000000000000000, -6.646953231504538984, -1.378124999385478056 ) ) ;
#26169=ORIENTED_EDGE ( 'NONE', *, *, #34842, .T. ) ;
#26173=CARTESIAN_POINT ( 'NONE',  ( 15.24356964374999990, 0.000000000000000000, -10.15312499938547575 ) ) ;
#26175=VERTEX_POINT ( 'NONE', #25785 ) ;
#26178=CARTESIAN_POINT ( 'NONE',  ( 37.48158259977161322, -3.604726614523238837, 166.7484234259230220 ) ) ;
#26184=CARTESIAN_POINT ( 'NONE',  ( 31.35818766391586365, 7.209453229046475009, 168.3946267603846820 ) ) ;
#26185=VERTEX_POINT ( 'NONE', #17454 ) ;
#26186=CARTESIAN_POINT ( 'NONE',  ( 26.97716818855048260, 0.000000000000000000, 49.47706554351410801 ) ) ;
#26187=FACE_OUTER_BOUND ( 'NONE', #10505, .T. ) ;
#26202=CARTESIAN_POINT ( 'NONE',  ( 21.00000000000000355, 0.000000000000000000, 50.00000000000001421 ) ) ;
#26205=CARTESIAN_POINT ( 'NONE',  ( 27.80990028412949755, -5.196152422706638241, 162.2586561612075116 ) ) ;
#26212=CARTESIAN_POINT ( 'NONE',  ( 21.00000000000000000, -6.646953231504538984, -1.040624999385473481 ) ) ;
#26218=ORIENTED_EDGE ( 'NONE', *, *, #34228, .T. ) ;
#26219=CARTESIAN_POINT ( 'NONE',  ( 15.24356964375000167, -3.323476615752272600, -4.603124999385474148 ) ) ;
#26226=CARTESIAN_POINT ( 'NONE',  ( 24.82131618996136879, 3.464101615137752166, 162.5201233906748541 ) ) ;
#26230=CARTESIAN_POINT ( 'NONE',  ( 15.24356964374999990, 3.323476615752268604, -4.340624999385463312 ) ) ;
#26238=DIRECTION ( 'NONE',  ( 1.000000000000000000, 0.000000000000000000, 0.000000000000000000 ) ) ;
#26239=AXIS2_PLACEMENT_3D ( 'NONE', #26576, #6307, #6686 ) ;
#26241=CARTESIAN_POINT ( 'NONE',  ( 33.93698784468253393, -5.407089921784861808, 162.0519838440392562 ) ) ;
#26250=CARTESIAN_POINT ( 'NONE',  ( 18.00000000000000000, 5.196152422706630247, -7.668749998770957532 ) ) ;
#26254=CARTESIAN_POINT ( 'NONE',  ( 26.99999999999999645, 3.464101615137755275, -4.237500000000010481 ) ) ;
#26258=CARTESIAN_POINT ( 'NONE',  ( 37.44726502606470575, -3.604726614523235284, 166.3561717635493835 ) ) ;
#26262=EDGE_CURVE ( 'NONE', #6369, #13208, #22587, .T. ) ;
#26264=ORIENTED_EDGE ( 'NONE', *, *, #1506, .F. ) ;
#26265=ORIENTED_EDGE ( 'NONE', *, *, #7799, .F. ) ;
#26268=CARTESIAN_POINT ( 'NONE',  ( 15.24356964374999990, 0.000000000000000000, -5.990624999385463667 ) ) ;
#26272=EDGE_CURVE ( 'NONE', #31540, #22269, #1539, .T. ) ;
#26275=EDGE_CURVE ( 'NONE', #24633, #16958, #36623, .T. ) ;
#26276=CARTESIAN_POINT ( 'NONE',  ( 26.99999999999999289, 0.000000000000000000, -8.000000000000000000 ) ) ;
#26277=CARTESIAN_POINT ( 'NONE',  ( 34.35249135386247588, -5.196152422706629359, 168.1985348098161808 ) ) ;
#26289=CARTESIAN_POINT ( 'NONE',  ( 34.45992230116843302, 5.407089921784862696, 168.0291520325897636 ) ) ;
#26290=CARTESIAN_POINT ( 'NONE',  ( 26.99999999999999645, 7.347880794884117764E-16, -1.518749998770940746 ) ) ;
#26295=CARTESIAN_POINT ( 'NONE',  ( 20.99999999999999645, 0.000000000000000000, -8.000000000000000000 ) ) ;
#26298=ORIENTED_EDGE ( 'NONE', *, *, #16382, .F. ) ;
#26299=CARTESIAN_POINT ( 'NONE',  ( 24.44548853280171130, -3.604726614523240613, 161.0190418602530258 ) ) ;
#26300=CARTESIAN_POINT ( 'NONE',  ( 15.24356964374999990, 3.323476615752268604, -7.828124999385470240 ) ) ;
#26303=CARTESIAN_POINT ( 'NONE',  ( 31.03952447949476579, 7.209453229046482114, 164.7522898954867685 ) ) ;
#26304=CARTESIAN_POINT ( 'NONE',  ( 28.00600070531170971, -5.196152422706638241, 164.5000942319139483 ) ) ;
#26312=ORIENTED_EDGE ( 'NONE', *, *, #12409, .T. ) ;
#26315=ADVANCED_FACE ( 'NONE', ( #23082 ), #17400, .T. ) ;
#26317=CARTESIAN_POINT ( 'NONE',  ( 15.24356964375000167, -3.323476615752272600, -3.815624999385473615 ) ) ;
#26323=( BOUNDED_CURVE ( )  B_SPLINE_CURVE ( 2, ( #12703, #23709, #29953, #35819, #9677, #29382, #12893 ),
 .UNSPECIFIED., .F., .F. ) 
 B_SPLINE_CURVE_WITH_KNOTS ( ( 3, 2, 2, 3 ),
 ( 0.3260869565217384136, 0.3333333333333327042, 0.3405797101449269948, 0.3478260869565212854 ),
 .UNSPECIFIED. ) 
 CURVE ( )  GEOMETRIC_REPRESENTATION_ITEM ( )  RATIONAL_B_SPLINE_CURVE ( ( 1.000000000000013545, 0.8660254037844254960, 1.000000000000000000, 0.8660254037844387076, 1.000000000000000000, 0.8660254037844469233, 0.9999999999999917843 ) ) 
 REPRESENTATION_ITEM ( '' )  );
#26331=CARTESIAN_POINT ( 'NONE',  ( 24.73307100032172201, 3.464101615137450185, 161.5114762576326370 ) ) ;
#26333=DIRECTION ( 'NONE',  ( 0.000000000000000000, -0.000000000000000000, -1.000000000000000000 ) ) ;
#26334=FACE_OUTER_BOUND ( 'NONE', #12642, .T. ) ;
#26335=CARTESIAN_POINT ( 'NONE',  ( 15.00000000000000000, 0.000000000000000000, -2.643749998770955401 ) ) ;
#26342=CARTESIAN_POINT ( 'NONE',  ( 34.54326498017087488, 5.407089921784857367, 168.9817632126399758 ) ) ;
#26344=CARTESIAN_POINT ( 'NONE',  ( 15.24356964374999990, 3.323476615752268604, -0.1781249993854788494 ) ) ;
#26349=CARTESIAN_POINT ( 'NONE',  ( 36.95214294612679851, -3.464101615137475942, 163.4915487413387893 ) ) ;
#26356=CARTESIAN_POINT ( 'NONE',  ( 23.87821517812500005, -4.985214923628404016, -10.00312499938549315 ) ) ;
#26364=CARTESIAN_POINT ( 'NONE',  ( 31.25523494279520165, -7.209453229046482114, 167.2178717732638233 ) ) ;
#26371=CARTESIAN_POINT ( 'NONE',  ( 25.05990503573306682, 0.000000000000000000, 165.2472063767010013 ) ) ;
#26372=CARTESIAN_POINT ( 'NONE',  ( 37.31166038496018444, 3.464101615137866297, 167.6008518709673183 ) ) ;
#26388=CARTESIAN_POINT ( 'NONE',  ( 15.00000000000000000, 0.000000000000000000, -3.993749998770945719 ) ) ;
#26392=STYLED_ITEM('',(#37528),#21232);
#26402=CARTESIAN_POINT ( 'NONE',  ( 27.46714883140487373, 5.407089921784856479, 159.7383132535862842 ) ) ;
#26403=CARTESIAN_POINT ( 'NONE',  ( 21.00000000000000000, -6.646953231504538984, -2.840624999385488181 ) ) ;
#26408=CARTESIAN_POINT ( 'NONE',  ( 26.75643035624999655, 3.323476615752271268, -5.278124999385450877 ) ) ;
#26413=CARTESIAN_POINT ( 'NONE',  ( 27.74126513682283601, -5.196152422706632912, 161.4741528376846134 ) ) ;
#26418=CARTESIAN_POINT ( 'NONE',  ( 18.12178482187499640, 4.985214923628404904, -6.178124999385470772 ) ) ;
#26423=CARTESIAN_POINT ( 'NONE',  ( 24.86380461455084756, 0.000000000000000000, 163.0057683059945930 ) ) ;
#26427=CARTESIAN_POINT ( 'NONE',  ( 33.82899049407978964, 6.917534487978463709, 159.0481132747639492 ) ) ;
#26438=CARTESIAN_POINT ( 'NONE',  ( 25.09912511996950713, 0.000000000000000000, 165.6954939908422944 ) ) ;
#26442=CARTESIAN_POINT ( 'NONE',  ( 15.00000000000000000, 0.000000000000000000, -8.099999999999996092 ) ) ;
#26446=CARTESIAN_POINT ( 'NONE',  ( 37.52570519453759346, -3.604726614523235284, 167.2527469918319412 ) ) ;
#26448=CARTESIAN_POINT ( 'NONE',  ( 36.60569886870491985, 3.464101615137448409, 159.5316748164241005 ) ) ;
#26453=CARTESIAN_POINT ( 'NONE',  ( 26.99999999999999289, 0.000000000000000000, -8.000000000000000000 ) ) ;
#26454=CARTESIAN_POINT ( 'NONE',  ( 20.99999999999999645, 0.000000000000000000, -8.000000000000000000 ) ) ;
#26455=CARTESIAN_POINT ( 'NONE',  ( 26.75643035624999655, 3.323476615752271712, -5.728124999385479477 ) ) ;
#26462=CARTESIAN_POINT ( 'NONE',  ( 27.50146640511176344, 5.407089921784862696, 160.1305649159599227 ) ) ;
#26475=CARTESIAN_POINT ( 'NONE',  ( 25.06157068934916765, 3.604726614523240613, 168.0608931323890829 ) ) ;
#26476=CARTESIAN_POINT ( 'NONE',  ( 26.99999999999999645, -3.464101615137751278, -3.356249998770971743 ) ) ;
#26477=( BOUNDED_CURVE ( )  B_SPLINE_CURVE ( 2, ( #10029, #21609, #32590, #6628, #18204, #33159, #7205 ),
 .UNSPECIFIED., .F., .F. ) 
 B_SPLINE_CURVE_WITH_KNOTS ( ( 3, 2, 2, 3 ),
 ( 0.4565217391304355332, 0.4637681159420298238, 0.4710144927536241144, 0.4782608695652184050 ),
 .UNSPECIFIED. ) 
 CURVE ( )  GEOMETRIC_REPRESENTATION_ITEM ( )  RATIONAL_B_SPLINE_CURVE ( ( 0.9999999999999856781, 0.8660254037844530295, 1.000000000000000000, 0.8660254037844387076, 1.000000000000000000, 0.8660254037844202779, 1.000000000000018430 ) ) 
 REPRESENTATION_ITEM ( '' )  );
#26481=DIRECTION ( 'NONE',  ( 0.08715574274765150453, 0.000000000000000000, 0.9961946980917461003 ) ) ;
#26483=EDGE_CURVE ( 'NONE', #26027, #26157, #8307, .T. ) ;
#26485=DIRECTION ( 'NONE',  ( 0.08715574274765150453, 0.000000000000000000, 0.9961946980917461003 ) ) ;
#26487=CARTESIAN_POINT ( 'NONE',  ( 24.43895185209563792, 3.604726614523236616, 160.9443272578961626 ) ) ;
#26488=CARTESIAN_POINT ( 'NONE',  ( 15.00000000000000000, 3.464101615137752166, -0.4874999999999927169 ) ) ;
#26490=CARTESIAN_POINT ( 'NONE',  ( 37.25279877505901993, 3.604726614523243278, 164.1334123434321555 ) ) ;
#26491=CARTESIAN_POINT ( 'NONE',  ( 27.91448717542667168, 5.196152422706636465, 163.4540897989176642 ) ) ;
#26498=CIRCLE ( 'NONE', #30138, 6.000000000000001776 ) ;
#26502=CARTESIAN_POINT ( 'NONE',  ( 36.91945954259546880, 3.464101615138031054, 163.1179757295544448 ) ) ;
#26504=CARTESIAN_POINT ( 'NONE',  ( 21.00000000000000000, -6.646953231504538984, -4.640624999385471128 ) ) ;
#26514=CARTESIAN_POINT ( 'NONE',  ( 37.19073179189800271, 7.347880794884117764E-16, 166.2186317273649934 ) ) ;
#26518=FACE_OUTER_BOUND ( 'NONE', #161, .T. ) ;
#26520=VECTOR ( 'NONE', #14351, 1000.000000000000000 ) ;
#26530=ORIENTED_EDGE ( 'NONE', *, *, #1751, .T. ) ;
#26531=CARTESIAN_POINT ( 'NONE',  ( 37.52897353489062482, 7.646167579472015790E-16, 167.2901042930103586 ) ) ;
#26532=CARTESIAN_POINT ( 'NONE',  ( 21.00000000000000000, -6.646953231504538984, -0.4781249993854547187 ) ) ;
#26533=EDGE_CURVE ( 'NONE', #25349, #21187, #6963, .T. ) ;
#26537=CARTESIAN_POINT ( 'NONE',  ( 25.37366570962461054, 0.000000000000000000, 168.8335072898312887 ) ) ;
#26541=VECTOR ( 'NONE', #35571, 1000.000000000000000 ) ;
#26542=ORIENTED_EDGE ( 'NONE', *, *, #33928, .T. ) ;
#26545=CARTESIAN_POINT ( 'NONE',  ( 21.00000000000000000, -6.646953231504538984, -1.378124999385478056 ) ) ;
#26548=( BOUNDED_CURVE ( )  B_SPLINE_CURVE ( 2, ( #15598, #27154, #4589, #8189, #25052, #22038, #2302 ),
 .UNSPECIFIED., .F., .F. ) 
 B_SPLINE_CURVE_WITH_KNOTS ( ( 3, 2, 2, 3 ),
 ( 0.4999999999999988898, 0.5072463768115932359, 0.5144927536231874710, 0.5217391304347818171 ),
 .UNSPECIFIED. ) 
 CURVE ( )  GEOMETRIC_REPRESENTATION_ITEM ( )  RATIONAL_B_SPLINE_CURVE ( ( 1.000000000000020428, 0.8660254037844181685, 1.000000000000000000, 0.8660254037844387076, 1.000000000000000000, 0.8660254037844530295, 0.9999999999999856781 ) ) 
 REPRESENTATION_ITEM ( '' )  );
#26553=CARTESIAN_POINT ( 'NONE',  ( 37.21357869082257253, 3.604726614523243278, 163.6851247292908909 ) ) ;
#26557=CARTESIAN_POINT ( 'NONE',  ( 27.00000000000001776, 11.99999999999999822, 49.73803434254939759 ) ) ;
#26558=EDGE_CURVE ( 'NONE', #33575, #23156, #16062, .T. ) ;
#26561=CARTESIAN_POINT ( 'NONE',  ( 31.10325711637897328, -7.209453229046475009, 165.4807572684663342 ) ) ;
#26562=ORIENTED_EDGE ( 'NONE', *, *, #8908, .T. ) ;
#26576=CARTESIAN_POINT ( 'NONE',  ( 15.12178482187499995, 0.000000000000000000, -0.07031249969274844247 ) ) ;
#26579=CARTESIAN_POINT ( 'NONE',  ( 20.99999999999999645, 0.000000000000000000, -8.000000000000000000 ) ) ;
#26589=CARTESIAN_POINT ( 'NONE',  ( 15.24356964374999990, 0.000000000000000000, -2.053124999385480542 ) ) ;
#26594=CARTESIAN_POINT ( 'NONE',  ( 15.24356964374999990, 3.323476615752268604, -4.228124999385472371 ) ) ;
#26595=CARTESIAN_POINT ( 'NONE',  ( 24.65789917220240213, 0.000000000000000000, 160.6522583305284968 ) ) ;
#26603=CARTESIAN_POINT ( 'NONE',  ( 36.76257920565016235, 3.464101615137755275, 161.3248252729892727 ) ) ;
#26608=EDGE_CURVE ( 'NONE', #16385, #8744, #27612, .T. ) ;
#26609=CARTESIAN_POINT ( 'NONE',  ( 15.24356964374999990, 3.323476615752268604, -5.690624999385482496 ) ) ;
#26616=CYLINDRICAL_SURFACE ( 'NONE', #5333, 5.999999999999994671 ) ;
#26617=CARTESIAN_POINT ( 'NONE',  ( 36.82137784845814821, 3.604726614523243278, 159.2022485878779889 ) ) ;
#26628=ORIENTED_EDGE ( 'NONE', *, *, #36955, .T. ) ;
#26629=CARTESIAN_POINT ( 'NONE',  ( 26.99999999999999645, -3.464101615137751278, -7.012500000000010836 ) ) ;
#26633=CARTESIAN_POINT ( 'NONE',  ( 24.98803303140584120, 3.604726614523236616, 167.2203538558741798 ) ) ;
#26642=CARTESIAN_POINT ( 'NONE',  ( 24.77882776526536190, -3.464101615138098111, 162.0344784741307649 ) ) ;
#26643=CARTESIAN_POINT ( 'NONE',  ( 26.75643035624999655, -3.323476615752267715, -6.253124999385469174 ) ) ;
#26650=DIRECTION ( 'NONE',  ( 0.08715574274765150453, 0.000000000000000000, 0.9961946980917461003 ) ) ;
#26651=CARTESIAN_POINT ( 'NONE',  ( 25.45210587809749825, 0.000000000000000000, 169.7300825181138748 ) ) ;
#26657=CARTESIAN_POINT ( 'NONE',  ( 15.24356964374999990, 3.323476615752268604, -0.2906249993854698177 ) ) ;
#26665=CARTESIAN_POINT ( 'NONE',  ( 34.28996860281051795, -5.407089921784861808, 166.0865723713108366 ) ) ;
#26676=CARTESIAN_POINT ( 'NONE',  ( 24.47817193633207822, 3.604726614523236616, 161.3926148720374556 ) ) ;
#26677=CARTESIAN_POINT ( 'NONE',  ( 21.00000000000000000, -6.928203230275506996, -0.3375000000000047962 ) ) ;
#26679=CARTESIAN_POINT ( 'NONE',  ( 24.83278686463658502, -3.604726614523244610, 165.4458820498982732 ) ) ;
#26681=CARTESIAN_POINT ( 'NONE',  ( 30.88019288723065259, -6.928203230275514990, 162.9311214624256365 ) ) ;
#26682=CYLINDRICAL_SURFACE ( 'NONE', #3533, 5.999999999999994671 ) ;
#26687=AXIS2_PLACEMENT_3D ( 'NONE', #20139, #20520, #402 ) ;
#26692=CARTESIAN_POINT ( 'NONE',  ( 26.75643035624999655, 7.049594010296217766E-16, -3.178124999385495641 ) ) ;
#26702=DIRECTION ( 'NONE',  ( 0.08715574274765142126, 0.000000000000000000, 0.9961946980917461003 ) ) ;
#26707=CARTESIAN_POINT ( 'NONE',  ( 34.02033052368495447, -5.407089921784855591, 163.0045950240894967 ) ) ;
#26719=CARTESIAN_POINT ( 'NONE',  ( 28.01623001071507701, 5.407089921784856479, 166.0143398515642730 ) ) ;
#26720=CARTESIAN_POINT ( 'NONE',  ( 15.24356964374999990, 3.323476615752268604, -3.778124999385444660 ) ) ;
#26721=CARTESIAN_POINT ( 'NONE',  ( 15.00000000000000000, 0.000000000000000000, -5.343749998770963572 ) ) ;
#26732=CARTESIAN_POINT ( 'NONE',  ( 21.00000000000000000, -6.646953231504538984, -1.828124999385473792 ) ) ;
#26734=CARTESIAN_POINT ( 'NONE',  ( 15.00000000000000000, 0.000000000000000000, -7.593749998770965348 ) ) ;
#26735=ADVANCED_FACE ( 'NONE', ( #27552 ), #1768, .T. ) ;
#26736=CARTESIAN_POINT ( 'NONE',  ( 25.28542051998549667, 0.000000000000000000, 167.8248601567890432 ) ) ;
#26741=CARTESIAN_POINT ( 'NONE',  ( 37.24626209435294300, -3.604726614523238837, 164.0586977410752638 ) ) ;
#26751=CARTESIAN_POINT ( 'NONE',  ( 24.98803303140584120, 3.604726614523236616, 167.2203538558741798 ) ) ;
#26753=CARTESIAN_POINT ( 'NONE',  ( 15.00000000000000000, 0.000000000000000000, -6.299999999999999822 ) ) ;
#26769=CARTESIAN_POINT ( 'NONE',  ( 25.18249928241153413, 0.000000000000000000, 169.4431132759913794 ) ) ;
#26770=FACE_OUTER_BOUND ( 'NONE', #8608, .T. ) ;
#26771=( BOUNDED_CURVE ( )  B_SPLINE_CURVE ( 2, ( #15177, #20876, #32415, #6459, #18030, #32979, #29573 ),
 .UNSPECIFIED., .F., .F. ) 
 B_SPLINE_CURVE_WITH_KNOTS ( ( 3, 2, 2, 3 ),
 ( 0.4130434782608686239, 0.4202898550724629145, 0.4275362318840573161, 0.4347826086956516067 ),
 .UNSPECIFIED. ) 
 CURVE ( )  GEOMETRIC_REPRESENTATION_ITEM ( )  RATIONAL_B_SPLINE_CURVE ( ( 1.000000000000017542, 0.8660254037844213881, 1.000000000000000000, 0.8660254037844387076, 1.000000000000000000, 0.8660254037844489217, 0.9999999999999897859 ) ) 
 REPRESENTATION_ITEM ( '' )  );
#26777=EDGE_CURVE ( 'NONE', #35535, #10416, #32531, .T. ) ;
#26780=CARTESIAN_POINT ( 'NONE',  ( 18.12178482187499640, 4.985214923628404904, -5.728124999385491911 ) ) ;
#26783=ORIENTED_EDGE ( 'NONE', *, *, #22577, .T. ) ;
#26785=CARTESIAN_POINT ( 'NONE',  ( 15.24356964374999990, 0.000000000000000000, -5.540624999385457272 ) ) ;
#26789=VECTOR ( 'NONE', #24186, 1000.000000000000000 ) ;
#26798=CARTESIAN_POINT ( 'NONE',  ( 23.87821517812499650, 4.985214923628404904, -6.253124999385489602 ) ) ;
#26802=AXIS2_PLACEMENT_3D ( 'NONE', #36671, #30999, #1804 ) ;
#26808=CARTESIAN_POINT ( 'NONE',  ( 27.55375985076035761, -5.407089921784865361, 160.7282817348149706 ) ) ;
#26820=CARTESIAN_POINT ( 'NONE',  ( 23.99999999999999645, 5.196152422706631135, -7.349999999999995204 ) ) ;
#26825=CARTESIAN_POINT ( 'NONE',  ( 28.05545009495152087, 5.407089921784856479, 166.4626274657055660 ) ) ;
#26829=VERTEX_POINT ( 'NONE', #25265 ) ;
#26836=CARTESIAN_POINT ( 'NONE',  ( 23.87821517812499650, 4.985214923628404904, -5.690624999385468286 ) ) ;
#26840=CARTESIAN_POINT ( 'NONE',  ( 33.81648353596441581, 5.196152422706631135, 162.0719374165519469 ) ) ;
#26843=CARTESIAN_POINT ( 'NONE',  ( 36.85732959234155004, 7.646167579472024665E-16, 159.6131789008408646 ) ) ;
#26849=CARTESIAN_POINT ( 'NONE',  ( 15.24356964375000167, -3.323476615752272600, -0.6656249993855035685 ) ) ;
#26857=CARTESIAN_POINT ( 'NONE',  ( 34.42070221693199272, 5.407089921784862696, 167.5808644184484706 ) ) ;
#26863=LINE ( 'NONE', #9246, #10428 ) ;
#26870=CARTESIAN_POINT ( 'NONE',  ( 18.00000000000000000, 5.196152422706630247, -0.5249999999999976907 ) ) ;
#26872=CARTESIAN_POINT ( 'NONE',  ( 37.24953043470598146, 7.646167579472024665E-16, 164.0960550422537096 ) ) ;
#26873=CARTESIAN_POINT ( 'NONE',  ( 31.01746318205820785, 6.928203230275514990, 164.5001281119201053 ) ) ;
#26885=CARTESIAN_POINT ( 'NONE',  ( 26.75643035624999655, -3.323476615752267715, -3.665624999385485694 ) ) ;
#26897=CARTESIAN_POINT ( 'NONE',  ( 25.22005371303209387, -3.464101615137879620, 167.0777141344445909 ) ) ;
#26901=CARTESIAN_POINT ( 'NONE',  ( 23.99999999999999645, 5.196152422706631135, -7.293749998770943321 ) ) ;
#26902=CARTESIAN_POINT ( 'NONE',  ( 34.07262396933355575, 5.407089921784857367, 163.6023118429445162 ) ) ;
#26907=CARTESIAN_POINT ( 'NONE',  ( 15.00000000000053468, -3.464101615138063472, -5.756249998770931242 ) ) ;
#26914=CARTESIAN_POINT ( 'NONE',  ( 37.40804494182826545, -3.604726614523235284, 165.9078841494080336 ) ) ;
#26915=CARTESIAN_POINT ( 'NONE',  ( 23.87821517812499650, 4.985214923628404904, -2.540624999385482141 ) ) ;
#26916=CARTESIAN_POINT ( 'NONE',  ( 24.00000000000000000, -5.196152422706629359, -4.743749998770946164 ) ) ;
#26917=CARTESIAN_POINT ( 'NONE',  ( 15.02283181144952628, 7.347880794884122694E-16, 50.52293445648592751 ) ) ;
#26925=CARTESIAN_POINT ( 'NONE',  ( 21.00000000000000000, -6.646953231504538984, -2.278124999385469529 ) ) ;
#26927=CARTESIAN_POINT ( 'NONE',  ( 15.00000000000000000, 0.000000000000000000, -6.243749998770947940 ) ) ;
#26928=CYLINDRICAL_SURFACE ( 'NONE', #10465, 3.999999999999996447 ) ;
#26934=CARTESIAN_POINT ( 'NONE',  ( 24.79029844004710625, 0.000000000000000000, 164.9602371345785343 ) ) ;
#26941=CARTESIAN_POINT ( 'NONE',  ( 24.91286120328598841, 0.000000000000000000, 166.3611359287700395 ) ) ;
#26950=ORIENTED_EDGE ( 'NONE', *, *, #7484, .F. ) ;
#26956=CARTESIAN_POINT ( 'NONE',  ( 20.99999999999999645, 6.928203230275506996, -1.462500000000010125 ) ) ;
#26964=AXIS2_PLACEMENT_3D ( 'NONE', #7997, #11020, #34510 ) ;
#26969=CARTESIAN_POINT ( 'NONE',  ( 23.87821517812500005, -4.985214923628404016, -3.703124999385493332 ) ) ;
#26973=EDGE_LOOP ( 'NONE', ( #35351, #22823 ) ) ;
#26976=CARTESIAN_POINT ( 'NONE',  ( 25.02395329185000250, -3.464101615137956003, 164.8362760637381541 ) ) ;
#26983=CARTESIAN_POINT ( 'NONE',  ( 24.66443585301559693, 3.464101615137752166, 160.7269729341097104 ) ) ;
#26987=CARTESIAN_POINT ( 'NONE',  ( 26.75643035624999655, -3.323476615752267271, -7.265624999385483562 ) ) ;
#27005=CARTESIAN_POINT ( 'NONE',  ( 25.36386068845838082, 0.000000000000000000, 168.7214353850716293 ) ) ;
#27010=ORIENTED_EDGE ( 'NONE', *, *, #7177, .T. ) ;
#27011=CARTESIAN_POINT ( 'NONE',  ( 18.00000000000000000, 5.196152422706630247, -7.275000000000003908 ) ) ;
#27017=CARTESIAN_POINT ( 'NONE',  ( 30.94637677943320497, -7.209453229046475009, 163.6876068119012189 ) ) ;
#27018=CARTESIAN_POINT ( 'NONE',  ( 25.43903251657820164, 3.464101615137743728, 169.5806533121757411 ) ) ;
#27024=CARTESIAN_POINT ( 'NONE',  ( 14.99999999999960387, -3.464101615137527457, -2.662500000000015188 ) ) ;
#27025=DIRECTION ( 'NONE',  ( 1.000000000000000000, 0.000000000000000000, 0.000000000000000000 ) ) ;
#27027=CARTESIAN_POINT ( 'NONE',  ( 21.00000000000000000, -6.646953231504538984, -8.578124999385442706 ) ) ;
#27030=CARTESIAN_POINT ( 'NONE',  ( 26.99999999999999289, 0.000000000000000000, -8.000000000000000000 ) ) ;
#27032=CARTESIAN_POINT ( 'NONE',  ( 30.83116778204221475, 6.928203230275506996, 162.3707619459733564 ) ) ;
#27034=CARTESIAN_POINT ( 'NONE',  ( 26.99999999999999645, 7.347880794884117764E-16, -1.124999999999987121 ) ) ;
#27035=CARTESIAN_POINT ( 'NONE',  ( 28.27727295472088542, 5.196152422706630247, 167.6007502309489041 ) ) ;
#27045=EDGE_CURVE ( 'NONE', #8971, #19908, #8212, .T. ) ;
#27048=CARTESIAN_POINT ( 'NONE',  ( 18.00000000000000355, -5.196152422706632912, -6.225000000000008527 ) ) ;
#27049=DIRECTION ( 'NONE',  ( 0.000000000000000000, 0.000000000000000000, 1.000000000000000000 ) ) ;
#27050=CARTESIAN_POINT ( 'NONE',  ( 25.02235060511272735, 3.604726614523240613, 167.6126055182478183 ) ) ;
#27059=CYLINDRICAL_SURFACE ( 'NONE', #28749, 4.000000000000000888 ) ;
#27062=VERTEX_POINT ( 'NONE', #29022 ) ;
#27064=EDGE_CURVE ( 'NONE', #21163, #31223, #37188, .T. ) ;
#27065=CARTESIAN_POINT ( 'NONE',  ( 23.99999999999999645, 5.196152422706631135, -0.5999999999999894307 ) ) ;
#27066=AXIS2_PLACEMENT_3D ( 'NONE', #22441, #13908, #25641 ) ;
#27067=CARTESIAN_POINT ( 'NONE',  ( 25.24293209539582961, 3.464101615137650025, 167.3392152414693612 ) ) ;
#27068=CARTESIAN_POINT ( 'NONE',  ( 34.28996860281051795, -5.407089921784861808, 166.0865723713108366 ) ) ;
#27069=CARTESIAN_POINT ( 'NONE',  ( 30.91941297146709644, -6.928203230275514990, 163.3794090765669011 ) ) ;
#27080=CARTESIAN_POINT ( 'NONE',  ( 21.00000000000000000, 6.646953231504538984, -7.115624999385463667 ) ) ;
#27091=CARTESIAN_POINT ( 'NONE',  ( 37.19073179189800271, 7.347880794884117764E-16, 166.2186317273649934 ) ) ;
#27095=CARTESIAN_POINT ( 'NONE',  ( 15.24356964374999990, 0.000000000000000000, -0.2531249993854844949 ) ) ;
#27096=CARTESIAN_POINT ( 'NONE',  ( 34.09877069215784218, -5.407089921784855591, 163.9011702523720544 ) ) ;
#27107=CARTESIAN_POINT ( 'NONE',  ( 37.49302179100722299, 3.604726614523238837, 166.8791739800475113 ) ) ;
#27108=CARTESIAN_POINT ( 'NONE',  ( 26.75643035624999655, 7.049594010296217766E-16, -3.065624999385479832 ) ) ;
#27112=CARTESIAN_POINT ( 'NONE',  ( 27.00000000000052580, 3.464101615137448409, -3.281249998770952025 ) ) ;
#27120=CARTESIAN_POINT ( 'NONE',  ( 18.12178482187500350, -4.985214923628407568, -1.415624999385467486 ) ) ;
#27122=CARTESIAN_POINT ( 'NONE',  ( 26.99999999999999645, 7.347880794884117764E-16, -10.06874999877094368 ) ) ;
#27123=ORIENTED_EDGE ( 'NONE', *, *, #33667, .F. ) ;
#27128=CARTESIAN_POINT ( 'NONE',  ( 30.98069435314010178, -7.209453229046482114, 164.0798584742748574 ) ) ;
#27134=CARTESIAN_POINT ( 'NONE',  ( 37.45053336641773711, 7.646167579472015790E-16, 166.3935290647278009 ) ) ;
#27136=CARTESIAN_POINT ( 'NONE',  ( 34.30346624845981296, -5.196152422706635576, 167.6381752909151999 ) ) ;
#27154=CARTESIAN_POINT ( 'NONE',  ( 36.98155800919708014, -3.464101615137448409, 163.8277644507203661 ) ) ;
#27155=CARTESIAN_POINT ( 'NONE',  ( 15.08037007377155803, 0.2408480140671711567, -8.000000000000021316 ) ) ;
#27156=CARTESIAN_POINT ( 'NONE',  ( 33.72823834632531259, 5.196152422706637353, 161.0632902835097013 ) ) ;
#27163=CARTESIAN_POINT ( 'NONE',  ( 26.75643035624999655, 7.049594010296217766E-16, -4.978124999385491023 ) ) ;
#27166=CARTESIAN_POINT ( 'NONE',  ( 25.02068495149662297, 0.000000000000000000, 164.7989187625597367 ) ) ;
#27172=CARTESIAN_POINT ( 'NONE',  ( 24.62521576877915308, 3.464101615137752166, 160.2786853199683890 ) ) ;
#27176=CARTESIAN_POINT ( 'NONE',  ( 20.99999999999999645, -6.646953231504538984, -7.790624999385473259 ) ) ;
#27190=LINE ( 'NONE', #1214, #6298 ) ;
#27200=CARTESIAN_POINT ( 'NONE',  ( 24.87037277869651319, 3.604726614523236616, 165.8754910134502722 ) ) ;
#27201=( BOUNDED_SURFACE ( )  B_SPLINE_SURFACE ( 1, 2, ( 
 ( #19144, #28211, #19705, #14000, #22726, #30694, #34273, #19888, #5451, #31430, #17034, #28572, #24807, #33527, #4711, #19335, #16291, #13439, #24989, #10589, #30874, #16478, #28024, #141, #8865, #28949, #17222, #325, #20626, #20442, #26290, #14187, #28760, #11890, #35194, #23458, #35012, #31985, #34822, #14743, #20066, #32168, #2986, #6013, #2799, #12076, #6206, #25739, #34456, #509, #17597, #14555, #14371, #29512, #11521, #20252, #26108, #23651, #20815, #34635, #29128, #3170, #11704, #23279, #31611, #8681, #9242, #17778, #25927, #37471, #9055, #23091, #29321, #3360, #32357, #31792, #14930, #5829, #17408, #26476, #6396, #17969, #8498, #37291, #11339, #22911, #5637, #30805, #13368, #13751, #22282, #19265, #36476, #36849, #5201, #24923, #8058, #33835, #10517, #11080, #1985, #13556, #31179, #10336, #19073, #28139, #25110, #19446, #24739, #25297, #16777, #10893, #27585, #22654, #5381, #34201, #7873, #33456, #30996, #21907, #4827, #27772, #22096, #19633, #30625, #36289, #36667, #16595, #16408, #1614, #8246, #13934, #10705, #27954, #4642, #13184, #33646, #7685, #5015, #37033, #19820, #2169, #22465, #34012, #28322, #2360, #7497, #25482, #31356, #16221, #1801, #17151, #18039, #28687, #9314, #768, #26927, #5566, #32425, #23021, #20179, #17334, #31727, #2727, #11268, #15378, #35259, #34569, #8609, #37222, #14301, #8428, #22838, #28878, #25854, #11452, #32615, #6470, #19997, #14484, #28504, #21264, #37402, #5756, #34386, #2912, #26038, #31541, #2547, #16961, #66, #20885, #26734, #25666, #29583, #18229, #3621, #15187, #957, #12337, #23910, #35452, #11632, #9502, #23720, #21078, #6653, #29769, #3800, #12532, #24096, #35642, #9687, #32803, #14114, #1146, #18981, #13281, #25020, #7598, #21820, #7410, #21633, #30539, #29963, #15756, #24649, #33184, #19173, #4557, #15946, #10434, #7228, #30343, #1521, #18801, #9870, #16132, #24835, #13094, #27684, #6840, #21452, #1709, #27865, #36388, #22007, #36199, #27500, #33560, #12716, #30722, #4368, #10243, #32991, #4743, #16317, #18418, #27122, #33372, #1897, #22197, #3991, #13468, #36577, #15565, #10618, #36018, #24285 ),
 ( #35830, #7044, #18611, #30155, #4184, #27307, #1337, #12907, #24472, #10057, #2271, #4924, #20093, #36946, #19544, #19915, #28416, #25396, #5115, #5479, #11367, #31092, #14215, #2456, #16694, #17247, #8162, #19736, #37317, #16505, #25214, #34301, #31274, #25580, #30903, #31456, #22938, #17062, #33745, #28788, #11547, #2825, #14029, #2088, #37132, #28053, #10992, #33929, #28242, #25765, #36765, #13662, #5300, #22752, #22563, #7784, #14396, #22380, #34484, #11178, #8344, #8527, #25953, #31639, #34110, #37496, #16880, #28600, #19363, #2637, #10807, #5666, #13848, #7970, #14582, #9270, #11919, #168, #26692, #23121, #17997, #35220, #11733, #20281, #3759, #32008, #21032, #917, #34664, #31821, #23486, #26885, #35037, #5856, #20841, #26317, #32383, #34851, #6610, #17433, #12101, #23305, #15333, #17807, #9082, #20652, #28972, #6423, #3012, #32198, #6233, #23866, #29540, #29349, #721, #3388, #14958, #26504, #354, #26134, #3579, #15141, #535, #12294, #8708, #8891, #35406, #18184, #9455, #32569, #23675, #29726, #20469, #6038, #17625, #29154, #3196, #14772, #10389, #18941, #24053, #32760, #36344, #33144, #1290, #15525, #27825, #9829, #18570, #12861, #21965, #19129, #32946, #7188, #15904, #10013, #27265, #18371, #7000, #33511, #4515, #24241, #12673, #13055, #35787, #4325, #33329, #7555, #1105, #27450, #30112, #15714, #24428, #35977, #21407, #6797, #30678, #30299, #4142, #21594, #29918, #18757, #3949, #27080, #1480, #24610, #36159, #27641, #10205, #21779, #7369, #35599, #16278, #30493, #16089, #1670, #13244, #24793, #4697, #9644, #12486, #21221, #5257, #11136, #10575, #31228, #2596, #28375, #2411, #11321, #34255, #37088, #16834, #4884, #19689, #36722, #34068, #8298, #25536, #8117, #25722, #10762, #13984, #16464, #28194, #22713, #33699, #19870, #31414, #20048, #14167, #5433, #17014, #16651, #28555, #24972, #22334, #37274, #22890, #34439, #8479, #22522, #31594, #7738, #5618, #2224, #17202, #28008, #1855, #13424, #36531, #22152, #19322, #30859, #13805, #2040, #13619, #33886, #7928, #25353, #25168, #19502, #31049, #5070, #36900, #10948, #5996, #34618, #23260 ) ),
 .UNSPECIFIED., .F., .F., .F. ) 
 B_SPLINE_SURFACE_WITH_KNOTS ( ( 2, 2 ),
 ( 3, 2, 2, 2, 2, 2, 2, 2, 2, 2, 2, 2, 2, 2, 2, 2, 2, 2, 2, 2, 2, 2, 2, 2, 2, 2, 2, 2, 2, 2, 2, 2, 2, 2, 2, 2, 2, 2, 2, 2, 2, 2, 2, 2, 2, 2, 2, 2, 2, 2, 2, 2, 2, 2, 2, 2, 2, 2, 2, 2, 2, 2, 2, 2, 2, 2, 2, 2, 2, 2, 2, 2, 2, 2, 2, 2, 2, 2, 2, 2, 2, 2, 2, 2, 2, 2, 2, 2, 2, 2, 2, 2, 2, 2, 2, 2, 2, 2, 2, 2, 2, 2, 2, 2, 2, 2, 2, 2, 2, 2, 2, 2, 2, 2, 2, 2, 2, 2, 2, 2, 2, 2, 2, 2, 2, 2, 2, 2, 2, 2, 2, 2, 2, 2, 3 ),
 ( 0.000000000000000000, 1.000000000000000000 ),
 ( 0.000000000000000000, 0.007246376811594202987, 0.01449275362318840597, 0.02173913043478260809, 0.02898550724637681195, 0.03623188405797101580, 0.04347826086956521618, 0.05072463768115942351, 0.05797101449275362389, 0.06521739130434782428, 0.07246376811594203160, 0.07971014492753622505, 0.08695652173913043237, 0.09420289855072463969, 0.1014492753623188470, 0.1086956521739130405, 0.1159420289855072478, 0.1231884057971014551, 0.1304347826086956486, 0.1376811594202898559, 0.1449275362318840632, 0.1521739130434782705, 0.1594202898550724501, 0.1666666666666666574, 0.1739130434782608647, 0.1811594202898550721, 0.1884057971014492794, 0.1956521739130434867, 0.2028985507246376940, 0.2101449275362318736, 0.2173913043478260809, 0.2246376811594202882, 0.2318840579710144956, 0.2391304347826087029, 0.2463768115942029102, 0.2536231884057971175, 0.2608695652173912971, 0.2681159420289855322, 0.2753623188405797118, 0.2826086956521738913, 0.2898550724637681264, 0.2971014492753623060, 0.3043478260869565410, 0.3115942028985507206, 0.3188405797101449002, 0.3260869565217391353, 0.3333333333333333148, 0.3405797101449275499, 0.3478260869565217295, 0.3550724637681159646, 0.3623188405797101441, 0.3695652173913043237, 0.3768115942028985588, 0.3840579710144927383, 0.3913043478260869734, 0.3985507246376811530, 0.4057971014492753881, 0.4130434782608695676, 0.4202898550724637472, 0.4275362318840579823, 0.4347826086956521618, 0.4420289855072463969, 0.4492753623188405765, 0.4565217391304347561, 0.4637681159420289911, 0.4710144927536231707, 0.4782608695652174058, 0.4855072463768115854, 0.4927536231884058204, 0.5000000000000000000, 0.5072463768115942351, 0.5144927536231883591, 0.5217391304347825942, 0.5289855072463768293, 0.5362318840579710644, 0.5434782608695651884, 0.5507246376811594235, 0.5579710144927536586, 0.5652173913043477826, 0.5724637681159420177, 0.5797101449275362528, 0.5869565217391304879, 0.5942028985507246119, 0.6014492753623188470, 0.6086956521739130821, 0.6159420289855072062, 0.6231884057971014412, 0.6304347826086956763, 0.6376811594202898004, 0.6449275362318840354, 0.6521739130434782705, 0.6594202898550725056, 0.6666666666666666297, 0.6739130434782608647, 0.6811594202898550998, 0.6884057971014492239, 0.6956521739130434590, 0.7028985507246376940, 0.7101449275362319291, 0.7173913043478260532, 0.7246376811594202882, 0.7318840579710145233, 0.7391304347826086474, 0.7463768115942028825, 0.7536231884057971175, 0.7608695652173913526, 0.7681159420289854767, 0.7753623188405797118, 0.7826086956521739468, 0.7898550724637680709, 0.7971014492753623060, 0.8043478260869565410, 0.8115942028985507761, 0.8188405797101449002, 0.8260869565217391353, 0.8333333333333333703, 0.8405797101449274944, 0.8478260869565217295, 0.8550724637681159646, 0.8623188405797101996, 0.8695652173913043237, 0.8768115942028985588, 0.8840579710144927938, 0.8913043478260869179, 0.8985507246376811530, 0.9057971014492753881, 0.9130434782608695121, 0.9202898550724637472, 0.9275362318840579823, 0.9347826086956522174, 0.9420289855072463414, 0.9492753623188405765, 0.9565217391304348116, 0.9637681159420289356, 0.9662082966761270653 ),
 .UNSPECIFIED. ) 
 GEOMETRIC_REPRESENTATION_ITEM ( )  RATIONAL_B_SPLINE_SURFACE ( (
 ( 1.000000000000000000, 0.8660254037844387076, 1.000000000000000000, 0.8660254037844387076, 1.000000000000000000, 0.8660254037844387076, 1.000000000000000000, 0.8660254037844387076, 1.000000000000000000, 0.8660254037844387076, 1.000000000000000000, 0.8660254037844387076, 1.000000000000000000, 0.8660254037844387076, 1.000000000000000000, 0.8660254037844387076, 1.000000000000000000, 0.8660254037844387076, 1.000000000000000000, 0.8660254037844387076, 1.000000000000000000, 0.8660254037844387076, 1.000000000000000000, 0.8660254037844387076, 1.000000000000000000, 0.8660254037844387076, 1.000000000000000000, 0.8660254037844387076, 1.000000000000000000, 0.8660254037844387076, 1.000000000000000000, 0.8660254037844387076, 1.000000000000000000, 0.8660254037844387076, 1.000000000000000000, 0.8660254037844387076, 1.000000000000000000, 0.8660254037844387076, 1.000000000000000000, 0.8660254037844387076, 1.000000000000000000, 0.8660254037844387076, 1.000000000000000000, 0.8660254037844387076, 1.000000000000000000, 0.8660254037844387076, 1.000000000000000000, 0.8660254037844387076, 1.000000000000000000, 0.8660254037844387076, 1.000000000000000000, 0.8660254037844387076, 1.000000000000000000, 0.8660254037844387076, 1.000000000000000000, 0.8660254037844387076, 1.000000000000000000, 0.8660254037844387076, 1.000000000000000000, 0.8660254037844387076, 1.000000000000000000, 0.8660254037844387076, 1.000000000000000000, 0.8660254037844387076, 1.000000000000000000, 0.8660254037844387076, 1.000000000000000000, 0.8660254037844387076, 1.000000000000000000, 0.8660254037844387076, 1.000000000000000000, 0.8660254037844387076, 1.000000000000000000, 0.8660254037844387076, 1.000000000000000000, 0.8660254037844387076, 1.000000000000000000, 0.8660254037844387076, 1.000000000000000000, 0.8660254037844387076, 1.000000000000000000, 0.8660254037844387076, 1.000000000000000000, 0.8660254037844387076, 1.000000000000000000, 0.8660254037844387076, 1.000000000000000000, 0.8660254037844387076, 1.000000000000000000, 0.8660254037844387076, 1.000000000000000000, 0.8660254037844387076, 1.000000000000000000, 0.8660254037844387076, 1.000000000000000000, 0.8660254037844387076, 1.000000000000000000, 0.8660254037844387076, 1.000000000000000000, 0.8660254037844387076, 1.000000000000000000, 0.8660254037844387076, 1.000000000000000000, 0.8660254037844387076, 1.000000000000000000, 0.8660254037844387076, 1.000000000000000000, 0.8660254037844387076, 1.000000000000000000, 0.8660254037844387076, 1.000000000000000000, 0.8660254037844387076, 1.000000000000000000, 0.8660254037844387076, 1.000000000000000000, 0.8660254037844387076, 1.000000000000000000, 0.8660254037844387076, 1.000000000000000000, 0.8660254037844387076, 1.000000000000000000, 0.8660254037844387076, 1.000000000000000000, 0.8660254037844387076, 1.000000000000000000, 0.8660254037844387076, 1.000000000000000000, 0.8660254037844387076, 1.000000000000000000, 0.8660254037844387076, 1.000000000000000000, 0.8660254037844387076, 1.000000000000000000, 0.8660254037844387076, 1.000000000000000000, 0.8660254037844387076, 1.000000000000000000, 0.8660254037844387076, 1.000000000000000000, 0.8660254037844387076, 1.000000000000000000, 0.8660254037844387076, 1.000000000000000000, 0.8660254037844387076, 1.000000000000000000, 0.8660254037844387076, 1.000000000000000000, 0.8660254037844387076, 1.000000000000000000, 0.8660254037844387076, 1.000000000000000000, 0.8660254037844387076, 1.000000000000000000, 0.8660254037844387076, 1.000000000000000000, 0.8660254037844387076, 1.000000000000000000, 0.8660254037844387076, 1.000000000000000000, 0.8660254037844387076, 1.000000000000000000, 0.8660254037844387076, 1.000000000000000000, 0.8660254037844387076, 1.000000000000000000, 0.8660254037844387076, 1.000000000000000000, 0.8660254037844387076, 1.000000000000000000, 0.8660254037844387076, 1.000000000000000000, 0.8660254037844387076, 1.000000000000000000, 0.8660254037844387076, 1.000000000000000000, 0.8660254037844387076, 1.000000000000000000, 0.8660254037844387076, 1.000000000000000000, 0.8660254037844387076, 1.000000000000000000, 0.8660254037844387076, 1.000000000000000000, 0.8660254037844387076, 1.000000000000000000, 0.8660254037844387076, 1.000000000000000000, 0.8660254037844387076, 1.000000000000000000, 0.8660254037844387076, 1.000000000000000000, 0.8660254037844387076, 1.000000000000000000, 0.8660254037844387076, 1.000000000000000000, 0.8660254037844387076, 1.000000000000000000, 0.8660254037844387076, 1.000000000000000000, 0.8660254037844387076, 1.000000000000000000, 0.8660254037844387076, 1.000000000000000000, 0.8660254037844387076, 1.000000000000000000, 0.8660254037844387076, 1.000000000000000000, 0.8660254037844387076, 1.000000000000000000, 0.8660254037844387076, 1.000000000000000000, 0.8660254037844387076, 1.000000000000000000, 0.8660254037844387076, 1.000000000000000000, 0.8660254037844387076, 1.000000000000000000, 0.8660254037844387076, 1.000000000000000000, 0.8660254037844387076, 1.000000000000000000, 0.8660254037844387076, 1.000000000000000000, 0.8660254037844387076, 1.000000000000000000, 0.8660254037844387076, 1.000000000000000000, 0.8660254037844387076, 1.000000000000000000, 0.8660254037844387076, 1.000000000000000000, 0.8660254037844387076, 1.000000000000000000, 0.8660254037844387076, 1.000000000000000000, 0.8660254037844387076, 1.000000000000000000, 0.8660254037844387076, 1.000000000000000000, 0.8660254037844387076, 1.000000000000000000, 0.8660254037844387076, 1.000000000000000000, 0.8660254037844387076, 1.000000000000000000, 0.8660254037844387076, 1.000000000000000000, 0.8660254037844387076, 1.000000000000000000, 0.8660254037844387076, 1.000000000000000000, 0.8660254037844387076, 1.000000000000000000, 0.8660254037844387076, 1.000000000000000000, 0.8660254037844387076, 1.000000000000000000, 0.8660254037844387076, 1.000000000000000000, 0.8660254037844387076, 1.000000000000000000, 0.8660254037844387076, 1.000000000000000000, 0.8660254037844387076, 1.000000000000000000, 0.8660254037844387076, 1.000000000000000000, 0.9548847324609573972, 0.9401541411607521326),
 ( 1.000000000000000000, 0.8660254037844387076, 1.000000000000000000, 0.8660254037844387076, 1.000000000000000000, 0.8660254037844387076, 1.000000000000000000, 0.8660254037844387076, 1.000000000000000000, 0.8660254037844387076, 1.000000000000000000, 0.8660254037844387076, 1.000000000000000000, 0.8660254037844387076, 1.000000000000000000, 0.8660254037844387076, 1.000000000000000000, 0.8660254037844387076, 1.000000000000000000, 0.8660254037844387076, 1.000000000000000000, 0.8660254037844387076, 1.000000000000000000, 0.8660254037844387076, 1.000000000000000000, 0.8660254037844387076, 1.000000000000000000, 0.8660254037844387076, 1.000000000000000000, 0.8660254037844387076, 1.000000000000000000, 0.8660254037844387076, 1.000000000000000000, 0.8660254037844387076, 1.000000000000000000, 0.8660254037844387076, 1.000000000000000000, 0.8660254037844387076, 1.000000000000000000, 0.8660254037844387076, 1.000000000000000000, 0.8660254037844387076, 1.000000000000000000, 0.8660254037844387076, 1.000000000000000000, 0.8660254037844387076, 1.000000000000000000, 0.8660254037844387076, 1.000000000000000000, 0.8660254037844387076, 1.000000000000000000, 0.8660254037844387076, 1.000000000000000000, 0.8660254037844387076, 1.000000000000000000, 0.8660254037844387076, 1.000000000000000000, 0.8660254037844387076, 1.000000000000000000, 0.8660254037844387076, 1.000000000000000000, 0.8660254037844387076, 1.000000000000000000, 0.8660254037844387076, 1.000000000000000000, 0.8660254037844387076, 1.000000000000000000, 0.8660254037844387076, 1.000000000000000000, 0.8660254037844387076, 1.000000000000000000, 0.8660254037844387076, 1.000000000000000000, 0.8660254037844387076, 1.000000000000000000, 0.8660254037844387076, 1.000000000000000000, 0.8660254037844387076, 1.000000000000000000, 0.8660254037844387076, 1.000000000000000000, 0.8660254037844387076, 1.000000000000000000, 0.8660254037844387076, 1.000000000000000000, 0.8660254037844387076, 1.000000000000000000, 0.8660254037844387076, 1.000000000000000000, 0.8660254037844387076, 1.000000000000000000, 0.8660254037844387076, 1.000000000000000000, 0.8660254037844387076, 1.000000000000000000, 0.8660254037844387076, 1.000000000000000000, 0.8660254037844387076, 1.000000000000000000, 0.8660254037844387076, 1.000000000000000000, 0.8660254037844387076, 1.000000000000000000, 0.8660254037844387076, 1.000000000000000000, 0.8660254037844387076, 1.000000000000000000, 0.8660254037844387076, 1.000000000000000000, 0.8660254037844387076, 1.000000000000000000, 0.8660254037844387076, 1.000000000000000000, 0.8660254037844387076, 1.000000000000000000, 0.8660254037844387076, 1.000000000000000000, 0.8660254037844387076, 1.000000000000000000, 0.8660254037844387076, 1.000000000000000000, 0.8660254037844387076, 1.000000000000000000, 0.8660254037844387076, 1.000000000000000000, 0.8660254037844387076, 1.000000000000000000, 0.8660254037844387076, 1.000000000000000000, 0.8660254037844387076, 1.000000000000000000, 0.8660254037844387076, 1.000000000000000000, 0.8660254037844387076, 1.000000000000000000, 0.8660254037844387076, 1.000000000000000000, 0.8660254037844387076, 1.000000000000000000, 0.8660254037844387076, 1.000000000000000000, 0.8660254037844387076, 1.000000000000000000, 0.8660254037844387076, 1.000000000000000000, 0.8660254037844387076, 1.000000000000000000, 0.8660254037844387076, 1.000000000000000000, 0.8660254037844387076, 1.000000000000000000, 0.8660254037844387076, 1.000000000000000000, 0.8660254037844387076, 1.000000000000000000, 0.8660254037844387076, 1.000000000000000000, 0.8660254037844387076, 1.000000000000000000, 0.8660254037844387076, 1.000000000000000000, 0.8660254037844387076, 1.000000000000000000, 0.8660254037844387076, 1.000000000000000000, 0.8660254037844387076, 1.000000000000000000, 0.8660254037844387076, 1.000000000000000000, 0.8660254037844387076, 1.000000000000000000, 0.8660254037844387076, 1.000000000000000000, 0.8660254037844387076, 1.000000000000000000, 0.8660254037844387076, 1.000000000000000000, 0.8660254037844387076, 1.000000000000000000, 0.8660254037844387076, 1.000000000000000000, 0.8660254037844387076, 1.000000000000000000, 0.8660254037844387076, 1.000000000000000000, 0.8660254037844387076, 1.000000000000000000, 0.8660254037844387076, 1.000000000000000000, 0.8660254037844387076, 1.000000000000000000, 0.8660254037844387076, 1.000000000000000000, 0.8660254037844387076, 1.000000000000000000, 0.8660254037844387076, 1.000000000000000000, 0.8660254037844387076, 1.000000000000000000, 0.8660254037844387076, 1.000000000000000000, 0.8660254037844387076, 1.000000000000000000, 0.8660254037844387076, 1.000000000000000000, 0.8660254037844387076, 1.000000000000000000, 0.8660254037844387076, 1.000000000000000000, 0.8660254037844387076, 1.000000000000000000, 0.8660254037844387076, 1.000000000000000000, 0.8660254037844387076, 1.000000000000000000, 0.8660254037844387076, 1.000000000000000000, 0.8660254037844387076, 1.000000000000000000, 0.8660254037844387076, 1.000000000000000000, 0.8660254037844387076, 1.000000000000000000, 0.8660254037844387076, 1.000000000000000000, 0.8660254037844387076, 1.000000000000000000, 0.8660254037844387076, 1.000000000000000000, 0.8660254037844387076, 1.000000000000000000, 0.8660254037844387076, 1.000000000000000000, 0.8660254037844387076, 1.000000000000000000, 0.8660254037844387076, 1.000000000000000000, 0.8660254037844387076, 1.000000000000000000, 0.8660254037844387076, 1.000000000000000000, 0.8660254037844387076, 1.000000000000000000, 0.8660254037844387076, 1.000000000000000000, 0.8660254037844387076, 1.000000000000000000, 0.8660254037844387076, 1.000000000000000000, 0.8660254037844387076, 1.000000000000000000, 0.8660254037844387076, 1.000000000000000000, 0.8660254037844387076, 1.000000000000000000, 0.8660254037844387076, 1.000000000000000000, 0.8660254037844387076, 1.000000000000000000, 0.8660254037844387076, 1.000000000000000000, 0.8660254037844387076, 1.000000000000000000, 0.8660254037844387076, 1.000000000000000000, 0.8660254037844387076, 1.000000000000000000, 0.9548847324609573972, 0.9401541411607521326) ) ) 
 REPRESENTATION_ITEM ( '' )  SURFACE ( )  );
#27202=FACE_OUTER_BOUND ( 'NONE', #34887, .T. ) ;
#27204=EDGE_CURVE ( 'NONE', #19175, #21723, #35408, .T. ) ;
#27211=CARTESIAN_POINT ( 'NONE',  ( 26.75643035624999655, 3.323476615752271268, -0.3281249993854667424 ) ) ;
#27214=CARTESIAN_POINT ( 'NONE',  ( 15.24356964374999990, 0.000000000000000000, -8.690624999385471838 ) ) ;
#27221=CARTESIAN_POINT ( 'NONE',  ( 25.29849388150476130, -3.464101615137757051, 167.9742893627271769 ) ) ;
#27225=( BOUNDED_CURVE ( )  B_SPLINE_CURVE ( 2, ( #18854, #30402, #36443, #10671, #1581, #30961, #22250 ),
 .UNSPECIFIED., .F., .F. ) 
 B_SPLINE_CURVE_WITH_KNOTS ( ( 3, 2, 2, 3 ),
 ( 0.6739130434782596435, 0.6811594202898539896, 0.6884057971014481137, 0.6956521739130424598 ),
 .UNSPECIFIED. ) 
 CURVE ( )  GEOMETRIC_REPRESENTATION_ITEM ( )  RATIONAL_B_SPLINE_CURVE ( ( 1.000000000000022649, 0.8660254037844161701, 1.000000000000000000, 0.8660254037844387076, 1.000000000000000000, 0.8660254037844571373, 0.9999999999999815703 ) ) 
 REPRESENTATION_ITEM ( '' )  );
#27232=VERTEX_POINT ( 'NONE', #26753 ) ;
#27235=CARTESIAN_POINT ( 'NONE',  ( 26.99999999999999645, 7.347880794884117764E-16, -4.275000000000001243 ) ) ;
#27236=CARTESIAN_POINT ( 'NONE',  ( 31.13757469008587719, -7.209453229046482114, 165.8730089308399442 ) ) ;
#27246=CARTESIAN_POINT ( 'NONE',  ( 26.99999999999999645, 7.347880794884117764E-16, -7.818749998770941012 ) ) ;
#27250=CARTESIAN_POINT ( 'NONE',  ( 15.02283181144952628, 7.347880794884122694E-16, 50.52293445648592751 ) ) ;
#27252=CARTESIAN_POINT ( 'NONE',  ( 18.00000000000000000, 5.196152422706630247, -0.9750000000000036415 ) ) ;
#27254=CARTESIAN_POINT ( 'NONE',  ( 37.05016167317072728, -3.604726614523238837, 161.8172596703688271 ) ) ;
#27255=CARTESIAN_POINT ( 'NONE',  ( 27.80990028412949755, -5.196152422706638241, 162.2586561612075116 ) ) ;
#27265=CARTESIAN_POINT ( 'NONE',  ( 15.24356964374999990, 0.000000000000000000, -6.103124999385478588 ) ) ;
#27277=CARTESIAN_POINT ( 'NONE',  ( 37.25770128558855987, 3.604726614523238837, 164.1894482951998100 ) ) ;
#27281=DIRECTION ( 'NONE',  ( 0.08715574274765150453, 0.000000000000000000, 0.9961946980917461003 ) ) ;
#27283=CARTESIAN_POINT ( 'NONE',  ( 26.99999999999999645, 7.347880794884117764E-16, -4.218749998770948473 ) ) ;
#27289=CARTESIAN_POINT ( 'NONE',  ( 34.34716455898865206, 5.407089921784857367, 166.7403251419335390 ) ) ;
#27290=CARTESIAN_POINT ( 'NONE',  ( 18.12178482187499640, 4.985214923628404904, -2.915624999385468819 ) ) ;
#27292=CARTESIAN_POINT ( 'NONE',  ( 25.18083362879568199, -3.464101615137894719, 166.6294265203033262 ) ) ;
#27293=CARTESIAN_POINT ( 'NONE',  ( 37.37702719191401002, 7.347880794884125653E-16, 168.3479978933117422 ) ) ;
#27294=CARTESIAN_POINT ( 'NONE',  ( 26.99999999999999645, 7.347880794884117764E-16, -3.318749998770964549 ) ) ;
#27304=CARTESIAN_POINT ( 'NONE',  ( 26.75643035624999655, -3.323476615752267715, -1.753124999385447857 ) ) ;
#27307=CARTESIAN_POINT ( 'NONE',  ( 26.75643035624999655, 3.323476615752271712, -0.4406249993854897129 ) ) ;
#27313=CARTESIAN_POINT ( 'NONE',  ( 27.94596069312478903, -5.407089921784865361, 165.2111578762278157 ) ) ;
#27322=CARTESIAN_POINT ( 'NONE',  ( 31.12286715849720409, 7.209453229046475009, 165.7049010755369807 ) ) ;
#27332=EDGE_LOOP ( 'NONE', ( #12228, #7129, #8656, #10638 ) ) ;
#27336=VECTOR ( 'NONE', #20350, 1000.000000000000000 ) ;
#27349=CARTESIAN_POINT ( 'NONE',  ( 23.87821517812500005, -4.985214923628404016, -4.153124999385471305 ) ) ;
#27352=CARTESIAN_POINT ( 'NONE',  ( 15.24356964374999990, 0.000000000000000000, -6.890624999385474680 ) ) ;
#27358=CARTESIAN_POINT ( 'NONE',  ( 27.64975160693779443, 5.196152422706630247, 160.4281484046883293 ) ) ;
#27363=CARTESIAN_POINT ( 'NONE',  ( 18.00000000000000000, 5.196152422706630247, -2.324999999999993960 ) ) ;
#27366=CARTESIAN_POINT ( 'NONE',  ( 21.00000000000000355, 0.000000000000000000, 50.00000000000001421 ) ) ;
#27375=CARTESIAN_POINT ( 'NONE',  ( 30.84097280299421229, -6.928203230275514990, 162.4828338482843151 ) ) ;
#27377=CARTESIAN_POINT ( 'NONE',  ( 28.34590810202754696, 5.196152422706636465, 168.3852535544717739 ) ) ;
#27382=ORIENTED_EDGE ( 'NONE', *, *, #35289, .T. ) ;
#27383=CARTESIAN_POINT ( 'NONE',  ( 20.99999999999999645, -6.928203230275506996, -4.387499999999998401 ) ) ;
#27386=CARTESIAN_POINT ( 'NONE',  ( 37.29038468911893034, -3.604726614523235284, 164.5630213069841830 ) ) ;
#27391=EDGE_LOOP ( 'NONE', ( #23143, #35844, #29815, #33496, #6995 ) ) ;
#27396=FACE_OUTER_BOUND ( 'NONE', #32447, .T. ) ;
#27397=CARTESIAN_POINT ( 'NONE',  ( 21.00000000000000000, 6.646953231504538984, -7.903124999385464200 ) ) ;
#27404=CARTESIAN_POINT ( 'NONE',  ( 31.32141883499775403, -6.928203230275506996, 167.9743571227394341 ) ) ;
#27414=DIRECTION ( 'NONE',  ( 0.08715574274765150453, 0.000000000000000000, 0.9961946980917461003 ) ) ;
#27416=EDGE_CURVE ( 'NONE', #30158, #16958, #35470, .T. ) ;
#27418=CARTESIAN_POINT ( 'NONE',  ( 24.86873860851999041, 0.000000000000000000, 165.8568123628610920 ) ) ;
#27434=CARTESIAN_POINT ( 'NONE',  ( 26.99999999999999645, 3.464101615137755275, -1.537500000000004086 ) ) ;
#27437=CARTESIAN_POINT ( 'NONE',  ( 37.01747826964035681, 3.604726614523243278, 161.4436866585844541 ) ) ;
#27438=CARTESIAN_POINT ( 'NONE',  ( 36.71355410024750654, 3.464101615137759271, 160.7644657540882918 ) ) ;
#27441=EDGE_CURVE ( 'NONE', #37335, #32501, #314, .T. ) ;
#27447=DIRECTION ( 'NONE',  ( 0.08715574274765150453, 0.000000000000000000, 0.9961946980917461003 ) ) ;
#27450=CARTESIAN_POINT ( 'NONE',  ( 15.24356964374999990, 3.323476615752268604, -6.590624999385473970 ) ) ;
#27460=CARTESIAN_POINT ( 'NONE',  ( 21.00000000000000355, 0.000000000000000000, 50.00000000000001421 ) ) ;
#27465=CIRCLE ( 'NONE', #17785, 3.999999999999996447 ) ;
#27467=CARTESIAN_POINT ( 'NONE',  ( 24.55661210480496948, 3.604726614523236616, 162.2891901003200132 ) ) ;
#27471=EDGE_CURVE ( 'NONE', #15328, #30939, #10260, .T. ) ;
#27478=CARTESIAN_POINT ( 'NONE',  ( 30.92676673731498482, 7.209453229046475009, 163.4634630048305439 ) ) ;
#27479=CARTESIAN_POINT ( 'NONE',  ( 26.75643035624999655, 3.323476615752271712, -2.128124999385482052 ) ) ;
#27482=CARTESIAN_POINT ( 'NONE',  ( 34.42112650116913386, -5.196152422706635576, 168.9830381333390505 ) ) ;
#27497=CARTESIAN_POINT ( 'NONE',  ( 23.87821517812500005, -4.985214923628404016, -3.140624999385472016 ) ) ;
#27500=CARTESIAN_POINT ( 'NONE',  ( 24.00000000000000000, -5.196152422706629359, -9.693749998770956111 ) ) ;
#27501=ORIENTED_EDGE ( 'NONE', *, *, #9725, .T. ) ;
#27503=ORIENTED_EDGE ( 'NONE', *, *, #10396, .F. ) ;
#27506=CARTESIAN_POINT ( 'NONE',  ( 24.47326942580252407, 3.604726614523240613, 161.3365789202697727 ) ) ;
#27514=EDGE_LOOP ( 'NONE', ( #36083, #36154, #13109, #15700 ) ) ;
#27519=ADVANCED_FACE ( 'NONE', ( #36403 ), #4384, .T. ) ;
#27523=DIRECTION ( 'NONE',  ( 1.000000000000000000, 0.000000000000000000, 0.000000000000000000 ) ) ;
#27528=FACE_OUTER_BOUND ( 'NONE', #7600, .T. ) ;
#27538=CARTESIAN_POINT ( 'NONE',  ( 23.87821517812500005, -4.985214923628404016, -5.053124999385483207 ) ) ;
#27541=CARTESIAN_POINT ( 'NONE',  ( 15.24356964374999990, 0.000000000000000000, -6.440624999385469174 ) ) ;
#27547=CARTESIAN_POINT ( 'NONE',  ( 24.67097253372167387, -3.464101615137757051, 160.8016875364665736 ) ) ;
#27552=FACE_OUTER_BOUND ( 'NONE', #9078, .T. ) ;
#27559=ADVANCED_FACE ( 'NONE', ( #33761 ), #8357, .T. ) ;
#27574=CYLINDRICAL_SURFACE ( 'NONE', #20844, 6.000000000000001776 ) ;
#27578=CARTESIAN_POINT ( 'NONE',  ( 34.02033052368495447, -5.407089921784855591, 163.0045950240894967 ) ) ;
#27581=ORIENTED_EDGE ( 'NONE', *, *, #18191, .F. ) ;
#27585=CARTESIAN_POINT ( 'NONE',  ( 23.99999999999999645, 5.196152422706631135, -4.593749998770962684 ) ) ;
#27586=CARTESIAN_POINT ( 'NONE',  ( 26.75643035624999655, 3.323476615752271268, -1.228124999385458160 ) ) ;
#27589=CARTESIAN_POINT ( 'NONE',  ( 18.12178482187500350, -4.985214923628407568, -8.165624999385473259 ) ) ;
#27592=CARTESIAN_POINT ( 'NONE',  ( 33.76419009031582874, -5.196152422706629359, 161.4742205976968989 ) ) ;
#27595=CARTESIAN_POINT ( 'NONE',  ( 37.14824336730853105, -3.464101615137751278, 165.7329868120451977 ) ) ;
#27601=CARTESIAN_POINT ( 'NONE',  ( 23.87821517812500005, -4.985214923628404016, -1.903124999385497063 ) ) ;
#27605=ORIENTED_EDGE ( 'NONE', *, *, #16987, .T. ) ;
#27610=CARTESIAN_POINT ( 'NONE',  ( 34.14616162727688931, 5.407089921784862696, 164.4428511194594478 ) ) ;
#27612=CIRCLE ( 'NONE', #25208, 3.999999999999996447 ) ;
#27621=LINE ( 'NONE', #13405, #11817 ) ;
#27626=ORIENTED_EDGE ( 'NONE', *, *, #1145, .F. ) ;
#27627=CARTESIAN_POINT ( 'NONE',  ( 15.00000000000000000, 3.464101615137752166, -3.187499999999998668 ) ) ;
#27628=CARTESIAN_POINT ( 'NONE',  ( 37.13187018199665346, 7.646167579472024665E-16, 162.7511921998298590 ) ) ;
#27629=CARTESIAN_POINT ( 'NONE',  ( 30.68409246604844043, -6.928203230275514990, 160.6896833917191714 ) ) ;
#27638=CARTESIAN_POINT ( 'NONE',  ( 20.99999999999999645, -6.928203230275506996, -3.937500000000003109 ) ) ;
#27641=CARTESIAN_POINT ( 'NONE',  ( 26.75643035624999655, -3.323476615752267715, -7.265624999385483562 ) ) ;
#27656=CARTESIAN_POINT ( 'NONE',  ( 37.05506418370026722, -3.604726614523235284, 161.8732956221364532 ) ) ;
#27662=ADVANCED_FACE ( 'NONE', ( #31467 ), #22394, .T. ) ;
#27666=VERTEX_POINT ( 'NONE', #5490 ) ;
#27667=CARTESIAN_POINT ( 'NONE',  ( 27.93778984224218931, 5.407089921784856479, 165.1177646232817153 ) ) ;
#27668=CARTESIAN_POINT ( 'NONE',  ( 21.00000000000000000, -6.646953231504538984, -4.978124999385476812 ) ) ;
#27670=CARTESIAN_POINT ( 'NONE',  ( 28.34590810202754696, 5.196152422706636465, 168.3852535544717739 ) ) ;
#27680=CARTESIAN_POINT ( 'NONE',  ( 15.24356964374999990, 3.323476615752268604, -4.678124999385468108 ) ) ;
#27684=CARTESIAN_POINT ( 'NONE',  ( 15.00000000000000000, 0.000000000000000000, -9.393749998770960730 ) ) ;
#27689=CARTESIAN_POINT ( 'NONE',  ( 27.74986027194257332, -5.407089921784865361, 162.9697198055213789 ) ) ;
#27692=SURFACE_STYLE_USAGE ( .BOTH. , #1531 ) ;
#27703=DIRECTION ( 'NONE',  ( 0.9961946980917462113, 0.000000000000000000, -0.08715574274765118534 ) ) ;
#27706=VERTEX_POINT ( 'NONE', #22950 ) ;
#27709=( BOUNDED_CURVE ( )  B_SPLINE_CURVE ( 2, ( #18291, #15442, #9563, #12402, #29265, #29458, #26423 ),
 .UNSPECIFIED., .F., .F. ) 
 B_SPLINE_CURVE_WITH_KNOTS ( ( 3, 2, 2, 3 ),
 ( 0.6304347826086944551, 0.6376811594202886901, 0.6449275362318829252, 0.6521739130434772713 ),
 .UNSPECIFIED. ) 
 CURVE ( )  GEOMETRIC_REPRESENTATION_ITEM ( )  RATIONAL_B_SPLINE_CURVE ( ( 1.000000000000022649, 0.8660254037844161701, 1.000000000000000000, 0.8660254037844387076, 1.000000000000000000, 0.8660254037844571373, 0.9999999999999815703 ) ) 
 REPRESENTATION_ITEM ( '' )  );
#27712=CARTESIAN_POINT ( 'NONE',  ( 25.09912511996950713, 0.000000000000000000, 165.6954939908422944 ) ) ;
#27715=FACE_OUTER_BOUND ( 'NONE', #24475, .T. ) ;
#27717=CARTESIAN_POINT ( 'NONE',  ( 26.99999999999999645, 7.347880794884117764E-16, -7.424999999999987388 ) ) ;
#27724=CARTESIAN_POINT ( 'NONE',  ( 15.24356964374999990, 3.323476615752268604, -6.140624999385478233 ) ) ;
#27728=CARTESIAN_POINT ( 'NONE',  ( 15.24356964374999990, 3.323476615752268604, -7.828124999385471128 ) ) ;
#27731=CARTESIAN_POINT ( 'NONE',  ( 28.24664800560418243, 5.407089921784862696, 168.6480295846443482 ) ) ;
#27748=ORIENTED_EDGE ( 'NONE', *, *, #32055, .F. ) ;
#27752=CARTESIAN_POINT ( 'NONE',  ( 33.83282523762249383, -5.196152422706635576, 162.2587239212197971 ) ) ;
#27762=EDGE_CURVE ( 'NONE', #37335, #20530, #5678, .T. ) ;
#27764=CARTESIAN_POINT ( 'NONE',  ( 37.17926111711567927, 3.604726614523238837, 163.2928730669172523 ) ) ;
#27772=CARTESIAN_POINT ( 'NONE',  ( 15.00000000000000000, 3.464101615137752166, -4.931249998770940834 ) ) ;
#27775=CARTESIAN_POINT ( 'NONE',  ( 15.24356964374999990, 0.000000000000000000, -7.790624999385459049 ) ) ;
#27785=CARTESIAN_POINT ( 'NONE',  ( 37.10902328307209785, -3.464101615137751278, 165.2846991979039615 ) ) ;
#27789=CARTESIAN_POINT ( 'NONE',  ( 18.12178482187499640, 4.985214923628404904, -3.028124999385484184 ) ) ;
#27794=CARTESIAN_POINT ( 'NONE',  ( 24.89321967762106169, 0.000000000000000000, 163.3419840153761982 ) ) ;
#27798=CARTESIAN_POINT ( 'NONE',  ( 34.09386818162830224, -5.407089921784861808, 163.8451343006043999 ) ) ;
#27814=CARTESIAN_POINT ( 'NONE',  ( 26.99999999999999645, 3.464101615137755275, -1.987499999999999600 ) ) ;
#27815=CARTESIAN_POINT ( 'NONE',  ( 27.77600699476686330, 5.407089921784862696, 163.2685782149489171 ) ) ;
#27816=CARTESIAN_POINT ( 'NONE',  ( 24.69385091608581462, 3.464101615137757051, 161.0631886434913156 ) ) ;
#27818=CARTESIAN_POINT ( 'NONE',  ( 21.00000000000000355, 0.000000000000000000, 50.00000000000001421 ) ) ;
#27825=CARTESIAN_POINT ( 'NONE',  ( 18.12178482187499640, 4.985214923628404904, -5.728124999385491911 ) ) ;
#27828=CARTESIAN_POINT ( 'NONE',  ( 26.99999999999946354, 3.464101615138061696, -7.387499999999973532 ) ) ;
#27837=CARTESIAN_POINT ( 'NONE',  ( 24.63832061363088854, 0.000000000000000000, 163.2231226297810451 ) ) ;
#27846=ORIENTED_EDGE ( 'NONE', *, *, #31954, .T. ) ;
#27847=CARTESIAN_POINT ( 'NONE',  ( 24.75271252598717808, 3.604726614523236616, 164.5306281710264216 ) ) ;
#27848=CARTESIAN_POINT ( 'NONE',  ( 18.12178482187499640, 4.985214923628404904, -4.715624999385465088 ) ) ;
#27850=CARTESIAN_POINT ( 'NONE',  ( 15.50407758876934672, -2.353417321935399098, -8.000000000000001776 ) ) ;
#27851=CARTESIAN_POINT ( 'NONE',  ( 37.29531868308808384, -3.464101615137755275, 167.4140653638507388 ) ) ;
#27862=CARTESIAN_POINT ( 'NONE',  ( 18.12178482187500350, -4.985214923628407568, -5.015624999385459581 ) ) ;
#27865=CARTESIAN_POINT ( 'NONE',  ( 23.99999999999999645, 5.196152422706631135, -9.543749998770945098 ) ) ;
#27879=ORIENTED_EDGE ( 'NONE', *, *, #22340, .F. ) ;
#27899=CARTESIAN_POINT ( 'NONE',  ( 37.13843834614275607, -3.464101615137510137, 165.6209149072855098 ) ) ;
#27905=CARTESIAN_POINT ( 'NONE',  ( 15.24356964374999990, 0.000000000000000000, -7.453124999385495997 ) ) ;
#27907=ORIENTED_EDGE ( 'NONE', *, *, #28617, .T. ) ;
#27910=EDGE_CURVE ( 'NONE', #18435, #2079, #28876, .T. ) ;
#27918=CARTESIAN_POINT ( 'NONE',  ( 15.00000000000000000, 0.000000000000000000, -6.750000000000006217 ) ) ;
#27919=CARTESIAN_POINT ( 'NONE',  ( 26.99999999999976197, -3.464101615137889834, -2.906249998770947141 ) ) ;
#27929=ORIENTED_EDGE ( 'NONE', *, *, #1898, .T. ) ;
#27932=ADVANCED_FACE ( 'NONE', ( #3402 ), #23316, .T. ) ;
#27935=CARTESIAN_POINT ( 'NONE',  ( 31.26258870864309003, 6.928203230275506996, 167.3019257015274945 ) ) ;
#27941=ORIENTED_EDGE ( 'NONE', *, *, #32869, .F. ) ;
#27945=ADVANCED_FACE ( 'NONE', ( #26518 ), #3773, .T. ) ;
#27947=CARTESIAN_POINT ( 'NONE',  ( 37.05506418370026722, -3.604726614523235284, 161.8732956221364532 ) ) ;
#27948=CARTESIAN_POINT ( 'NONE',  ( 18.12178482187499640, 4.985214923628404904, -0.7781249993854821856 ) ) ;
#27950=VERTEX_POINT ( 'NONE', #32397 ) ;
#27954=CARTESIAN_POINT ( 'NONE',  ( 15.00000000000000000, 3.464101615137752166, -5.381249998770968546 ) ) ;
#27955=CARTESIAN_POINT ( 'NONE',  ( 20.99999999999999645, -6.646953231504538984, -0.9281249993854503444 ) ) ;
#27958=CARTESIAN_POINT ( 'NONE',  ( 15.24356964375000167, -3.323476615752272600, -10.00312499938545407 ) ) ;
#27966=CARTESIAN_POINT ( 'NONE',  ( 24.97819652690714065, 3.464101615137752166, 164.3132738472399694 ) ) ;
#27970=CARTESIAN_POINT ( 'NONE',  ( 23.87821517812500005, -4.985214923628404016, -2.803124999385481431 ) ) ;
#27974=VERTEX_POINT ( 'NONE', #29169 ) ;
#27976=CARTESIAN_POINT ( 'NONE',  ( 33.84589859903464060, 5.196152422706637353, 162.4081531259335804 ) ) ;
#27980=CARTESIAN_POINT ( 'NONE',  ( 34.05464809739185483, -5.407089921784861808, 163.3968466864631068 ) ) ;
#27983=EDGE_CURVE ( 'NONE', #37220, #2680, #19811, .T. ) ;
#27995=CARTESIAN_POINT ( 'NONE',  ( 26.99999999999999645, 3.464101615137755275, -1.087499999999976374 ) ) ;
#27996=CARTESIAN_POINT ( 'NONE',  ( 24.70858993122118008, 3.604726614523240613, 164.0263046051175024 ) ) ;
#27997=CARTESIAN_POINT ( 'NONE',  ( 24.88995133726802322, 3.464101615137757051, 163.3046267141977239 ) ) ;
#28006=CARTESIAN_POINT ( 'NONE',  ( 31.23317364535864726, -6.928203230275514990, 166.9657099896972170 ) ) ;
#28008=CARTESIAN_POINT ( 'NONE',  ( 26.75643035624999655, -3.323476615752267715, -9.515624999385494220 ) ) ;
#28022=CARTESIAN_POINT ( 'NONE',  ( 23.99999999999999645, 5.196152422706631135, -1.893749998770954956 ) ) ;
#28023=CARTESIAN_POINT ( 'NONE',  ( 33.86345018673919327, -5.407089921784855591, 161.2114445675243530 ) ) ;
#28024=CARTESIAN_POINT ( 'NONE',  ( 18.00000000000000355, -5.196152422706632912, -1.218749998770946030 ) ) ;
#28027=CARTESIAN_POINT ( 'NONE',  ( 24.74614436184151955, 0.000000000000000000, 161.6609054635707423 ) ) ;
#28036=CARTESIAN_POINT ( 'NONE',  ( 34.19028422204287665, 5.407089921784857367, 164.9471746853683669 ) ) ;
#28037=CARTESIAN_POINT ( 'NONE',  ( 18.12178482187500350, -4.985214923628407568, -4.115624999385475213 ) ) ;
#28039=CARTESIAN_POINT ( 'NONE',  ( 37.63846293671737442, -3.604726614523238837, 168.5415738824881373 ) ) ;
#28040=CARTESIAN_POINT ( 'NONE',  ( 28.30668801779110311, 5.196152422706636465, 167.9369659403305093 ) ) ;
#28043=LINE ( 'NONE', #13838, #16058 ) ;
#28047=ORIENTED_EDGE ( 'NONE', *, *, #28617, .F. ) ;
#28050=CARTESIAN_POINT ( 'NONE',  ( 26.75643035624999655, 7.049594010296217766E-16, -4.415624999385469707 ) ) ;
#28053=CARTESIAN_POINT ( 'NONE',  ( 21.00000000000000000, -6.646953231504538984, -1.940624999385496929 ) ) ;
#28065=VECTOR ( 'NONE', #7076, 1000.000000000000000 ) ;
#28079=CARTESIAN_POINT ( 'NONE',  ( 20.99999999999999645, -6.928203230275506996, -2.137499999999987743 ) ) ;
#28081=CARTESIAN_POINT ( 'NONE',  ( 20.99999999999999645, -6.928203230275506996, -1.631249998770951004 ) ) ;
#28085=CARTESIAN_POINT ( 'NONE',  ( 15.00000000000000178, -3.464101615137757051, -8.512500000000017053 ) ) ;
#28091=CARTESIAN_POINT ( 'NONE',  ( 26.75643035624999655, -3.323476615752267715, -6.815624999385487826 ) ) ;
#28098=CARTESIAN_POINT ( 'NONE',  ( 27.68897169117423829, 5.196152422706630247, 160.8764360188296223 ) ) ;
#28101=CARTESIAN_POINT ( 'NONE',  ( 20.99999999999999645, 0.000000000000000000, -8.000000000000000000 ) ) ;
#28133=CARTESIAN_POINT ( 'NONE',  ( 30.76988640036921652, 7.209453229046475009, 161.6703125482654286 ) ) ;
#28136=VERTEX_POINT ( 'NONE', #11408 ) ;
#28137=VERTEX_POINT ( 'NONE', #13705 ) ;
#28139=CARTESIAN_POINT ( 'NONE',  ( 21.00000000000000000, -6.928203230275506996, -4.331249998770957177 ) ) ;
#28140=CARTESIAN_POINT ( 'NONE',  ( 15.24356964374999990, 3.323476615752268604, -1.978124999385461935 ) ) ;
#28148=CARTESIAN_POINT ( 'NONE',  ( 37.03711979530527287, 3.464101615137755275, 164.4628385719782671 ) ) ;
#28153=CARTESIAN_POINT ( 'NONE',  ( 23.87821517812499650, 4.985214923628404904, -3.103124999385475924 ) ) ;
#28159=LINE ( 'NONE', #37240, #21082 ) ;
#28163=CARTESIAN_POINT ( 'NONE',  ( 25.13834520420595098, 0.000000000000000000, 166.1437816049835874 ) ) ;
#28164=CARTESIAN_POINT ( 'NONE',  ( 27.94596069312478903, -5.407089921784865361, 165.2111578762278157 ) ) ;
#28179=CARTESIAN_POINT ( 'NONE',  ( 26.99999999999999645, 3.464101615137755275, -3.337499999999986589 ) ) ;
#28181=CARTESIAN_POINT ( 'NONE',  ( 27.50146640511176344, 5.407089921784862696, 160.1305649159599227 ) ) ;
#28183=CARTESIAN_POINT ( 'NONE',  ( 37.60741370336351252, 7.646167579472015790E-16, 168.1866795212929446 ) ) ;
#28188=VERTEX_POINT ( 'NONE', #24246 ) ;
#28194=CARTESIAN_POINT ( 'NONE',  ( 23.87821517812500005, -4.985214923628404016, -8.653124999385475746 ) ) ;
#28199=CARTESIAN_POINT ( 'NONE',  ( 34.35249135386247588, -5.196152422706629359, 168.1985348098161808 ) ) ;
#28210=CARTESIAN_POINT ( 'NONE',  ( 27.59788244552635206, -5.407089921784859143, 161.2326053007238897 ) ) ;
#28211=CARTESIAN_POINT ( 'NONE',  ( 15.00000000000000000, 3.464101615137752166, -0.4312499987709516591 ) ) ;
#28220=CARTESIAN_POINT ( 'NONE',  ( 26.99999999999999645, 7.347880794884117764E-16, -3.318749998770964549 ) ) ;
#28223=CARTESIAN_POINT ( 'NONE',  ( 31.02481694790609268, -7.209453229046475009, 164.5841820401837765 ) ) ;
#28224=CARTESIAN_POINT ( 'NONE',  ( 15.24356964374999990, 3.323476615752268604, -4.228124999385472371 ) ) ;
#28226=CARTESIAN_POINT ( 'NONE',  ( 25.10732745429168489, -3.604726614523244610, 168.5838953488872676 ) ) ;
#28227=CARTESIAN_POINT ( 'NONE',  ( 31.13512343476753230, 6.928203230275514990, 165.8449909543439560 ) ) ;
#28230=CARTESIAN_POINT ( 'NONE',  ( 34.01258395714663152, 5.196152422706631135, 164.3133754872583836 ) ) ;
#28239=CARTESIAN_POINT ( 'NONE',  ( 18.12178482187500350, -4.985214923628407568, -4.565624999385481608 ) ) ;
#28242=CARTESIAN_POINT ( 'NONE',  ( 15.24356964374999990, 0.000000000000000000, -2.053124999385480542 ) ) ;
#28250=LINE ( 'NONE', #2279, #2470 ) ;
#28258=CARTESIAN_POINT ( 'NONE',  ( 21.00000000000000355, 0.000000000000000000, 50.00000000000001421 ) ) ;
#28271=CARTESIAN_POINT ( 'NONE',  ( 15.00000000000000178, -3.464101615137757051, -9.862500000000006040 ) ) ;
#28276=CARTESIAN_POINT ( 'NONE',  ( 18.12178482187499640, 4.985214923628404904, -7.978124999385494576 ) ) ;
#28282=CARTESIAN_POINT ( 'NONE',  ( 25.14327919817509027, 0.000000000000000000, 168.9948256618500864 ) ) ;
#28305=CARTESIAN_POINT ( 'NONE',  ( 24.66116751255602679, -3.464101615138098111, 160.6896156317068858 ) ) ;
#28316=CARTESIAN_POINT ( 'NONE',  ( 33.95496371662422064, 5.407089921784857367, 162.2574490005206655 ) ) ;
#28317=DIRECTION ( 'NONE',  ( 1.000000000000000000, 0.000000000000000000, 0.000000000000000000 ) ) ;
#28322=CARTESIAN_POINT ( 'NONE',  ( 15.00000000000000000, 0.000000000000000000, -5.793749998770941545 ) ) ;
#28323=CARTESIAN_POINT ( 'NONE',  ( 20.99999999999999645, 6.646953231504538984, -2.053124999385488092 ) ) ;
#28324=CARTESIAN_POINT ( 'NONE',  ( 24.62521576877984231, 3.464101615138150514, 160.2786853199683605 ) ) ;
#28330=VECTOR ( 'NONE', #7709, 1000.000000000000000 ) ;
#28333=CARTESIAN_POINT ( 'NONE',  ( 31.02726820322443047, 6.928203230275506996, 164.6122000166797932 ) ) ;
#28338=CARTESIAN_POINT ( 'NONE',  ( 26.75643035624999655, 7.049594010296217766E-16, -3.178124999385495641 ) ) ;
#28347=CARTESIAN_POINT ( 'NONE',  ( 24.55170959427540822, 3.604726614523240613, 162.2331541485523587 ) ) ;
#28357=LINE ( 'NONE', #7538, #22039 ) ;
#28362=CARTESIAN_POINT ( 'NONE',  ( 24.00000000000000000, -5.196152422706629359, -3.899999999999987033 ) ) ;
#28363=CARTESIAN_POINT ( 'NONE',  ( 37.15151170766156952, 7.347880794884117764E-16, 165.7703441132237003 ) ) ;
#28364=CARTESIAN_POINT ( 'NONE',  ( 28.41103595111929181, 5.957544813848101306, 159.5877724440177303 ) ) ;
#28366=CARTESIAN_POINT ( 'NONE',  ( 37.64663378759995283, 7.646167579472015790E-16, 168.6349671354342092 ) ) ;
#28371=ORIENTED_EDGE ( 'NONE', *, *, #12248, .T. ) ;
#28373=CARTESIAN_POINT ( 'NONE',  ( 36.72335912141303993, 3.464101615138153178, 160.8765376588480649 ) ) ;
#28375=CARTESIAN_POINT ( 'NONE',  ( 21.00000000000000000, 6.646953231504538984, -8.015624999385487115 ) ) ;
#28379=CARTESIAN_POINT ( 'NONE',  ( 23.99999999999999645, 5.196152422706631135, -7.349999999999995204 ) ) ;
#28380=CARTESIAN_POINT ( 'NONE',  ( 30.84342405831255007, 7.209453229046482114, 162.5108518247803318 ) ) ;
#28389=CARTESIAN_POINT ( 'NONE',  ( 36.86550044322413555, 3.604726614523238837, 159.7065721537869365 ) ) ;
#28399=CARTESIAN_POINT ( 'NONE',  ( 33.82423010250274586, -5.407089921784855591, 160.7631569533830600 ) ) ;
#28400=CARTESIAN_POINT ( 'NONE',  ( 15.24356964375000167, -3.323476615752272600, -8.653124999385468641 ) ) ;
#28402=CARTESIAN_POINT ( 'NONE',  ( 25.10079077358561150, 3.604726614523240613, 168.5091807465304043 ) ) ;
#28403=CARTESIAN_POINT ( 'NONE',  ( 37.25609859885165775, -3.464101615137755275, 166.9657777497094457 ) ) ;
#28416=CARTESIAN_POINT ( 'NONE',  ( 23.87821517812499650, 4.985214923628404904, -0.8531249993854739255 ) ) ;
#28427=EDGE_CURVE ( 'NONE', #20921, #12708, #28647, .T. ) ;
#28440=CARTESIAN_POINT ( 'NONE',  ( 25.18413345258805691, 3.604726614523236616, 169.4617919265805881 ) ) ;
#28445=FACE_OUTER_BOUND ( 'NONE', #12763, .T. ) ;
#28449=CARTESIAN_POINT ( 'NONE',  ( 25.28542051998549667, 0.000000000000000000, 167.8248601567890432 ) ) ;
#28454=AXIS2_PLACEMENT_3D ( 'NONE', #30378, #13495, #22410 ) ;
#28457=CARTESIAN_POINT ( 'NONE',  ( 15.24356964374999990, 3.323476615752268604, -7.940624999385462068 ) ) ;
#28460=ORIENTED_EDGE ( 'NONE', *, *, #15354, .T. ) ;
#28463=CARTESIAN_POINT ( 'NONE',  ( 37.52407102436108488, 7.646167579472024665E-16, 167.2340683412427040 ) ) ;
#28466=( BOUNDED_CURVE ( )  B_SPLINE_CURVE ( 2, ( #30933, #18643, #36415, #25050, #33587, #30749, #15789 ),
 .UNSPECIFIED., .F., .F. ) 
 B_SPLINE_CURVE_WITH_KNOTS ( ( 3, 2, 2, 3 ),
 ( 0.5434782608695644113, 0.5507246376811587574, 0.5579710144927531035, 0.5652173913043473386 ),
 .UNSPECIFIED. ) 
 CURVE ( )  GEOMETRIC_REPRESENTATION_ITEM ( )  RATIONAL_B_SPLINE_CURVE ( ( 1.000000000000014433, 0.8660254037844243857, 1.000000000000000000, 0.8660254037844387076, 1.000000000000000000, 0.8660254037844469233, 0.9999999999999917843 ) ) 
 REPRESENTATION_ITEM ( '' )  );
#28470=CARTESIAN_POINT ( 'NONE',  ( 25.18740179294109183, 0.000000000000000000, 169.4991492277590339 ) ) ;
#28473=CARTESIAN_POINT ( 'NONE',  ( 26.99999999999999645, 7.347880794884117764E-16, -1.518749998770940746 ) ) ;
#28481=EDGE_LOOP ( 'NONE', ( #19187, #36707, #10610 ) ) ;
#28498=CARTESIAN_POINT ( 'NONE',  ( 37.10082094864278446, 3.604726614523238837, 162.3962978386346663 ) ) ;
#28499=DIRECTION ( 'NONE',  ( 0.000000000000000000, 0.000000000000000000, 1.000000000000000000 ) ) ;
#28504=CARTESIAN_POINT ( 'NONE',  ( 15.00000000000000000, 0.000000000000000000, -7.143749998770959841 ) ) ;
#28505=CARTESIAN_POINT ( 'NONE',  ( 26.75643035624999655, 3.323476615752271268, -3.478124999385468819 ) ) ;
#28507=CARTESIAN_POINT ( 'NONE',  ( 28.28054129496681313, -5.196152422706638241, 167.6381075309029711 ) ) ;
#28513=CARTESIAN_POINT ( 'NONE',  ( 36.95214294612631534, -3.464101615137751278, 163.4915487413387893 ) ) ;
#28517=CARTESIAN_POINT ( 'NONE',  ( 18.12178482187500350, -4.985214923628407568, -5.578124999385480898 ) ) ;
#28519=CARTESIAN_POINT ( 'NONE',  ( 20.99999999999999645, 6.928203230275506996, -0.5624999999999866773 ) ) ;
#28527=CARTESIAN_POINT ( 'NONE',  ( 30.82381401619432637, -7.209453229046482114, 162.2867080177096852 ) ) ;
#28540=CARTESIAN_POINT ( 'NONE',  ( 15.00000000000000178, -3.464101615137757051, -5.362499999999983835 ) ) ;
#28543=CARTESIAN_POINT ( 'NONE',  ( 24.47653776615555898, 0.000000000000000000, 161.3739362214482469 ) ) ;
#28545=CARTESIAN_POINT ( 'NONE',  ( 24.65463083184936366, 3.464101615137757051, 160.6149010293500226 ) ) ;
#28555=CARTESIAN_POINT ( 'NONE',  ( 26.75643035624999655, 7.049594010296217766E-16, -9.028124999385489957 ) ) ;
#28558=CARTESIAN_POINT ( 'NONE',  ( 24.98477879236699195, 0.000000000000000000, 49.65137702900941008 ) ) ;
#28559=CARTESIAN_POINT ( 'NONE',  ( 24.59092967851185207, 3.604726614523240613, 162.6814417626936518 ) ) ;
#28568=ORIENTED_EDGE ( 'NONE', *, *, #20383, .T. ) ;
#28571=CARTESIAN_POINT ( 'NONE',  ( 36.82628035898769525, 3.604726614523238837, 159.2582845396456719 ) ) ;
#28572=CARTESIAN_POINT ( 'NONE',  ( 15.00000000000000178, -3.464101615137757051, -0.8062499987709534910 ) ) ;
#28580=DIRECTION ( 'NONE',  ( 1.000000000000000000, 0.000000000000000000, 0.000000000000000000 ) ) ;
#28582=CARTESIAN_POINT ( 'NONE',  ( 37.02238078016990386, 3.604726614523238837, 161.4997226103520802 ) ) ;
#28583=CARTESIAN_POINT ( 'NONE',  ( 15.24356964375000167, -3.323476615752272600, -6.853124999385484806 ) ) ;
#28585=CARTESIAN_POINT ( 'NONE',  ( 28.14206111430700474, -5.407089921784865361, 167.4525959469342524 ) ) ;
#28586=CARTESIAN_POINT ( 'NONE',  ( 25.16776026727616511, 0.000000000000000000, 166.4799973143651926 ) ) ;
#28590=EDGE_CURVE ( 'NONE', #952, #2107, #32762, .T. ) ;
#28600=CARTESIAN_POINT ( 'NONE',  ( 26.75643035624999655, -3.323476615752267715, -2.765624999385494220 ) ) ;
#28607=EDGE_CURVE ( 'NONE', #34104, #32257, #18944, .T. ) ;
#28616=FACE_OUTER_BOUND ( 'NONE', #22904, .T. ) ;
#28617=EDGE_CURVE ( 'NONE', #26185, #34425, #6860, .T. ) ;
#28618=CARTESIAN_POINT ( 'NONE',  ( 34.34268633269625326, -5.196152422706635576, 168.0864629050564929 ) ) ;
#28623=CARTESIAN_POINT ( 'NONE',  ( 25.19067013329413385, -3.604726614523240613, 169.5365065289374513 ) ) ;
#28626=EDGE_CURVE ( 'NONE', #1229, #14950, #13166, .T. ) ;
#28634=CARTESIAN_POINT ( 'NONE',  ( 26.99999999999999645, -3.464101615137751278, -9.262500000000022382 ) ) ;
#28640=CARTESIAN_POINT ( 'NONE',  ( 18.12178482187499640, 4.985214923628404904, -9.328124999385483562 ) ) ;
#28642=EDGE_CURVE ( 'NONE', #16220, #20921, #18272, .T. ) ;
#28646=CARTESIAN_POINT ( 'NONE',  ( 37.36719068741531657, 7.646167579472024665E-16, 165.4409178846775603 ) ) ;
#28647=( BOUNDED_CURVE ( )  B_SPLINE_CURVE ( 2, ( #15145, #24431, #35981, #10017, #21598, #33147, #7191 ),
 .UNSPECIFIED., .F., .F. ) 
 B_SPLINE_CURVE_WITH_KNOTS ( ( 3, 2, 2, 3 ),
 ( 0.5869565217391301548, 0.5942028985507243899, 0.6014492753623187360, 0.6086956521739130821 ),
 .UNSPECIFIED. ) 
 CURVE ( )  GEOMETRIC_REPRESENTATION_ITEM ( )  RATIONAL_B_SPLINE_CURVE ( ( 1.000000000000006217, 0.8660254037844326014, 1.000000000000000000, 0.8660254037844387076, 1.000000000000000000, 0.8660254037844387076, 1.000000000000000000 ) ) 
 REPRESENTATION_ITEM ( '' )  );
#28651=EDGE_CURVE ( 'NONE', #24633, #2680, #2970, .T. ) ;
#28654=CARTESIAN_POINT ( 'NONE',  ( 25.37366570962461054, 0.000000000000000000, 168.8335072898312887 ) ) ;
#28666=CARTESIAN_POINT ( 'NONE',  ( 33.88511868327108090, 5.196152422706637353, 162.8564407400748451 ) ) ;
#28667=DIRECTION ( 'NONE',  ( 0.9961946980917462113, 0.000000000000000000, -0.08715574274765118534 ) ) ;
#28680=CARTESIAN_POINT ( 'NONE',  ( 27.75476278247212747, -5.407089921784859143, 163.0257557572890335 ) ) ;
#28681=CARTESIAN_POINT ( 'NONE',  ( 21.00000000000000000, -6.646953231504538984, -2.390624999385460470 ) ) ;
#28687=CARTESIAN_POINT ( 'NONE',  ( 21.00000000000000000, -6.928203230275506996, -6.131249998770972098 ) ) ;
#28688=CARTESIAN_POINT ( 'NONE',  ( 26.75643035624999655, 3.323476615752271268, -2.128124999385481608 ) ) ;
#28690=CARTESIAN_POINT ( 'NONE',  ( 27.61053152270135058, 5.196152422706630247, 159.9798607905470362 ) ) ;
#28699=CARTESIAN_POINT ( 'NONE',  ( 21.00000000000000355, 0.000000000000000000, 50.00000000000001421 ) ) ;
#28701=CARTESIAN_POINT ( 'NONE',  ( 34.03873067997093216, -5.196152422706629359, 164.6122338966858933 ) ) ;
#28706=CARTESIAN_POINT ( 'NONE',  ( 23.87821517812499650, 4.985214923628404904, -4.453124999385494220 ) ) ;
#28712=CARTESIAN_POINT ( 'NONE',  ( 24.94551312337715032, -3.464101615137971546, 163.9397008354555965 ) ) ;
#28716=CARTESIAN_POINT ( 'NONE',  ( 30.74537384772143866, -7.209453229046482114, 161.3901327894271276 ) ) ;
#28719=LINE ( 'NONE', #6160, #33407 ) ;
#28723=CARTESIAN_POINT ( 'NONE',  ( 25.09585677961620576, 3.464101615137598067, 165.6581366896638770 ) ) ;
#28727=CARTESIAN_POINT ( 'NONE',  ( 21.00000000000000000, -6.928203230275506996, -3.487500000000006928 ) ) ;
#28729=CARTESIAN_POINT ( 'NONE',  ( 24.44058602227215360, -3.604726614523244610, 160.9630059084853997 ) ) ;
#28731=CARTESIAN_POINT ( 'NONE',  ( 30.64487238181199302, -6.928203230275514990, 160.2413957775779068 ) ) ;
#28733=CARTESIAN_POINT ( 'NONE',  ( 19.80074372294634344, 5.630122097104456991, -7.999999999999998224 ) ) ;
#28737=CARTESIAN_POINT ( 'NONE',  ( 15.00000000000000355, 7.347880794884112834E-16, -8.000000000000000000 ) ) ;
#28739=CARTESIAN_POINT ( 'NONE',  ( 23.99999999999999645, 5.196152422706631135, -5.043749998770941545 ) ) ;
#28741=DIRECTION ( 'NONE',  ( 0.08715574274765150453, 0.000000000000000000, 0.9961946980917461003 ) ) ;
#28745=CARTESIAN_POINT ( 'NONE',  ( 24.59419801886489054, 0.000000000000000000, 162.7187990638720976 ) ) ;
#28747=CARTESIAN_POINT ( 'NONE',  ( 28.11058759660888740, 5.196152422706636465, 165.6955278696240725 ) ) ;
#28749=AXIS2_PLACEMENT_3D ( 'NONE', #21946, #1462, #15505 ) ;
#28759=CARTESIAN_POINT ( 'NONE',  ( 29.49486222041940664, 6.148715791637009431, 159.5363414366720178 ) ) ;
#28760=CARTESIAN_POINT ( 'NONE',  ( 24.00000000000000000, -5.196152422706629359, -1.593749998770960241 ) ) ;
#28769=CARTESIAN_POINT ( 'NONE',  ( 27.66324925258708589, 5.407089921784856479, 161.9797513242927209 ) ) ;
#28770=CARTESIAN_POINT ( 'NONE',  ( 26.75643035624999655, -3.323476615752267715, -6.703124999385464911 ) ) ;
#28772=CARTESIAN_POINT ( 'NONE',  ( 25.06483902970220967, 0.000000000000000000, 168.0982504335675287 ) ) ;
#28773=CARTESIAN_POINT ( 'NONE',  ( 25.20371201115956694, 3.464101615137757051, 166.8909276273280682 ) ) ;
#28774=CARTESIAN_POINT ( 'NONE',  ( 15.00000000000000000, 3.464101615137752610, -0.03749999999999697325 ) ) ;
#28781=ADVANCED_FACE ( 'NONE', ( #28935 ), #12061, .T. ) ;
#28783=ORIENTED_EDGE ( 'NONE', *, *, #1506, .T. ) ;
#28788=CARTESIAN_POINT ( 'NONE',  ( 21.00000000000000000, 6.646953231504538984, -1.715624999385482852 ) ) ;
#28809=CARTESIAN_POINT ( 'NONE',  ( 31.35818766391586365, 7.209453229046475009, 168.3946267603846820 ) ) ;
#28811=CARTESIAN_POINT ( 'NONE',  ( 15.24356964374999990, 0.000000000000000000, -1.040624999385481031 ) ) ;
#28826=CARTESIAN_POINT ( 'NONE',  ( 26.75643035624999655, 3.323476615752271712, -0.3281249993854667424 ) ) ;
#28829=EDGE_LOOP ( 'NONE', ( #31045, #26169, #9894, #25984 ) ) ;
#28832=CARTESIAN_POINT ( 'NONE',  ( 25.02235060511272735, 3.604726614523240613, 167.6126055182478183 ) ) ;
#28840=CARTESIAN_POINT ( 'NONE',  ( 37.30839204460733782, 7.347880794884117764E-16, 167.5634945697888440 ) ) ;
#28847=( BOUNDED_CURVE ( )  B_SPLINE_CURVE ( 2, ( #35206, #1091, #35392, #18171, #21208, #9441, #9255 ),
 .UNSPECIFIED., .F., .F. ) 
 B_SPLINE_CURVE_WITH_KNOTS ( ( 3, 2, 2, 3 ),
 ( 0.04347826086956516067, 0.05072463768115926391, 0.05797101449275336715, 0.06521739130434746345 ),
 .UNSPECIFIED. ) 
 CURVE ( )  GEOMETRIC_REPRESENTATION_ITEM ( )  RATIONAL_B_SPLINE_CURVE ( ( 1.000000000000000888, 0.8660254037844375974, 1.000000000000000000, 0.8660254037844387076, 1.000000000000000000, 0.8660254037844453689, 0.9999999999999933387 ) ) 
 REPRESENTATION_ITEM ( '' )  );
#28855=FACE_OUTER_BOUND ( 'NONE', #22920, .T. ) ;
#28867=ORIENTED_EDGE ( 'NONE', *, *, #10856, .T. ) ;
#28870=CARTESIAN_POINT ( 'NONE',  ( 24.40300010821222898, 0.000000000000000000, 160.5333969449332869 ) ) ;
#28871=CARTESIAN_POINT ( 'NONE',  ( 26.75643035624999655, 3.323476615752271712, -3.140624999385464022 ) ) ;
#28874=VERTEX_POINT ( 'NONE', #20235 ) ;
#28876=( BOUNDED_CURVE ( )  B_SPLINE_CURVE ( 2, ( #29362, #23500, #15347, #32019, #26901, #6050, #12115 ),
 .UNSPECIFIED., .F., .F. ) 
 B_SPLINE_CURVE_WITH_KNOTS ( ( 3, 2, 2, 3 ),
 ( 0.6521739130434789367, 0.6594202898550732828, 0.6666666666666675178, 0.6739130434782618639 ),
 .UNSPECIFIED. ) 
 CURVE ( )  GEOMETRIC_REPRESENTATION_ITEM ( )  RATIONAL_B_SPLINE_CURVE ( ( 0.9999999999999876765, 0.8660254037844510311, 1.000000000000000000, 0.8660254037844387076, 1.000000000000000000, 0.8660254037844202779, 1.000000000000018430 ) ) 
 REPRESENTATION_ITEM ( '' )  );
#28878=CARTESIAN_POINT ( 'NONE',  ( 26.99999999999999645, 3.464101615137755275, -6.881249998770976539 ) ) ;
#28879=CARTESIAN_POINT ( 'NONE',  ( 15.24356964374999990, 0.000000000000000000, -3.290624999385455496 ) ) ;
#28888=CARTESIAN_POINT ( 'NONE',  ( 27.80663194388356629, 5.196152422706630247, 162.2212988612534730 ) ) ;
#28892=CARTESIAN_POINT ( 'NONE',  ( 15.24356964374999990, 3.323476615752268604, -5.240624999385486760 ) ) ;
#28897=CARTESIAN_POINT ( 'NONE',  ( 14.99999999999968203, -3.464101615137573198, -6.712500000000007461 ) ) ;
#28900=CARTESIAN_POINT ( 'NONE',  ( 23.35209618661503583, -3.999999999999909850, 50.00000000000000000 ) ) ;
#28901=CARTESIAN_POINT ( 'NONE',  ( 34.02850137456756130, 5.407089921784862696, 163.0979882770355971 ) ) ;
#28905=CARTESIAN_POINT ( 'NONE',  ( 36.56321044411491528, 7.347880794884117764E-16, 159.0460299011043901 ) ) ;
#28914=CARTESIAN_POINT ( 'NONE',  ( 24.00000000000000000, -5.196152422706629359, -5.250000000000004441 ) ) ;
#28916=CYLINDRICAL_SURFACE ( 'NONE', #20325, 6.000000000000001776 ) ;
#28918=CARTESIAN_POINT ( 'NONE',  ( 24.93897644267032732, 3.464101615137538115, 163.8649862330987332 ) ) ;
#28920=CARTESIAN_POINT ( 'NONE',  ( 30.62526233969377998, 6.928203230275514990, 160.0172519705072318 ) ) ;
#28922=EDGE_CURVE ( 'NONE', #13615, #17372, #14727, .T. ) ;
#28926=FACE_OUTER_BOUND ( 'NONE', #19819, .T. ) ;
#28928=CARTESIAN_POINT ( 'NONE',  ( 15.24356964375000167, -3.323476615752272600, -5.503124999385465621 ) ) ;
#28935=FACE_OUTER_BOUND ( 'NONE', #7777, .T. ) ;
#28936=CARTESIAN_POINT ( 'NONE',  ( 31.39985900347063819, -6.928203230275506996, 168.8709323510220202 ) ) ;
#28948=CARTESIAN_POINT ( 'NONE',  ( 33.70656984979341786, -5.407089921784855591, 159.4182941109592093 ) ) ;
#28949=CARTESIAN_POINT ( 'NONE',  ( 15.00000000000000000, 3.464101615137752166, -1.331249998770975163 ) ) ;
#28958=CARTESIAN_POINT ( 'NONE',  ( 24.52392870127459901, -3.604726614523240613, 161.9156170885355834 ) ) ;
#28959=CARTESIAN_POINT ( 'NONE',  ( 15.24356964375000167, -3.323476615752272600, -8.203124999385472904 ) ) ;
#28961=CARTESIAN_POINT ( 'NONE',  ( 37.60251119283397259, 7.646167579472024665E-16, 168.1306435695252901 ) ) ;
#28962=CARTESIAN_POINT ( 'NONE',  ( 37.14170668649535401, 7.347880794884125653E-16, 165.6582722084640125 ) ) ;
#28967=ORIENTED_EDGE ( 'NONE', *, *, #30342, .F. ) ;
#28972=CARTESIAN_POINT ( 'NONE',  ( 18.12178482187500350, -4.985214923628407568, -4.228124999385491023 ) ) ;
#28994=CARTESIAN_POINT ( 'NONE',  ( 25.15145004905768644, -3.604726614523240613, 169.0882189147961583 ) ) ;
#28996=CARTESIAN_POINT ( 'NONE',  ( 26.75643035624999655, 3.323476615752271712, -0.3281249993854667424 ) ) ;
#29003=VERTEX_POINT ( 'NONE', #35558 ) ;
#29008=CARTESIAN_POINT ( 'NONE',  ( 26.75643035624999655, 7.049594010296217766E-16, -9.928124999385474325 ) ) ;
#29010=ORIENTED_EDGE ( 'NONE', *, *, #22684, .T. ) ;
#29013=CARTESIAN_POINT ( 'NONE',  ( 31.29445502703164905, -7.209453229046482114, 167.6661593874051164 ) ) ;
#29020=CARTESIAN_POINT ( 'NONE',  ( 37.52570519453759346, -3.604726614523235284, 167.2527469918319412 ) ) ;
#29022=CARTESIAN_POINT ( 'NONE',  ( 25.16776026727616511, 0.000000000000000000, 166.4799973143651926 ) ) ;
#29023=CARTESIAN_POINT ( 'NONE',  ( 36.91619120224290640, 7.347880794884117764E-16, 163.0806184283759706 ) ) ;
#29031=ORIENTED_EDGE ( 'NONE', *, *, #6641, .F. ) ;
#29036=FACE_OUTER_BOUND ( 'NONE', #32240, .T. ) ;
#29050=CARTESIAN_POINT ( 'NONE',  ( 21.00000000000000000, -6.646953231504538984, -1.490624999385501193 ) ) ;
#29054=ORIENTED_EDGE ( 'NONE', *, *, #21957, .F. ) ;
#29056=EDGE_LOOP ( 'NONE', ( #23554, #7951, #33852, #2692 ) ) ;
#29057=CARTESIAN_POINT ( 'NONE',  ( 26.75643035624999655, -3.323476615752267271, -4.903124999385481964 ) ) ;
#29065=CARTESIAN_POINT ( 'NONE',  ( 30.87038786627866216, 6.928203230275506996, 162.8190495601146495 ) ) ;
#29070=CARTESIAN_POINT ( 'NONE',  ( 26.75643035624999655, -3.323476615752267271, -3.665624999385486138 ) ) ;
#29071=CARTESIAN_POINT ( 'NONE',  ( 26.99999999999999645, 7.347880794884117764E-16, -1.574999999999993072 ) ) ;
#29074=EDGE_CURVE ( 'NONE', #13953, #17429, #9602, .T. ) ;
#29080=ADVANCED_FACE ( 'NONE', ( #681 ), #30254, .T. ) ;
#29081=CARTESIAN_POINT ( 'NONE',  ( 37.09265009776020605, 7.646167579472024665E-16, 162.3029045856885659 ) ) ;
#29094=CARTESIAN_POINT ( 'NONE',  ( 18.00000000000000355, -5.196152422706632912, -5.775000000000002132 ) ) ;
#29097=CARTESIAN_POINT ( 'NONE',  ( 36.87697111800645899, 7.347880794884117764E-16, 162.6323308142347059 ) ) ;
#29099=CARTESIAN_POINT ( 'NONE',  ( 37.37209319794485651, 7.646167579472015790E-16, 165.4969538364452148 ) ) ;
#29107=CARTESIAN_POINT ( 'NONE',  ( 26.75643035624999655, 3.323476615752271712, -7.528124999385462424 ) ) ;
#29109=CARTESIAN_POINT ( 'NONE',  ( 15.00000000000000000, 0.000000000000000000, -5.343749998770963572 ) ) ;
#29114=CARTESIAN_POINT ( 'NONE',  ( 24.35887751344623098, 0.000000000000000000, 160.0290733790243962 ) ) ;
#29126=CARTESIAN_POINT ( 'NONE',  ( 23.43386378601147513, 5.229754410370055062, -8.000000000000001776 ) ) ;
#29127=CARTESIAN_POINT ( 'NONE',  ( 28.29894145125277660, -5.407089921784865361, 169.2457464034993961 ) ) ;
#29128=CARTESIAN_POINT ( 'NONE',  ( 15.00000000000000000, 0.000000000000000000, -2.643749998770955401 ) ) ;
#29140=CARTESIAN_POINT ( 'NONE',  ( 27.70246933682352974, 5.407089921784856479, 162.4280389384339855 ) ) ;
#29141=CARTESIAN_POINT ( 'NONE',  ( 26.75643035624999655, 7.049594010296217766E-16, -8.465624999385468641 ) ) ;
#29142=CARTESIAN_POINT ( 'NONE',  ( 28.02440086159767674, -5.407089921784865361, 166.1077331045103733 ) ) ;
#29143=CARTESIAN_POINT ( 'NONE',  ( 25.05010001456683710, 0.000000000000000000, 165.1351344719413419 ) ) ;
#29149=VERTEX_POINT ( 'NONE', #27034 ) ;
#29154=CARTESIAN_POINT ( 'NONE',  ( 21.00000000000000000, 6.646953231504538984, -5.315624999385480720 ) ) ;
#29167=ADVANCED_FACE ( 'NONE', ( #6957 ), #18525, .F. ) ;
#29169=CARTESIAN_POINT ( 'NONE',  ( 26.99999999999999645, 7.347880794884117764E-16, -2.024999999999999023 ) ) ;
#29172=CARTESIAN_POINT ( 'NONE',  ( 25.22417062191275861, 0.000000000000000000, 169.9194188660164571 ) ) ;
#29173=CARTESIAN_POINT ( 'NONE',  ( 18.00000000000000355, -5.196152422706632912, -0.3749999999999864553 ) ) ;
#29174=( BOUNDED_CURVE ( )  B_SPLINE_CURVE ( 2, ( #14526, #26082, #5249, #8840, #23250, #34796, #20412 ),
 .UNSPECIFIED., .F., .F. ) 
 B_SPLINE_CURVE_WITH_KNOTS ( ( 3, 2, 2, 3 ),
 ( 0.04347826086956579211, 0.05072463768116009658, 0.05797101449275439411, 0.06521739130434869858 ),
 .UNSPECIFIED. ) 
 CURVE ( )  GEOMETRIC_REPRESENTATION_ITEM ( )  RATIONAL_B_SPLINE_CURVE ( ( 0.9999999999999893419, 0.8660254037844493658, 1.000000000000000000, 0.8660254037844387076, 1.000000000000000000, 0.8660254037844226094, 1.000000000000016209 ) ) 
 REPRESENTATION_ITEM ( '' )  );
#29182=CYLINDRICAL_SURFACE ( 'NONE', #15516, 5.999999999999994671 ) ;
#29184=CARTESIAN_POINT ( 'NONE',  ( 26.75643035624999655, 3.323476615752271712, -0.7781249993854945091 ) ) ;
#29197=CARTESIAN_POINT ( 'NONE',  ( 18.12178482187500350, -4.985214923628407568, -9.178124999385472549 ) ) ;
#29199=( BOUNDED_CURVE ( )  B_SPLINE_CURVE ( 2, ( #22520, #33884, #19500, #28006, #16649, #13422, #16276 ),
 .UNSPECIFIED., .F., .F. ) 
 B_SPLINE_CURVE_WITH_KNOTS ( ( 3, 2, 2, 3 ),
 ( 0.2391304347826079535, 0.2463768115942022718, 0.2536231884057966179, 0.2608695652173909085 ),
 .UNSPECIFIED. ) 
 CURVE ( )  GEOMETRIC_REPRESENTATION_ITEM ( )  RATIONAL_B_SPLINE_CURVE ( ( 1.000000000000013989, 0.8660254037844249408, 1.000000000000000000, 0.8660254037844387076, 1.000000000000000000, 0.8660254037844459241, 0.9999999999999927836 ) ) 
 REPRESENTATION_ITEM ( '' )  );
#29205=CARTESIAN_POINT ( 'NONE',  ( 28.06362094583411704, -5.407089921784865361, 166.5560207186516664 ) ) ;
#29211=DIRECTION ( 'NONE',  ( 0.08715574274765150453, 0.000000000000000000, 0.9961946980917461003 ) ) ;
#29212=CARTESIAN_POINT ( 'NONE',  ( 37.64336544724691436, -3.604726614523235284, 168.5976098342557918 ) ) ;
#29213=ORIENTED_EDGE ( 'NONE', *, *, #36432, .F. ) ;
#29230=CARTESIAN_POINT ( 'NONE',  ( 28.23805287048444512, 5.196152422706630247, 167.1524626168076111 ) ) ;
#29231=CARTESIAN_POINT ( 'NONE',  ( 25.33444562538816669, 0.000000000000000000, 168.3852196756899957 ) ) ;
#29235=ORIENTED_EDGE ( 'NONE', *, *, #10261, .F. ) ;
#29240=CARTESIAN_POINT ( 'NONE',  ( 28.41594069642870579, 5.957546110389989380, 159.6438081731886314 ) ) ;
#29241=CARTESIAN_POINT ( 'NONE',  ( 18.12178482187500350, -4.985214923628407568, -2.428124999385494753 ) ) ;
#29245=ORIENTED_EDGE ( 'NONE', *, *, #36523, .F. ) ;
#29247=CARTESIAN_POINT ( 'NONE',  ( 26.75643035624999655, 7.049594010296217766E-16, -6.215624999385465976 ) ) ;
#29254=CARTESIAN_POINT ( 'NONE',  ( 30.73311757145110690, -6.928203230275506996, 161.2500429106201523 ) ) ;
#29260=CARTESIAN_POINT ( 'NONE',  ( 26.75643035624999655, 7.049594010296217766E-16, -4.528124999385485516 ) ) ;
#29265=CARTESIAN_POINT ( 'NONE',  ( 27.85892538953216757, -5.196152422706632912, 162.8190156801084925 ) ) ;
#29268=EDGE_CURVE ( 'NONE', #17429, #8055, #10731, .T. ) ;
#29270=CARTESIAN_POINT ( 'NONE',  ( 28.41103595111929536, 5.957544813848101306, 159.5877724440177303 ) ) ;
#29274=CARTESIAN_POINT ( 'NONE',  ( 24.00000000000000000, -5.196152422706629359, -1.143749998770954290 ) ) ;
#29276=CARTESIAN_POINT ( 'NONE',  ( 37.34107544803033107, 3.464101615137920032, 167.9370675803488950 ) ) ;
#29279=CARTESIAN_POINT ( 'NONE',  ( 15.00000000000000000, 0.000000000000000000, -7.593749998770965348 ) ) ;
#29284=CARTESIAN_POINT ( 'NONE',  ( 15.00000000000000000, 0.000000000000000000, -6.299999999999999822 ) ) ;
#29285=FACE_OUTER_BOUND ( 'NONE', #21834, .T. ) ;
#29286=DIRECTION ( 'NONE',  ( 0.000000000000000000, 0.000000000000000000, 1.000000000000000000 ) ) ;
#29288=CARTESIAN_POINT ( 'NONE',  ( 34.30794447475221176, 5.407089921784857367, 166.2920375277922460 ) ) ;
#29290=CARTESIAN_POINT ( 'NONE',  ( 36.60243052835136268, 7.347880794884117764E-16, 159.4943175152456831 ) ) ;
#29295=CARTESIAN_POINT ( 'NONE',  ( 27.60072650153512441, 5.196152422706636465, 159.8677888857873768 ) ) ;
#29296=CYLINDRICAL_SURFACE ( 'NONE', #4572, 3.999999999999996447 ) ;
#29298=CARTESIAN_POINT ( 'NONE',  ( 26.75643035624999655, 3.323476615752271712, -6.178124999385475213 ) ) ;
#29305=CARTESIAN_POINT ( 'NONE',  ( 31.41946904558886544, 6.928203230275506996, 169.0950761580926383 ) ) ;
#29307=EDGE_CURVE ( 'NONE', #6128, #17802, #18497, .T. ) ;
#29320=CARTESIAN_POINT ( 'NONE',  ( 24.98313052087628350, 3.604726614523240613, 167.1643179041065252 ) ) ;
#29321=CARTESIAN_POINT ( 'NONE',  ( 15.00000000000000000, 0.000000000000000000, -3.093749998770961795 ) ) ;
#29322=VERTEX_POINT ( 'NONE', #31501 ) ;
#29334=CARTESIAN_POINT ( 'NONE',  ( 24.00000000000000000, -5.196152422706629359, -0.2999999999999947153 ) ) ;
#29336=CARTESIAN_POINT ( 'NONE',  ( 31.13757469008587719, -7.209453229046482114, 165.8730089308399442 ) ) ;
#29337=CARTESIAN_POINT ( 'NONE',  ( 36.90311784072365242, -3.464101615137755275, 162.9311892224378369 ) ) ;
#29343=EDGE_LOOP ( 'NONE', ( #1800, #13283, #3382, #15681 ) ) ;
#29349=CARTESIAN_POINT ( 'NONE',  ( 26.75643035624999655, 3.323476615752271712, -4.490624999385484095 ) ) ;
#29358=CARTESIAN_POINT ( 'NONE',  ( 24.90302469878729141, 0.000000000000000000, 163.4540559201358576 ) ) ;
#29362=CARTESIAN_POINT ( 'NONE',  ( 15.00000000000000000, 0.000000000000000000, -7.143749998770959841 ) ) ;
#29375=CARTESIAN_POINT ( 'NONE',  ( 31.16208724273364439, 7.209453229046475009, 166.1531886896782737 ) ) ;
#29376=CARTESIAN_POINT ( 'NONE',  ( 23.87821517812499650, 4.985214923628404904, -1.640624999385470462 ) ) ;
#29379=CARTESIAN_POINT ( 'NONE',  ( 23.99999999999999645, 5.196152422706631135, -3.750000000000003553 ) ) ;
#29380=CARTESIAN_POINT ( 'NONE',  ( 15.02283181144952628, 7.347880794884122694E-16, 50.52293445648592751 ) ) ;
#29381=EDGE_CURVE ( 'NONE', #36867, #22329, #22370, .T. ) ;
#29382=CARTESIAN_POINT ( 'NONE',  ( 25.14161354455920261, -3.464101615137879620, 166.1811389061619764 ) ) ;
#29390=CARTESIAN_POINT ( 'NONE',  ( 23.87821517812500005, -4.985214923628404016, -8.653124999385475746 ) ) ;
#29399=CARTESIAN_POINT ( 'NONE',  ( 30.88264414254898682, 7.209453229046482114, 162.9591394389216532 ) ) ;
#29405=CARTESIAN_POINT ( 'NONE',  ( 17.00000000000000000, 4.898587196589404940E-16, -8.000000000000000000 ) ) ;
#29407=( BOUNDED_CURVE ( )  B_SPLINE_CURVE ( 2, ( #8969, #3085, #26022, #23192, #26205, #34740, #242 ),
 .UNSPECIFIED., .F., .F. ) 
 B_SPLINE_CURVE_WITH_KNOTS ( ( 3, 2, 2, 3 ),
 ( 0.7173913043478246099, 0.7246376811594190670, 0.7318840579710134131, 0.7391304347826077592 ),
 .UNSPECIFIED. ) 
 CURVE ( )  GEOMETRIC_REPRESENTATION_ITEM ( )  RATIONAL_B_SPLINE_CURVE ( ( 1.000000000000026645, 0.8660254037844120623, 1.000000000000000000, 0.8660254037844387076, 1.000000000000000000, 0.8660254037844551389, 0.9999999999999835687 ) ) 
 REPRESENTATION_ITEM ( '' )  );
#29409=CARTESIAN_POINT ( 'NONE',  ( 37.32960477335537774, -3.604726614523235284, 165.0113089211254760 ) ) ;
#29425=CARTESIAN_POINT ( 'NONE',  ( 33.80667851479820030, 5.196152422706637353, 161.9598655117922874 ) ) ;
#29435=CARTESIAN_POINT ( 'NONE',  ( 36.85896376251805151, -3.604726614523235284, 159.6318575514300449 ) ) ;
#29436=CARTESIAN_POINT ( 'NONE',  ( 26.75643035624999655, 7.049594010296217766E-16, -1.828124999385477567 ) ) ;
#29439=ORIENTED_EDGE ( 'NONE', *, *, #21502, .T. ) ;
#29441=CARTESIAN_POINT ( 'NONE',  ( 18.12178482187499640, 4.985214923628404904, -4.265624999385458693 ) ) ;
#29449=CARTESIAN_POINT ( 'NONE',  ( 27.85892538953216757, -5.196152422706632912, 162.8190156801084925 ) ) ;
#29453=CARTESIAN_POINT ( 'NONE',  ( 18.12178482187500350, -4.985214923628407568, -7.828124999385482674 ) ) ;
#29457=ORIENTED_EDGE ( 'NONE', *, *, #35891, .F. ) ;
#29458=CARTESIAN_POINT ( 'NONE',  ( 24.86707295490436209, -3.464101615138032830, 163.0431256071729820 ) ) ;
#29461=CARTESIAN_POINT ( 'NONE',  ( 20.99999999999999645, 0.000000000000000000, -8.000000000000000000 ) ) ;
#29462=CARTESIAN_POINT ( 'NONE',  ( 24.47980610650859390, -3.604726614523244610, 161.4112935226266359 ) ) ;
#29471=CARTESIAN_POINT ( 'NONE',  ( 34.05180404138307182, 5.196152422706631135, 164.7616631013996766 ) ) ;
#29475=CARTESIAN_POINT ( 'NONE',  ( 24.00000000000000000, -5.196152422706629359, -6.599999999999994316 ) ) ;
#29479=CARTESIAN_POINT ( 'NONE',  ( 28.10774354060011504, -5.407089921784859143, 167.0603442845606139 ) ) ;
#29483=ORIENTED_EDGE ( 'NONE', *, *, #1751, .F. ) ;
#29485=CARTESIAN_POINT ( 'NONE',  ( 24.61541074761229098, 3.464101615137389345, 160.1666134152088148 ) ) ;
#29486=B_SPLINE_CURVE_WITH_KNOTS ( 'NONE', 1,
 ( #31296, #32031 ),
 .UNSPECIFIED., .F., .F.,
 ( 2, 2 ),
 ( 0.000000000000000000, 1.000000000000000000 ),
 .UNSPECIFIED. ) ;
#29490=CARTESIAN_POINT ( 'NONE',  ( 26.75643035624999655, -3.323476615752267715, -5.803124999385441463 ) ) ;
#29493=CARTESIAN_POINT ( 'NONE',  ( 25.05336835492019176, -3.464101615137944457, 165.1724917731197024 ) ) ;
#29497=CARTESIAN_POINT ( 'NONE',  ( 27.46224632087531958, 5.407089921784862696, 159.6822773018186297 ) ) ;
#29511=CARTESIAN_POINT ( 'NONE',  ( 31.19640481644053409, 7.209453229046482114, 166.5454403520519122 ) ) ;
#29512=CARTESIAN_POINT ( 'NONE',  ( 26.99999999999999645, 3.464101615137755275, -2.381249998770954779 ) ) ;
#29516=CARTESIAN_POINT ( 'NONE',  ( 26.97716818855048260, 0.000000000000000000, 49.47706554351410801 ) ) ;
#29521=CARTESIAN_POINT ( 'NONE',  ( 36.95541128647934670, 7.347880794884117764E-16, 163.5289060425172636 ) ) ;
#29524=CARTESIAN_POINT ( 'NONE',  ( 18.12178482187499640, 4.985214923628404904, -10.11562499938548143 ) ) ;
#29526=CARTESIAN_POINT ( 'NONE',  ( 26.99999999999999645, 7.347880794884117764E-16, -0.6750000000000089262 ) ) ;
#29527=CARTESIAN_POINT ( 'NONE',  ( 37.20704201011650269, -3.604726614523238837, 163.6104101269339424 ) ) ;
#29528=CARTESIAN_POINT ( 'NONE',  ( 28.07136751237244354, 5.196152422706636465, 165.2472402554827795 ) ) ;
#29529=CARTESIAN_POINT ( 'NONE',  ( 26.99999999999983658, -3.464101615137843648, -6.956249998770940302 ) ) ;
#29540=CARTESIAN_POINT ( 'NONE',  ( 23.87821517812499650, 4.985214923628404904, -4.453124999385494220 ) ) ;
#29554=DIRECTION ( 'NONE',  ( 0.9961946980917462113, 0.000000000000000000, -0.08715574274765118534 ) ) ;
#29555=CARTESIAN_POINT ( 'NONE',  ( 37.09755260828975310, 7.646167579472015790E-16, 162.3589405374562205 ) ) ;
#29568=CARTESIAN_POINT ( 'NONE',  ( 34.33409119757650529, -5.407089921784855591, 166.5908959372197558 ) ) ;
#29569=CARTESIAN_POINT ( 'NONE',  ( 23.87821517812500005, -4.985214923628404016, -3.140624999385472016 ) ) ;
#29572=CARTESIAN_POINT ( 'NONE',  ( 25.01527935017339033, 0.000000000000000000, 50.00000000000000000 ) ) ;
#29573=CARTESIAN_POINT ( 'NONE',  ( 25.08932009880328096, 0.000000000000000000, 165.5834220860826349 ) ) ;
#29577=VERTEX_POINT ( 'NONE', #13252 ) ;
#29578=ORIENTED_EDGE ( 'NONE', *, *, #908, .T. ) ;
#29581=CARTESIAN_POINT ( 'NONE',  ( 15.24356964375000167, -3.323476615752272600, -1.453124999385472016 ) ) ;
#29583=CARTESIAN_POINT ( 'NONE',  ( 18.00000000000000000, 5.196152422706630247, -7.668749998770957532 ) ) ;
#29588=CARTESIAN_POINT ( 'NONE',  ( 31.03952447949476223, 7.209453229046482114, 164.7522898954867401 ) ) ;
#29596=CARTESIAN_POINT ( 'NONE',  ( 28.09467017918796472, 5.407089921784856479, 166.9109150798468306 ) ) ;
#29607=ADVANCED_FACE ( 'NONE', ( #21228 ), #3958, .T. ) ;
#29610=CARTESIAN_POINT ( 'NONE',  ( 21.00000000000000355, 0.000000000000000000, 50.00000000000001421 ) ) ;
#29615=CARTESIAN_POINT ( 'NONE',  ( 28.29894145125277660, -5.407089921784865361, 169.2457464034993961 ) ) ;
#29616=CYLINDRICAL_SURFACE ( 'NONE', #31462, 6.000000000000001776 ) ;
#29618=LINE ( 'NONE', #3274, #33691 ) ;
#29624=CARTESIAN_POINT ( 'NONE',  ( 15.24356964375000167, -3.323476615752272600, -5.615624999385488536 ) ) ;
#29628=ORIENTED_EDGE ( 'NONE', *, *, #6337, .T. ) ;
#29629=CARTESIAN_POINT ( 'NONE',  ( 26.75643035624999655, 3.323476615752271268, -5.728124999385479477 ) ) ;
#29637=CARTESIAN_POINT ( 'NONE',  ( 30.77233765568754720, -6.928203230275506996, 161.6983305247614453 ) ) ;
#29642=CARTESIAN_POINT ( 'NONE',  ( 26.75643035624999655, -3.323476615752267271, -6.365624999385492089 ) ) ;
#29645=AXIS2_PLACEMENT_3D ( 'NONE', #26579, #4214, #12566 ) ;
#29651=( BOUNDED_CURVE ( )  B_SPLINE_CURVE ( 2, ( #2968, #14538, #678, #3155, #123, #32147, #20988 ),
 .UNSPECIFIED., .F., .F. ) 
 B_SPLINE_CURVE_WITH_KNOTS ( ( 3, 2, 2, 3 ),
 ( 0.3043478260869560970, 0.3115942028985501100, 0.3188405797101441785, 0.3260869565217382471 ),
 .UNSPECIFIED. ) 
 CURVE ( )  GEOMETRIC_REPRESENTATION_ITEM ( )  RATIONAL_B_SPLINE_CURVE ( ( 1.000000000000008216, 0.8660254037844304920, 1.000000000000000000, 0.8660254037844387076, 1.000000000000000000, 0.8660254037844551389, 0.9999999999999835687 ) ) 
 REPRESENTATION_ITEM ( '' )  );
#29652=CARTESIAN_POINT ( 'NONE',  ( 30.70615376348499836, -7.209453229046482114, 160.9418451752858346 ) ) ;
#29662=AXIS2_PLACEMENT_3D ( 'NONE', #35618, #27281, #6815 ) ;
#29664=CARTESIAN_POINT ( 'NONE',  ( 15.00000000000000000, 3.464101615137752166, -6.787499999999996092 ) ) ;
#29665=CARTESIAN_POINT ( 'NONE',  ( 26.99999999999991118, -3.464101615137797463, -4.312500000000005329 ) ) ;
#29668=CARTESIAN_POINT ( 'NONE',  ( 37.48975345065418452, 7.646167579472015790E-16, 166.8418166788690655 ) ) ;
#29672=ORIENTED_EDGE ( 'NONE', *, *, #30455, .T. ) ;
#29675=CARTESIAN_POINT ( 'NONE',  ( 21.00000000000000355, 0.000000000000000000, 50.00000000000001421 ) ) ;
#29677=CARTESIAN_POINT ( 'NONE',  ( 15.24356964374999990, 0.000000000000000000, -5.540624999385457272 ) ) ;
#29678=AXIS2_PLACEMENT_3D ( 'NONE', #28101, #7832, #36438 ) ;
#29685=CARTESIAN_POINT ( 'NONE',  ( 28.40800656884236730, -5.196152422706632912, 169.0950422780865097 ) ) ;
#29697=CARTESIAN_POINT ( 'NONE',  ( 34.42112650116913386, -5.196152422706635576, 168.9830381333390505 ) ) ;
#29698=CARTESIAN_POINT ( 'NONE',  ( 28.16820783713129472, 5.407089921784862696, 167.7514543563617622 ) ) ;
#29708=ORIENTED_EDGE ( 'NONE', *, *, #17924, .F. ) ;
#29709=CARTESIAN_POINT ( 'NONE',  ( 27.58480908411420529, 5.407089921784856479, 161.0831760960101349 ) ) ;
#29710=CARTESIAN_POINT ( 'NONE',  ( 26.75643035624999655, -3.323476615752267715, -8.953124999385474680 ) ) ;
#29712=CARTESIAN_POINT ( 'NONE',  ( 24.94391043663983965, 3.604726614523240613, 166.7160302899652322 ) ) ;
#29714=CARTESIAN_POINT ( 'NONE',  ( 25.01087993033039325, 0.000000000000000000, 164.6868468578000488 ) ) ;
#29721=ORIENTED_EDGE ( 'NONE', *, *, #21502, .F. ) ;
#29725=EDGE_CURVE ( 'NONE', #31979, #4816, #36179, .T. ) ;
#29726=CARTESIAN_POINT ( 'NONE',  ( 15.24356964375000167, -3.323476615752272600, -5.165624999385460825 ) ) ;
#29738=EDGE_CURVE ( 'NONE', #10416, #4247, #14496, .T. ) ;
#29741=CARTESIAN_POINT ( 'NONE',  ( 27.85934967376930516, 5.407089921784856479, 164.2211893949991293 ) ) ;
#29753=ORIENTED_EDGE ( 'NONE', *, *, #5769, .T. ) ;
#29754=CARTESIAN_POINT ( 'NONE',  ( 37.41131328218130392, 7.646167579472015790E-16, 165.9452414505865079 ) ) ;
#29755=CARTESIAN_POINT ( 'NONE',  ( 26.75643035624999655, -3.323476615752267715, -1.753124999385447857 ) ) ;
#29757=LINE ( 'NONE', #755, #19743 ) ;
#29760=LINE ( 'NONE', #32229, #32709 ) ;
#29767=CARTESIAN_POINT ( 'NONE',  ( 26.75643035624999655, -3.323476615752267715, -0.8531249993854884694 ) ) ;
#29769=CARTESIAN_POINT ( 'NONE',  ( 21.00000000000000000, 6.928203230275506996, -8.156249998770968901 ) ) ;
#29770=FACE_OUTER_BOUND ( 'NONE', #36472, .T. ) ;
#29778=CARTESIAN_POINT ( 'NONE',  ( 37.28875051894242887, 7.646167579472024665E-16, 164.5443426563950027 ) ) ;
#29785=CARTESIAN_POINT ( 'NONE',  ( 24.99456971211191814, -3.604726614523240613, 167.2950684582310146 ) ) ;
#29798=DIRECTION ( 'NONE',  ( 0.08715574274765150453, 0.000000000000000000, 0.9961946980917461003 ) ) ;
#29801=CARTESIAN_POINT ( 'NONE',  ( 20.99999999999999645, 0.000000000000000000, -8.000000000000000000 ) ) ;
#29802=CARTESIAN_POINT ( 'NONE',  ( 15.33009822426688729, 1.665651000388348013, -7.999999999999992895 ) ) ;
#29803=CARTESIAN_POINT ( 'NONE',  ( 36.79199426871969791, 3.464101615138157619, 161.6610409823709347 ) ) ;
#29812=CARTESIAN_POINT ( 'NONE',  ( 15.24356964374999990, 0.000000000000000000, -3.403124999385470417 ) ) ;
#29815=ORIENTED_EDGE ( 'NONE', *, *, #36432, .T. ) ;
#29816=CARTESIAN_POINT ( 'NONE',  ( 15.24356964374999990, 3.323476615752268604, -5.578124999385491556 ) ) ;
#29819=EDGE_CURVE ( 'NONE', #15328, #13615, #15609, .T. ) ;
#29820=VECTOR ( 'NONE', #1681, 1000.000000000000000 ) ;
#29828=CARTESIAN_POINT ( 'NONE',  ( 15.24356964374999990, 3.323476615752268604, -6.590624999385473970 ) ) ;
#29841=CARTESIAN_POINT ( 'NONE',  ( 14.99999999999945111, -3.464101615137439083, -1.256249998770955889 ) ) ;
#29849=CARTESIAN_POINT ( 'NONE',  ( 21.00000000000000000, 6.928203230275506996, -6.862499999999990941 ) ) ;
#29854=CARTESIAN_POINT ( 'NONE',  ( 31.27974749544297595, 7.209453229046475009, 167.4980515321021244 ) ) ;
#29864=DIRECTION ( 'NONE',  ( 0.000000000000000000, 0.000000000000000000, 1.000000000000000000 ) ) ;
#29867=CARTESIAN_POINT ( 'NONE',  ( 26.75643035624999655, 7.049594010296217766E-16, -8.015624999385462246 ) ) ;
#29870=ADVANCED_FACE ( 'NONE', ( #25687 ), #34404, .T. ) ;
#29874=DIRECTION ( 'NONE',  ( 0.08715574274765150453, 0.000000000000000000, 0.9961946980917461003 ) ) ;
#29875=CARTESIAN_POINT ( 'NONE',  ( 37.26590362001785905, -3.464101615137751278, 167.0778496544691052 ) ) ;
#29879=( BOUNDED_CURVE ( )  B_SPLINE_CURVE ( 2, ( #10483, #27919, #13151, #13718, #36074, #13335, #1950 ),
 .UNSPECIFIED., .F., .F. ) 
 B_SPLINE_CURVE_WITH_KNOTS ( ( 3, 2, 2, 3 ),
 ( 0.2391304347826092025, 0.2463768115942035208, 0.2536231884057978392, 0.2608695652173921298 ),
 .UNSPECIFIED. ) 
 CURVE ( )  GEOMETRIC_REPRESENTATION_ITEM ( )  RATIONAL_B_SPLINE_CURVE ( ( 0.9999999999999907851, 0.8660254037844479225, 1.000000000000000000, 0.8660254037844387076, 1.000000000000000000, 0.8660254037844232755, 1.000000000000015321 ) ) 
 REPRESENTATION_ITEM ( '' )  );
#29880=CIRCLE ( 'NONE', #8699, 6.000000000000001776 ) ;
#29890=CARTESIAN_POINT ( 'NONE',  ( 37.52407102436108488, 7.646167579472024665E-16, 167.2340683412427040 ) ) ;
#29901=FACE_OUTER_BOUND ( 'NONE', #20124, .T. ) ;
#29906=CARTESIAN_POINT ( 'NONE',  ( 18.00000000000000355, -5.196152422706632912, -0.8249999999999924061 ) ) ;
#29908=CARTESIAN_POINT ( 'NONE',  ( 27.94596069312478903, -5.407089921784865361, 165.2111578762278157 ) ) ;
#29909=CARTESIAN_POINT ( 'NONE',  ( 24.93243976185750554, 0.000000000000000000, 163.7902716295174912 ) ) ;
#29918=CARTESIAN_POINT ( 'NONE',  ( 15.24356964374999990, 0.000000000000000000, -7.003124999385490490 ) ) ;
#29926=VECTOR ( 'NONE', #15848, 1000.000000000000000 ) ;
#29936=CARTESIAN_POINT ( 'NONE',  ( 34.11184405356999605, 5.407089921784857367, 164.0505994570858093 ) ) ;
#29948=CARTESIAN_POINT ( 'NONE',  ( 37.36882485759182515, -3.604726614523235284, 165.4595965352667974 ) ) ;
#29949=CARTESIAN_POINT ( 'NONE',  ( 15.24356964374999990, 3.323476615752268604, -2.878124999385485161 ) ) ;
#29951=CARTESIAN_POINT ( 'NONE',  ( 25.04683167421347889, 3.464101615137573198, 165.0977771707629529 ) ) ;
#29953=CARTESIAN_POINT ( 'NONE',  ( 34.11717084844381986, -5.196152422706629359, 165.5088091249684510 ) ) ;
#29961=CARTESIAN_POINT ( 'NONE',  ( 21.00000000000000000, 6.646953231504538984, -2.053124999385488092 ) ) ;
#29963=CARTESIAN_POINT ( 'NONE',  ( 24.00000000000000000, -5.196152422706629359, -8.793749998770945098 ) ) ;
#29969=CARTESIAN_POINT ( 'NONE',  ( 37.17435860658612512, 3.604726614523243278, 163.2368371151495694 ) ) ;
#29972=CYLINDRICAL_SURFACE ( 'NONE', #21272, 6.000000000000001776 ) ;
#29975=CARTESIAN_POINT ( 'NONE',  ( 28.05545009495152087, 5.407089921784856479, 166.4626274657055660 ) ) ;
#29986=SHAPE_REPRESENTATION ( 'extension pipe', ( #17215 ), #34722 ) ;
#29995=CARTESIAN_POINT ( 'NONE',  ( 15.00000000000000000, 0.000000000000000000, -0.9000000000000119016 ) ) ;
#29996=CARTESIAN_POINT ( 'NONE',  ( 16.07423293023537525, 3.170634016558939727, -7.999999999999998224 ) ) ;
#29997=CARTESIAN_POINT ( 'NONE',  ( 36.71355410024671784, 3.464101615138219348, 160.7644657540884054 ) ) ;
#30001=AXIS2_PLACEMENT_3D ( 'NONE', #31949, #2766, #14338 ) ;
#30005=CARTESIAN_POINT ( 'NONE',  ( 15.24356964375000167, -3.323476615752272600, -4.265624999385501326 ) ) ;
#30008=ORIENTED_EDGE ( 'NONE', *, *, #27045, .T. ) ;
#30009=CARTESIAN_POINT ( 'NONE',  ( 18.12178482187500350, -4.985214923628407568, -7.265624999385461358 ) ) ;
#30016=CARTESIAN_POINT ( 'NONE',  ( 33.56808966913361303, -5.196152422706629359, 159.2327825269904622 ) ) ;
#30020=CARTESIAN_POINT ( 'NONE',  ( 15.24356964375000167, -3.323476615752272600, -6.065624999385484273 ) ) ;
#30024=DIRECTION ( 'NONE',  ( 0.9961946980917462113, 0.000000000000000000, -0.08715574274765118534 ) ) ;
#30028=CARTESIAN_POINT ( 'NONE',  ( 30.66693367924855096, -7.209453229046482114, 160.4935575611445415 ) ) ;
#30029=ORIENTED_EDGE ( 'NONE', *, *, #8012, .F. ) ;
#30041=CARTESIAN_POINT ( 'NONE',  ( 15.00000000000000178, -3.464101615137757051, -7.612499999999993605 ) ) ;
#30046=CARTESIAN_POINT ( 'NONE',  ( 34.19028422204287665, 5.407089921784857367, 164.9471746853683669 ) ) ;
#30052=ORIENTED_EDGE ( 'NONE', *, *, #17924, .T. ) ;
#30054=CARTESIAN_POINT ( 'NONE',  ( 20.99999999999999645, 6.646953231504538984, -1.153124999385464200 ) ) ;
#30055=CARTESIAN_POINT ( 'NONE',  ( 26.99999999999999645, 7.347880794884117764E-16, -1.124999999999987121 ) ) ;
#30057=CARTESIAN_POINT ( 'NONE',  ( 15.24356964374999990, 3.323476615752268604, -7.828124999385470240 ) ) ;
#30061=CARTESIAN_POINT ( 'NONE',  ( 24.86053627419733658, 3.464101615137476831, 162.9684110048161756 ) ) ;
#30063=CARTESIAN_POINT ( 'NONE',  ( 21.00000000000000355, 0.000000000000000000, 50.00000000000001421 ) ) ;
#30064=CARTESIAN_POINT ( 'NONE',  ( 37.22995187613445012, 7.347880794884117764E-16, 166.6669193415062580 ) ) ;
#30069=CARTESIAN_POINT ( 'NONE',  ( 29.51984097383938987, 5.908847061326898853, 159.3365289693693398 ) ) ;
#30078=CARTESIAN_POINT ( 'NONE',  ( 34.26382187998621731, 5.407089921784862696, 165.7877139618832985 ) ) ;
#30081=EDGE_CURVE ( 'NONE', #14162, #24412, #21697, .T. ) ;
#30093=ORIENTED_EDGE ( 'NONE', *, *, #29738, .T. ) ;
#30094=CARTESIAN_POINT ( 'NONE',  ( 24.44222019244867283, 0.000000000000000000, 160.9816845590745800 ) ) ;
#30096=CARTESIAN_POINT ( 'NONE',  ( 18.00000000000000000, 5.196152422706630247, -0.07499999999999173994 ) ) ;
#30097=VECTOR ( 'NONE', #10309, 1000.000000000000000 ) ;
#30098=CARTESIAN_POINT ( 'NONE',  ( 31.21356360324042356, 6.928203230275514990, 166.7415661826265421 ) ) ;
#30099=CARTESIAN_POINT ( 'NONE',  ( 37.16782192588006239, -3.604726614523238837, 163.1621225127927062 ) ) ;
#30100=CARTESIAN_POINT ( 'NONE',  ( 36.78545758801433152, -3.464101615137755275, 161.5863263800139862 ) ) ;
#30107=ORIENTED_EDGE ( 'NONE', *, *, #9772, .T. ) ;
#30112=CARTESIAN_POINT ( 'NONE',  ( 18.12178482187499640, 4.985214923628404904, -6.628124999385476279 ) ) ;
#30125=CARTESIAN_POINT ( 'NONE',  ( 37.17599277676264080, 7.646167579472015790E-16, 163.2555157657388065 ) ) ;
#30131=CARTESIAN_POINT ( 'NONE',  ( 23.99999999999999645, 5.196152422706631135, -2.343749998770960907 ) ) ;
#30137=CARTESIAN_POINT ( 'NONE',  ( 24.95534962787547073, -3.604726614523240613, 166.8467808440897500 ) ) ;
#30138=AXIS2_PLACEMENT_3D ( 'NONE', #45, #17131, #28667 ) ;
#30139=CARTESIAN_POINT ( 'NONE',  ( 26.75643035624999655, 7.049594010296217766E-16, -3.515624999385458249 ) ) ;
#30141=CARTESIAN_POINT ( 'NONE',  ( 23.30664739095454507, -5.481896322917826581, -8.000000000000001776 ) ) ;
#30142=CARTESIAN_POINT ( 'NONE',  ( 31.29200377171330771, 6.928203230275514990, 167.6381414109090997 ) ) ;
#30143=CARTESIAN_POINT ( 'NONE',  ( 26.99999999999952038, -3.464101615138027057, -7.406249998770969789 ) ) ;
#30145=CARTESIAN_POINT ( 'NONE',  ( 25.01087993033039325, 0.000000000000000000, 164.6868468578000488 ) ) ;
#30148=VERTEX_POINT ( 'NONE', #7101 ) ;
#30149=ORIENTED_EDGE ( 'NONE', *, *, #5304, .T. ) ;
#30153=CARTESIAN_POINT ( 'NONE',  ( 26.75643035624999655, -3.323476615752267715, -1.303124999385484095 ) ) ;
#30155=CARTESIAN_POINT ( 'NONE',  ( 21.00000000000000000, 6.646953231504538984, -0.3656249993854637226 ) ) ;
#30158=VERTEX_POINT ( 'NONE', #15060 ) ;
#30161=CARTESIAN_POINT ( 'NONE',  ( 34.06772145880400160, 5.407089921784862696, 163.5462758911768617 ) ) ;
#30168=CARTESIAN_POINT ( 'NONE',  ( 34.26872439051576436, 5.407089921784857367, 165.8437499136509814 ) ) ;
#30182=DIRECTION ( 'NONE',  ( 0.9961946980917462113, 0.000000000000000000, -0.08715574274765178209 ) ) ;
#30185=CARTESIAN_POINT ( 'NONE',  ( 21.00000000000000355, 0.000000000000000000, 50.00000000000001421 ) ) ;
#30188=CARTESIAN_POINT ( 'NONE',  ( 36.82794601260381029, 7.347880794884125653E-16, 162.0719712953337250 ) ) ;
#30195=CARTESIAN_POINT ( 'NONE',  ( 15.24356964374999990, 0.000000000000000000, -5.203124999385494220 ) ) ;
#30209=ADVANCED_FACE ( 'NONE', ( #12774 ), #21510, .T. ) ;
#30211=CARTESIAN_POINT ( 'NONE',  ( 15.24356964374999990, 0.000000000000000000, -6.103124999385478588 ) ) ;
#30212=DIRECTION ( 'NONE',  ( 0.08715574274765150453, 0.000000000000000000, 0.9961946980917461003 ) ) ;
#30221=ORIENTED_EDGE ( 'NONE', *, *, #14345, .F. ) ;
#30227=CARTESIAN_POINT ( 'NONE',  ( 24.99999999999999289, 0.000000000000000000, 49.65004534589634488 ) ) ;
#30237=CARTESIAN_POINT ( 'NONE',  ( 27.85934967376930516, 5.407089921784856479, 164.2211893949991293 ) ) ;
#30238=CARTESIAN_POINT ( 'NONE',  ( 25.44230085693126497, 0.000000000000000000, 169.6180106133541869 ) ) ;
#30248=CARTESIAN_POINT ( 'NONE',  ( 18.12178482187500350, -4.985214923628407568, -9.515624999385464022 ) ) ;
#30254=CYLINDRICAL_SURFACE ( 'NONE', #12518, 6.000000000000001776 ) ;
#30255=CARTESIAN_POINT ( 'NONE',  ( 34.13024420985595953, 5.196152422706631135, 165.6582383296822343 ) ) ;
#30257=EDGE_CURVE ( 'NONE', #30542, #30763, #29879, .T. ) ;
#30262=CARTESIAN_POINT ( 'NONE',  ( 18.12178482187499640, 4.985214923628404904, -0.7781249993854821856 ) ) ;
#30268=CARTESIAN_POINT ( 'NONE',  ( 27.87526709119022783, 5.196152422706636465, 163.0058021847763712 ) ) ;
#30270=CARTESIAN_POINT ( 'NONE',  ( 24.82951852428355011, 0.000000000000000000, 165.4085247487197989 ) ) ;
#30282=ORIENTED_EDGE ( 'NONE', *, *, #13782, .T. ) ;
#30283=FACE_OUTER_BOUND ( 'NONE', #27514, .T. ) ;
#30285=CARTESIAN_POINT ( 'NONE',  ( 23.99999999999999645, 5.196152422706631135, -1.950000000000007283 ) ) ;
#30288=CARTESIAN_POINT ( 'NONE',  ( 30.86303410043077022, -7.209453229046482114, 162.7349956318509783 ) ) ;
#30289=CARTESIAN_POINT ( 'NONE',  ( 30.70370250816666058, 6.928203230275514990, 160.9138271987898463 ) ) ;
#30299=CARTESIAN_POINT ( 'NONE',  ( 21.00000000000000000, -6.646953231504538984, -6.890624999385480898 ) ) ;
#30314=CARTESIAN_POINT ( 'NONE',  ( 30.94637677943320497, -7.209453229046475009, 163.6876068119012189 ) ) ;
#30317=CARTESIAN_POINT ( 'NONE',  ( 26.99999999999999645, 7.347880794884117764E-16, -3.768749998770942966 ) ) ;
#30318=DIRECTION ( 'NONE',  ( 0.08715574274765150453, 0.000000000000000000, 0.9961946980917461003 ) ) ;
#30320=CARTESIAN_POINT ( 'NONE',  ( 15.00000000000008171, -3.464101615137802348, -4.406249998770950249 ) ) ;
#30326=CARTESIAN_POINT ( 'NONE',  ( 37.25443294523552851, 7.646167579472015790E-16, 164.1520909940213642 ) ) ;
#30327=CARTESIAN_POINT ( 'NONE',  ( 26.75643035624999655, 7.049594010296217766E-16, -3.965624999385464200 ) ) ;
#30329=CARTESIAN_POINT ( 'NONE',  ( 37.33780710767756972, 7.347880794884125653E-16, 167.8997102791704492 ) ) ;
#30330=CARTESIAN_POINT ( 'NONE',  ( 15.24356964374999990, 0.000000000000000000, -0.1406249993854691294 ) ) ;
#30340=CARTESIAN_POINT ( 'NONE',  ( 26.75643035624999655, 3.323476615752271712, -3.478124999385468819 ) ) ;
#30342=EDGE_CURVE ( 'NONE', #27706, #15426, #27225, .T. ) ;
#30343=CARTESIAN_POINT ( 'NONE',  ( 26.99999999999999645, 3.464101615137755275, -9.131249998770954335 ) ) ;
#30344=ORIENTED_EDGE ( 'NONE', *, *, #35976, .T. ) ;
#30350=CARTESIAN_POINT ( 'NONE',  ( 36.97498984505087805, 7.646167579472024665E-16, 160.9580417432647153 ) ) ;
#30351=EDGE_CURVE ( 'NONE', #10416, #952, #24572, .T. ) ;
#30360=CARTESIAN_POINT ( 'NONE',  ( 18.00000000000000355, -5.196152422706632912, -5.324999999999996625 ) ) ;
#30368=CARTESIAN_POINT ( 'NONE',  ( 20.99999999999999645, 0.000000000000000000, -8.000000000000000000 ) ) ;
#30371=CYLINDRICAL_SURFACE ( 'NONE', #4855, 4.000000000000000888 ) ;
#30375=DIRECTION ( 'NONE',  ( 1.000000000000000000, 0.000000000000000000, 0.000000000000000000 ) ) ;
#30377=CARTESIAN_POINT ( 'NONE',  ( 17.00000000000000000, 4.898587196589406912E-16, 50.17464377163448574 ) ) ;
#30378=CARTESIAN_POINT ( 'NONE',  ( 21.00000000000000355, 0.000000000000000000, 50.00000000000001421 ) ) ;
#30380=ORIENTED_EDGE ( 'NONE', *, *, #15016, .T. ) ;
#30386=CARTESIAN_POINT ( 'NONE',  ( 26.75643035624999655, 7.049594010296217766E-16, -4.528124999385485516 ) ) ;
#30389=CARTESIAN_POINT ( 'NONE',  ( 20.99999999999999645, -6.646953231504538984, -7.228124999385454608 ) ) ;
#30396=CARTESIAN_POINT ( 'NONE',  ( 24.59253236524878616, -3.464101615137757051, 159.9051123081840160 ) ) ;
#30400=EDGE_CURVE ( 'NONE', #21723, #8971, #9074, .T. ) ;
#30402=CARTESIAN_POINT ( 'NONE',  ( 36.79526260918112257, -3.464101615137414214, 161.6983982847735888 ) ) ;
#30410=ORIENTED_EDGE ( 'NONE', *, *, #25721, .T. ) ;
#30425=CARTESIAN_POINT ( 'NONE',  ( 24.77555942491173369, 0.000000000000000000, 161.9971211729523475 ) ) ;
#30429=CARTESIAN_POINT ( 'NONE',  ( 37.21194452064604974, -3.604726614523235284, 163.6664460787016253 ) ) ;
#30430=CARTESIAN_POINT ( 'NONE',  ( 20.99999999999999645, 6.928203230275506996, -1.912500000000006306 ) ) ;
#30433=EDGE_LOOP ( 'NONE', ( #1503, #15521, #16938 ) ) ;
#30438=CARTESIAN_POINT ( 'NONE',  ( 25.25600545691528254, 0.000000000000000000, 167.4886444474074381 ) ) ;
#30440=LINE ( 'NONE', #16224, #29926 ) ;
#30441=CARTESIAN_POINT ( 'NONE',  ( 26.75643035624999655, 7.049594010296217766E-16, -9.365624999385479654 ) ) ;
#30444=EDGE_CURVE ( 'NONE', #30939, #17372, #6415, .T. ) ;
#30446=( BOUNDED_CURVE ( )  B_SPLINE_CURVE ( 2, ( #9259, #7487, #18174, #3748, #21713, #6411, #32373 ),
 .UNSPECIFIED., .F., .F. ) 
 B_SPLINE_CURVE_WITH_KNOTS ( ( 3, 2, 2, 3 ),
 ( 0.3478260869565213409, 0.3550724637681154094, 0.3623188405797093670, 0.3695652173913033800 ),
 .UNSPECIFIED. ) 
 CURVE ( )  GEOMETRIC_REPRESENTATION_ITEM ( )  RATIONAL_B_SPLINE_CURVE ( ( 1.000000000000007105, 0.8660254037844313801, 1.000000000000000000, 0.8660254037844387076, 1.000000000000000000, 0.8660254037844561381, 0.9999999999999825695 ) ) 
 REPRESENTATION_ITEM ( '' )  );
#30447=B_SPLINE_CURVE_WITH_KNOTS ( 'NONE', 3,
 ( #7587, #22185, #1887, #13458 ),
 .UNSPECIFIED., .F., .F.,
 ( 4, 4 ),
 ( 0.000000000000000000, 1.000000000000000000 ),
 .UNSPECIFIED. ) ;
#30451=CARTESIAN_POINT ( 'NONE',  ( 37.19400013225104118, 3.464101615137755275, 166.2559890285434108 ) ) ;
#30455=EDGE_CURVE ( 'NONE', #11570, #9957, #11284, .T. ) ;
#30457=CARTESIAN_POINT ( 'NONE',  ( 18.12178482187500350, -4.985214923628407568, -1.978124999385488803 ) ) ;
#30461=EDGE_LOOP ( 'NONE', ( #9775, #31134, #10436, #36203, #1130, #7414, #35374, #19768, #9875, #29054, #25806, #14255, #12262, #34516, #19994, #37221, #34525, #22969, #20674, #1960, #31577, #34875, #25948, #24393, #13703, #8959, #15044, #14180, #15737, #34847, #10932, #2359, #14152, #22837, #19062, #1713, #5360 ) ) ;
#30463=CARTESIAN_POINT ( 'NONE',  ( 31.45868912971819142, 0.000000000000000000, 169.5433637710095809 ) ) ;
#30465=CARTESIAN_POINT ( 'NONE',  ( 37.28875051894242887, 7.646167579472024665E-16, 164.5443426563950027 ) ) ;
#30470=CARTESIAN_POINT ( 'NONE',  ( 18.00000000000000000, 5.196152422706630247, -2.718749998770947585 ) ) ;
#30474=CARTESIAN_POINT ( 'NONE',  ( 20.99999999999999645, -6.928203230275506996, -7.931249998770954157 ) ) ;
#30478=CARTESIAN_POINT ( 'NONE',  ( 27.00000000000036593, -3.464101615137536783, -6.056249998770942611 ) ) ;
#30479=VERTEX_POINT ( 'NONE', #29023 ) ;
#30480=CARTESIAN_POINT ( 'NONE',  ( 24.00000000000000000, -5.196152422706629359, -3.000000000000002665 ) ) ;
#30482=CARTESIAN_POINT ( 'NONE',  ( 30.82381401619432992, -7.209453229046482114, 162.2867080177096852 ) ) ;
#30483=CARTESIAN_POINT ( 'NONE',  ( 33.72823834632531259, 5.196152422706637353, 161.0632902835097013 ) ) ;
#30493=CARTESIAN_POINT ( 'NONE',  ( 15.24356964374999990, 3.323476615752268604, -7.490624999385497418 ) ) ;
#30497=ADVANCED_FACE ( 'NONE', ( #26187 ), #37189, .T. ) ;
#30498=CARTESIAN_POINT ( 'NONE',  ( 25.48152094116770883, 0.000000000000000000, 170.0662982274954800 ) ) ;
#30507=VECTOR ( 'NONE', #26485, 1000.000000000000000 ) ;
#30509=CARTESIAN_POINT ( 'NONE',  ( 36.98316069593346356, 3.604726614523238837, 161.0514349962108156 ) ) ;
#30519=CARTESIAN_POINT ( 'NONE',  ( 27.85934967376930516, 5.407089921784856479, 164.2211893949991293 ) ) ;
#30520=CARTESIAN_POINT ( 'NONE',  ( 18.12178482187499640, 4.985214923628404904, -4.265624999385458693 ) ) ;
#30523=CARTESIAN_POINT ( 'NONE',  ( 31.44888410865908313, 6.928203230275514990, 169.4312918674742434 ) ) ;
#30529=ORIENTED_EDGE ( 'NONE', *, *, #4696, .T. ) ;
#30535=CARTESIAN_POINT ( 'NONE',  ( 26.75643035624999655, 3.323476615752271712, -3.928124999385464999 ) ) ;
#30539=CARTESIAN_POINT ( 'NONE',  ( 26.99999999999999645, -3.464101615137751278, -8.756249998770950782 ) ) ;
#30542=VERTEX_POINT ( 'NONE', #16504 ) ;
#30546=CARTESIAN_POINT ( 'NONE',  ( 36.89654967657799745, 7.646167579472024665E-16, 160.0614665149821576 ) ) ;
#30554=ORIENTED_EDGE ( 'NONE', *, *, #7478, .F. ) ;
#30572=CARTESIAN_POINT ( 'NONE',  ( 25.05010001456683710, 0.000000000000000000, 165.1351344719413419 ) ) ;
#30576=ORIENTED_EDGE ( 'NONE', *, *, #33218, .T. ) ;
#30581=CARTESIAN_POINT ( 'NONE',  ( 26.75643035624999655, -3.323476615752267715, -6.365624999385492089 ) ) ;
#30584=CARTESIAN_POINT ( 'NONE',  ( 15.24356964374999990, 0.000000000000000000, -7.790624999385459049 ) ) ;
#30586=CARTESIAN_POINT ( 'NONE',  ( 25.18249928241153413, 0.000000000000000000, 169.4431132759913794 ) ) ;
#30593=CARTESIAN_POINT ( 'NONE',  ( 18.91026388320226914, 5.440443521936087379, -7.988398020327252880 ) ) ;
#30603=ORIENTED_EDGE ( 'NONE', *, *, #11723, .F. ) ;
#30607=CARTESIAN_POINT ( 'NONE',  ( 27.84912036836594140, -5.196152422706638241, 162.7069437753488046 ) ) ;
#30614=ORIENTED_EDGE ( 'NONE', *, *, #24095, .T. ) ;
#30618=CARTESIAN_POINT ( 'NONE',  ( 27.87242303518145548, -5.407089921784859143, 164.3706185997128841 ) ) ;
#30619=CARTESIAN_POINT ( 'NONE',  ( 36.90638618107669799, 7.347880794884125653E-16, 162.9685465236163111 ) ) ;
#30625=CARTESIAN_POINT ( 'NONE',  ( 23.99999999999999645, 5.196152422706631135, -5.043749998770941545 ) ) ;
#30627=CARTESIAN_POINT ( 'NONE',  ( 24.89321967762106169, 0.000000000000000000, 163.3419840153761982 ) ) ;
#30629=CARTESIAN_POINT ( 'NONE',  ( 18.12178482187500350, -4.985214923628407568, -9.965624999385468641 ) ) ;
#30635=CARTESIAN_POINT ( 'NONE',  ( 37.15478004801459377, 3.464101615137755275, 165.8077014144021462 ) ) ;
#30640=CARTESIAN_POINT ( 'NONE',  ( 26.75643035624999655, 3.323476615752271268, -2.690624999385500704 ) ) ;
#30649=CARTESIAN_POINT ( 'NONE',  ( 28.12039261777511356, 5.196152422706630247, 165.8075997743837604 ) ) ;
#30650=CARTESIAN_POINT ( 'NONE',  ( 27.89366724747619131, 5.407089921784862696, 164.6134410573727678 ) ) ;
#30663=DIRECTION ( 'NONE',  ( 0.000000000000000000, 0.000000000000000000, 1.000000000000000000 ) ) ;
#30665=CARTESIAN_POINT ( 'NONE',  ( 15.00000000000000000, 0.000000000000000000, -1.349999999999990097 ) ) ;
#30666=CARTESIAN_POINT ( 'NONE',  ( 37.05343001352376575, 7.646167579472024665E-16, 161.8546169715473013 ) ) ;
#30667=CARTESIAN_POINT ( 'NONE',  ( 24.77229108455869522, 3.464101615137757051, 161.9597638717739017 ) ) ;
#30669=CYLINDRICAL_SURFACE ( 'NONE', #30670, 6.000000000000001776 ) ;
#30670=AXIS2_PLACEMENT_3D ( 'NONE', #27818, #7730, #13235 ) ;
#30671=( BOUNDED_CURVE ( )  B_SPLINE_CURVE ( 2, ( #5018, #33838, #16410, #13004, #10339, #21727, #21544 ),
 .UNSPECIFIED., .F., .F. ) 
 B_SPLINE_CURVE_WITH_KNOTS ( ( 3, 2, 2, 3 ),
 ( 0.6956521739130424598, 0.7028985507246365838, 0.7101449275362308189, 0.7173913043478248319 ),
 .UNSPECIFIED. ) 
 CURVE ( )  GEOMETRIC_REPRESENTATION_ITEM ( )  RATIONAL_B_SPLINE_CURVE ( ( 1.000000000000018430, 0.8660254037844202779, 1.000000000000000000, 0.8660254037844387076, 1.000000000000000000, 0.8660254037844612451, 0.9999999999999774625 ) ) 
 REPRESENTATION_ITEM ( '' )  );
#30675=VERTEX_POINT ( 'NONE', #13661 ) ;
#30678=CARTESIAN_POINT ( 'NONE',  ( 23.87821517812500005, -4.985214923628404016, -6.853124999385479477 ) ) ;
#30681=AXIS2_PLACEMENT_3D ( 'NONE', #30463, #35234, #11930 ) ;
#30693=CARTESIAN_POINT ( 'NONE',  ( 24.63505227327785363, 3.604726614523236616, 163.1857653286025709 ) ) ;
#30694=CARTESIAN_POINT ( 'NONE',  ( 26.99999999999999645, 3.464101615137755275, -0.5812499987709716098 ) ) ;
#30703=CARTESIAN_POINT ( 'NONE',  ( 24.83768937516613917, -3.604726614523240613, 165.5019180016658993 ) ) ;
#30704=CARTESIAN_POINT ( 'NONE',  ( 21.00000000000000000, 6.646953231504538984, -6.103124999385481253 ) ) ;
#30708=CARTESIAN_POINT ( 'NONE',  ( 16.83508850220853148, 4.102936442506299741, -8.000000000000000000 ) ) ;
#30709=CARTESIAN_POINT ( 'NONE',  ( 31.40966402442264283, 6.928203230275514990, 168.9830042533329504 ) ) ;
#30712=LINE ( 'NONE', #1698, #5748 ) ;
#30716=ORIENTED_EDGE ( 'NONE', *, *, #19236, .T. ) ;
#30719=CARTESIAN_POINT ( 'NONE',  ( 23.87821517812499650, 4.985214923628404904, -3.440624999385466509 ) ) ;
#30722=CARTESIAN_POINT ( 'NONE',  ( 15.00000000000000178, -3.464101615137757051, -9.806249998770931953 ) ) ;
#30737=CARTESIAN_POINT ( 'NONE',  ( 15.00000000000000000, 0.000000000000000000, -5.399999999999987921 ) ) ;
#30749=CARTESIAN_POINT ( 'NONE',  ( 15.00000000000021316, -3.464101615137879620, -5.812500000000008882 ) ) ;
#30751=CARTESIAN_POINT ( 'NONE',  ( 15.00000000000045297, -3.464101615138017287, -1.706249998770939191 ) ) ;
#30754=CARTESIAN_POINT ( 'NONE',  ( 18.00000000000000000, 5.196152422706630247, -9.975000000000012079 ) ) ;
#30761=CARTESIAN_POINT ( 'NONE',  ( 15.24356964374999990, 0.000000000000000000, -7.003124999385490490 ) ) ;
#30763=VERTEX_POINT ( 'NONE', #5299 ) ;
#30777=CARTESIAN_POINT ( 'NONE',  ( 26.99999999999999289, 0.000000000000000000, -8.000000000000000000 ) ) ;
#30797=CARTESIAN_POINT ( 'NONE',  ( 24.55988044515800439, 0.000000000000000000, 162.3265474014984591 ) ) ;
#30798=FACE_OUTER_BOUND ( 'NONE', #22177, .T. ) ;
#30805=CARTESIAN_POINT ( 'NONE',  ( 21.00000000000000000, 6.928203230275506996, -3.656249998770947585 ) ) ;
#30806=CARTESIAN_POINT ( 'NONE',  ( 23.87821517812499650, 4.985214923628404904, -0.7406249993854585600 ) ) ;
#30808=CARTESIAN_POINT ( 'NONE',  ( 23.99999999999999645, 5.196152422706631135, -4.649999999999987921 ) ) ;
#30816=CARTESIAN_POINT ( 'NONE',  ( 34.01258395714663152, 5.196152422706631135, 164.3133754872583836 ) ) ;
#30822=CARTESIAN_POINT ( 'NONE',  ( 15.24356964374999990, 3.323476615752268604, -1.640624999385488891 ) ) ;
#30827=CARTESIAN_POINT ( 'NONE',  ( 25.25600545691528254, 0.000000000000000000, 167.4886444474074381 ) ) ;
#30830=PLANE ( 'NONE',  #4745 ) ;
#30831=CARTESIAN_POINT ( 'NONE',  ( 24.79356678040014117, -3.604726614523244610, 164.9975944357569517 ) ) ;
#30836=CARTESIAN_POINT ( 'NONE',  ( 27.00000000000023448, 3.464101615137617163, -2.831249998770953180 ) ) ;
#30846=CARTESIAN_POINT ( 'NONE',  ( 21.00000000000000000, -6.928203230275506996, -1.687500000000023981 ) ) ;
#30847=CARTESIAN_POINT ( 'NONE',  ( 22.38931379102810837, -5.788467285583099198, -8.000000000000003553 ) ) ;
#30848=CARTESIAN_POINT ( 'NONE',  ( 24.63668644345436931, -3.604726614523244610, 163.2044439791918080 ) ) ;
#30849=CARTESIAN_POINT ( 'NONE',  ( 24.77555942491173369, 0.000000000000000000, 161.9971211729523475 ) ) ;
#30857=CARTESIAN_POINT ( 'NONE',  ( 15.00000000000000000, 0.000000000000000000, -4.049999999999998046 ) ) ;
#30859=CARTESIAN_POINT ( 'NONE',  ( 15.24356964374999990, 3.323476615752268604, -9.740624999385508076 ) ) ;
#30873=CARTESIAN_POINT ( 'NONE',  ( 30.71105627401454896, -7.209453229046475009, 160.9978811270534891 ) ) ;
#30874=CARTESIAN_POINT ( 'NONE',  ( 24.00000000000000000, -5.196152422706629359, -1.143749998770954290 ) ) ;
#30884=CARTESIAN_POINT ( 'NONE',  ( 34.22950430627932406, 5.407089921784857367, 165.3954622995096599 ) ) ;
#30885=CARTESIAN_POINT ( 'NONE',  ( 15.24356964375000167, -3.323476615752272600, -5.953124999385460470 ) ) ;
#30887=CARTESIAN_POINT ( 'NONE',  ( 25.21845102629494306, 3.604726614523240613, 169.8540435889542266 ) ) ;
#30888=CARTESIAN_POINT ( 'NONE',  ( 37.30185536379416078, 3.464101615137759271, 167.4887799662076020 ) ) ;
#30892=ADVANCED_FACE ( 'NONE', ( #7949 ), #4904, .F. ) ;
#30896=ORIENTED_EDGE ( 'NONE', *, *, #2236, .F. ) ;
#30900=CARTESIAN_POINT ( 'NONE',  ( 18.12178482187500350, -4.985214923628407568, -4.115624999385475213 ) ) ;
#30903=CARTESIAN_POINT ( 'NONE',  ( 18.12178482187500350, -4.985214923628407568, -1.528124999385482852 ) ) ;
#30930=CARTESIAN_POINT ( 'NONE',  ( 15.00000000000000000, 0.000000000000000000, -2.700000000000008171 ) ) ;
#30933=CARTESIAN_POINT ( 'NONE',  ( 26.99999999999999645, 7.347880794884117764E-16, -5.624999999999991118 ) ) ;
#30936=CYLINDRICAL_SURFACE ( 'NONE', #28454, 6.000000000000001776 ) ;
#30939=VERTEX_POINT ( 'NONE', #7763 ) ;
#30945=CARTESIAN_POINT ( 'NONE',  ( 15.24356964375000167, -3.323476615752272600, -7.415624999385471483 ) ) ;
#30948=EDGE_LOOP ( 'NONE', ( #31672, #34220, #8294, #26542 ) ) ;
#30953=CARTESIAN_POINT ( 'NONE',  ( 28.28586808984062628, 5.407089921784862696, 169.0963171987856128 ) ) ;
#30961=CARTESIAN_POINT ( 'NONE',  ( 24.82785287066792179, -3.464101615138032830, 162.5948379930317174 ) ) ;
#30970=LINE ( 'NONE', #13343, #30097 ) ;
#30971=ORIENTED_EDGE ( 'NONE', *, *, #9243, .T. ) ;
#30975=CARTESIAN_POINT ( 'NONE',  ( 36.82794601260381029, 7.347880794884125653E-16, 162.0719712953337250 ) ) ;
#30976=CARTESIAN_POINT ( 'NONE',  ( 36.63184559142159458, 7.347880794884125653E-16, 159.8305332246273167 ) ) ;
#30977=LINE ( 'NONE', #2151, #8732 ) ;
#30989=CARTESIAN_POINT ( 'NONE',  ( 27.71554269823568362, -5.407089921784859143, 162.5774681431477404 ) ) ;
#30990=CARTESIAN_POINT ( 'NONE',  ( 26.75643035624999655, 3.323476615752271712, -0.8906249993854854496 ) ) ;
#30996=CARTESIAN_POINT ( 'NONE',  ( 18.00000000000000355, -5.196152422706632912, -4.818749998770965881 ) ) ;
#30997=CARTESIAN_POINT ( 'NONE',  ( 26.75643035624999655, -3.323476615752267271, -1.753124999385447857 ) ) ;
#30998=DIRECTION ( 'NONE',  ( 0.08715574274765150453, 0.000000000000000000, 0.9961946980917461003 ) ) ;
#30999=DIRECTION ( 'NONE',  ( 0.08715574274765150453, 0.000000000000000000, 0.9961946980917461003 ) ) ;
#31006=CARTESIAN_POINT ( 'NONE',  ( 36.99136303036276274, -3.464101615137751278, 163.9398363554801108 ) ) ;
#31010=CARTESIAN_POINT ( 'NONE',  ( 26.75643035624999655, 7.049594010296217766E-16, -2.728124999385489247 ) ) ;
#31018=CARTESIAN_POINT ( 'NONE',  ( 37.28548217858939040, -3.604726614523238837, 164.5069853552165284 ) ) ;
#31024=DIRECTION ( 'NONE',  ( 0.08715574274765150453, 0.000000000000000000, 0.9961946980917461003 ) ) ;
#31029=CYLINDRICAL_SURFACE ( 'NONE', #230, 6.000000000000001776 ) ;
#31033=ORIENTED_EDGE ( 'NONE', *, *, #33476, .T. ) ;
#31034=CARTESIAN_POINT ( 'NONE',  ( 21.00000000000000000, -6.928203230275506996, -3.037500000000010747 ) ) ;
#31035=CARTESIAN_POINT ( 'NONE',  ( 25.07590970989797086, -4.251393452926127914, -7.999999999999994671 ) ) ;
#31036=CARTESIAN_POINT ( 'NONE',  ( 29.48995970988985604, 6.148715791637016537, 159.4803054849043917 ) ) ;
#31038=CARTESIAN_POINT ( 'NONE',  ( 36.59262550718515428, 7.347880794884125653E-16, 159.3822456104860237 ) ) ;
#31044=ORIENTED_EDGE ( 'NONE', *, *, #908, .F. ) ;
#31045=ORIENTED_EDGE ( 'NONE', *, *, #32573, .F. ) ;
#31047=LINE ( 'NONE', #10387, #8970 ) ;
#31049=CARTESIAN_POINT ( 'NONE',  ( 18.12178482187500350, -4.985214923628407568, -10.07812499938548534 ) ) ;
#31052=CARTESIAN_POINT ( 'NONE',  ( 14.99999999999978684, 3.464101615137630485, -6.281249998770925380 ) ) ;
#31062=CARTESIAN_POINT ( 'NONE',  ( 30.67183618977810156, -7.209453229046475009, 160.5495935129122245 ) ) ;
#31074=CARTESIAN_POINT ( 'NONE',  ( 37.17926111711567927, 3.604726614523238837, 163.2928730669172239 ) ) ;
#31075=CARTESIAN_POINT ( 'NONE',  ( 15.24356964374999990, 0.000000000000000000, -5.540624999385457272 ) ) ;
#31077=CARTESIAN_POINT ( 'NONE',  ( 31.39250523762275691, 7.209453229046482114, 168.7868784227583205 ) ) ;
#31078=CARTESIAN_POINT ( 'NONE',  ( 37.22341519532126597, 3.464101615137759271, 166.5922047379250159 ) ) ;
#31088=CARTESIAN_POINT ( 'NONE',  ( 18.12178482187500350, -4.985214923628407568, -3.665624999385469707 ) ) ;
#31092=CARTESIAN_POINT ( 'NONE',  ( 21.00000000000000000, -6.646953231504538984, -1.040624999385473481 ) ) ;
#31108=DIRECTION ( 'NONE',  ( 0.08715574274765150453, 0.000000000000000000, 0.9961946980917461003 ) ) ;
#31113=CARTESIAN_POINT ( 'NONE',  ( 15.00000000000000000, 0.000000000000000000, -4.443749998770951670 ) ) ;
#31127=CARTESIAN_POINT ( 'NONE',  ( 15.00000000000000000, 0.000000000000000000, -9.449999999999986855 ) ) ;
#31132=CARTESIAN_POINT ( 'NONE',  ( 26.75643035624999655, 3.323476615752271712, -5.840624999385470417 ) ) ;
#31134=ORIENTED_EDGE ( 'NONE', *, *, #24239, .F. ) ;
#31137=CARTESIAN_POINT ( 'NONE',  ( 28.22050128277989245, -5.407089921784865361, 168.3491711752168385 ) ) ;
#31140=( BOUNDED_CURVE ( )  B_SPLINE_CURVE ( 2, ( #14885, #35147, #3503, #20961, #21336, #17922, #32493 ),
 .UNSPECIFIED., .F., .F. ) 
 B_SPLINE_CURVE_WITH_KNOTS ( ( 3, 2, 2, 3 ),
 ( 0.1521739130434776044, 0.1594202898550718950, 0.1666666666666661856, 0.1739130434782605039 ),
 .UNSPECIFIED. ) 
 CURVE ( )  GEOMETRIC_REPRESENTATION_ITEM ( )  RATIONAL_B_SPLINE_CURVE ( ( 1.000000000000012212, 0.8660254037844263841, 1.000000000000000000, 0.8660254037844387076, 1.000000000000000000, 0.8660254037844453689, 0.9999999999999933387 ) ) 
 REPRESENTATION_ITEM ( '' )  );
#31141=CARTESIAN_POINT ( 'NONE',  ( 15.00000000000037481, -3.464101615137971546, -7.612499999999990941 ) ) ;
#31160=CARTESIAN_POINT ( 'NONE',  ( 25.29195720079856713, 3.464101615137683332, 167.8995747603702853 ) ) ;
#31161=CARTESIAN_POINT ( 'NONE',  ( 26.99999999999999645, 7.347880794884117764E-16, -5.568749998770966769 ) ) ;
#31173=CARTESIAN_POINT ( 'NONE',  ( 24.52066036092156054, 0.000000000000000000, 161.8782597873571660 ) ) ;
#31174=CARTESIAN_POINT ( 'NONE',  ( 30.91941297146709644, -6.928203230275514990, 163.3794090765669011 ) ) ;
#31177=ORIENTED_EDGE ( 'NONE', *, *, #23485, .F. ) ;
#31179=CARTESIAN_POINT ( 'NONE',  ( 26.99999999999999645, 7.347880794884117764E-16, -4.218749998770948473 ) ) ;
#31180=CARTESIAN_POINT ( 'NONE',  ( 20.99999999999999645, 6.646953231504538984, -2.953124999385479121 ) ) ;
#31182=CARTESIAN_POINT ( 'NONE',  ( 25.40308077269482112, 0.000000000000000000, 169.1697229992128939 ) ) ;
#31188=CARTESIAN_POINT ( 'NONE',  ( 25.01741661114358450, 3.464101615137752166, 164.7615614613812625 ) ) ;
#31192=CARTESIAN_POINT ( 'NONE',  ( 26.75643035624999655, -3.323476615752267271, -2.315624999385466509 ) ) ;
#31196=VERTEX_POINT ( 'NONE', #517 ) ;
#31202=CARTESIAN_POINT ( 'NONE',  ( 37.05343001352376575, 7.646167579472024665E-16, 161.8546169715473013 ) ) ;
#31214=CARTESIAN_POINT ( 'NONE',  ( 23.99999999999999645, 5.196152422706631135, -3.750000000000003553 ) ) ;
#31215=CARTESIAN_POINT ( 'NONE',  ( 26.30554917760220590, -2.480918870684495126, -8.000000000000003553 ) ) ;
#31216=CARTESIAN_POINT ( 'NONE',  ( 27.63220001923324176, -5.407089921784865361, 161.6248569630975283 ) ) ;
#31218=CARTESIAN_POINT ( 'NONE',  ( 34.49097153452227360, -5.407089921784855591, 168.3840463937848995 ) ) ;
#31222=ORIENTED_EDGE ( 'NONE', *, *, #35785, .F. ) ;
#31223=VERTEX_POINT ( 'NONE', #29521 ) ;
#31226=CARTESIAN_POINT ( 'NONE',  ( 24.78209610572444532, 3.464101615137476831, 162.0718357765335895 ) ) ;
#31228=CARTESIAN_POINT ( 'NONE',  ( 15.24356964374999990, 3.323476615752268604, -7.940624999385462068 ) ) ;
#31232=CARTESIAN_POINT ( 'NONE',  ( 18.00000000000000000, 5.196152422706630247, -6.318749998770966769 ) ) ;
#31233=CARTESIAN_POINT ( 'NONE',  ( 33.93698784468253393, -5.407089921784861808, 162.0519838440392562 ) ) ;
#31235=CARTESIAN_POINT ( 'NONE',  ( 37.06326651802246630, 7.347880794884125653E-16, 164.7616969801814548 ) ) ;
#31239=EDGE_CURVE ( 'NONE', #10799, #14365, #27465, .T. ) ;
#31243=CARTESIAN_POINT ( 'NONE',  ( 37.01584409946383403, -3.604726614523235284, 161.4250080079952170 ) ) ;
#31256=CARTESIAN_POINT ( 'NONE',  ( 30.84832656884210067, 7.209453229046475009, 162.5668877765479863 ) ) ;
#31257=CARTESIAN_POINT ( 'NONE',  ( 15.24356964374999990, 0.000000000000000000, -4.190624999385467397 ) ) ;
#31259=CARTESIAN_POINT ( 'NONE',  ( 31.31406506914986920, 7.209453229046482114, 167.8903031944757629 ) ) ;
#31260=CARTESIAN_POINT ( 'NONE',  ( 37.18092677073180141, 7.347880794884125653E-16, 166.1065598226053055 ) ) ;
#31263=CARTESIAN_POINT ( 'NONE',  ( 36.99789971106840625, 3.464101615138000856, 164.0145509578370024 ) ) ;
#31267=ORIENTED_EDGE ( 'NONE', *, *, #17592, .F. ) ;
#31271=CARTESIAN_POINT ( 'NONE',  ( 26.75643035624999655, 7.049594010296217766E-16, -6.215624999385465976 ) ) ;
#31274=CARTESIAN_POINT ( 'NONE',  ( 23.87821517812500005, -4.985214923628404016, -1.453124999385491112 ) ) ;
#31296=CARTESIAN_POINT ( 'NONE',  ( 25.48152094116770883, 0.000000000000000000, 170.0662982274954800 ) ) ;
#31300=DIRECTION ( 'NONE',  ( 0.9961946980917462113, 0.000000000000000000, -0.08715574274765118534 ) ) ;
#31305=CARTESIAN_POINT ( 'NONE',  ( 26.99999999999999645, 7.347880794884117764E-16, -9.225000000000010303 ) ) ;
#31310=CARTESIAN_POINT ( 'NONE',  ( 18.12178482187499640, 4.985214923628404904, -7.528124999385488181 ) ) ;
#31315=CARTESIAN_POINT ( 'NONE',  ( 31.31406506914986920, 7.209453229046482114, 167.8903031944757629 ) ) ;
#31320=CARTESIAN_POINT ( 'NONE',  ( 20.99999999999999645, -6.928203230275506996, -7.537500000000000533 ) ) ;
#31324=CARTESIAN_POINT ( 'NONE',  ( 26.97716818855048260, 0.000000000000000000, 49.47706554351410801 ) ) ;
#31325=CARTESIAN_POINT ( 'NONE',  ( 15.00000000000054712, 3.464101615138070134, -1.331249998770982046 ) ) ;
#31332=VERTEX_POINT ( 'NONE', #17607 ) ;
#31338=DIRECTION ( 'NONE',  ( 0.000000000000000000, 0.000000000000000000, 1.000000000000000000 ) ) ;
#31349=CARTESIAN_POINT ( 'NONE',  ( 30.80910648460565682, 7.209453229046475009, 162.1186001624066932 ) ) ;
#31350=LINE ( 'NONE', #16771, #24440 ) ;
#31352=ADVANCED_FACE ( 'NONE', ( #11899 ), #3178, .T. ) ;
#31354=ORIENTED_EDGE ( 'NONE', *, *, #13538, .F. ) ;
#31356=CARTESIAN_POINT ( 'NONE',  ( 23.99999999999999645, 5.196152422706631135, -5.943749998770952558 ) ) ;
#31357=CARTESIAN_POINT ( 'NONE',  ( 20.99999999999999645, -6.646953231504538984, -3.628124999385488714 ) ) ;
#31358=CARTESIAN_POINT ( 'NONE',  ( 15.00000000000000000, 0.000000000000000000, -6.299999999999999822 ) ) ;
#31360=CARTESIAN_POINT ( 'NONE',  ( 31.39005398230441912, -6.928203230275514990, 168.7588604462623039 ) ) ;
#31368=CARTESIAN_POINT ( 'NONE',  ( 28.08117253353866971, 5.196152422706630247, 165.3593121602424674 ) ) ;
#31372=EDGE_CURVE ( 'NONE', #17676, #17383, #32179, .T. ) ;
#31374=CARTESIAN_POINT ( 'NONE',  ( 26.75643035624999655, 7.049594010296217766E-16, -4.078124999385480010 ) ) ;
#31384=CARTESIAN_POINT ( 'NONE',  ( 15.02283181144952628, 7.347880794884122694E-16, 50.52293445648592751 ) ) ;
#31385=CARTESIAN_POINT ( 'NONE',  ( 27.69756682629397915, 5.407089921784862696, 162.3720029866663594 ) ) ;
#31394=VECTOR ( 'NONE', #27049, 1000.000000000000000 ) ;
#31400=CARTESIAN_POINT ( 'NONE',  ( 26.99999999999999645, -3.464101615137751278, -5.212499999999995914 ) ) ;
#31402=CARTESIAN_POINT ( 'NONE',  ( 24.40136593803570975, -3.604726614523244610, 160.5147182943441067 ) ) ;
#31404=CARTESIAN_POINT ( 'NONE',  ( 37.56492527877403376, -3.604726614523235284, 167.7010346059732342 ) ) ;
#31406=DIRECTION ( 'NONE',  ( 0.08715574274765150453, 0.000000000000000000, 0.9961946980917461003 ) ) ;
#31414=CARTESIAN_POINT ( 'NONE',  ( 15.24356964374999990, 0.000000000000000000, -8.803124999385486760 ) ) ;
#31418=CARTESIAN_POINT ( 'NONE',  ( 27.73678691053042300, 5.407089921784862696, 162.8202906008076241 ) ) ;
#31429=CARTESIAN_POINT ( 'NONE',  ( 37.63846293671737442, -3.604726614523238837, 168.5415738824881373 ) ) ;
#31430=CARTESIAN_POINT ( 'NONE',  ( 21.00000000000000000, -6.928203230275506996, -0.7312499987709595306 ) ) ;
#31439=CARTESIAN_POINT ( 'NONE',  ( 24.56314878551104286, -3.604726614523240613, 162.3639047026769049 ) ) ;
#31440=CARTESIAN_POINT ( 'NONE',  ( 21.00000000000000000, 6.646953231504538984, -8.803124999385454785 ) ) ;
#31442=CARTESIAN_POINT ( 'NONE',  ( 31.37289519550453321, -7.209453229046482114, 168.5627346156876740 ) ) ;
#31443=CARTESIAN_POINT ( 'NONE',  ( 34.18580599575048495, -5.196152422706635576, 166.2933124484913492 ) ) ;
#31456=CARTESIAN_POINT ( 'NONE',  ( 15.24356964375000167, -3.323476615752272600, -1.565624999385462957 ) ) ;
#31462=AXIS2_PLACEMENT_3D ( 'NONE', #802, #4028, #15415 ) ;
#31467=FACE_OUTER_BOUND ( 'NONE', #24423, .T. ) ;
#31471=CARTESIAN_POINT ( 'NONE',  ( 33.92433876750752830, 5.196152422706637353, 163.3047283542161381 ) ) ;
#31477=CARTESIAN_POINT ( 'NONE',  ( 37.60741370336351252, 7.646167579472015790E-16, 168.1866795212929446 ) ) ;
#31479=CARTESIAN_POINT ( 'NONE',  ( 15.24356964374999990, 3.323476615752268604, -1.078124999385470462 ) ) ;
#31480=CARTESIAN_POINT ( 'NONE',  ( 18.00000000000000000, 5.196152422706630247, -5.025000000000002132 ) ) ;
#31487=CARTESIAN_POINT ( 'NONE',  ( 26.99999999999999645, 3.464101615137755275, -9.187499999999994671 ) ) ;
#31493=CARTESIAN_POINT ( 'NONE',  ( 15.24356964374999990, 3.323476615752268604, -0.1781249993854788494 ) ) ;
#31499=CARTESIAN_POINT ( 'NONE',  ( 37.33123894353190764, 3.604726614523243278, 165.0299875717147415 ) ) ;
#31501=CARTESIAN_POINT ( 'NONE',  ( 24.73633934067528983, 0.000000000000000000, 161.5488335588110544 ) ) ;
#31506=CARTESIAN_POINT ( 'NONE',  ( 25.11222996482124259, -3.604726614523240613, 168.6399313006548653 ) ) ;
#31507=EDGE_LOOP ( 'NONE', ( #36308, #34752, #624, #1702 ) ) ;
#31512=( BOUNDED_CURVE ( )  B_SPLINE_CURVE ( 2, ( #23246, #35538, #9020, #9583, #35158, #20779, #32695 ),
 .UNSPECIFIED., .F., .F. ) 
 B_SPLINE_CURVE_WITH_KNOTS ( ( 3, 2, 2, 3 ),
 ( 0.6086956521739130821, 0.6159420289855073172, 0.6231884057971016633, 0.6304347826086960094 ),
 .UNSPECIFIED. ) 
 CURVE ( )  GEOMETRIC_REPRESENTATION_ITEM ( )  RATIONAL_B_SPLINE_CURVE ( ( 1.000000000000000000, 0.8660254037844387076, 1.000000000000000000, 0.8660254037844387076, 1.000000000000000000, 0.8660254037844326014, 1.000000000000006217 ) ) 
 REPRESENTATION_ITEM ( '' )  );
#31520=CARTESIAN_POINT ( 'NONE',  ( 20.99999999999999645, 6.928203230275506996, -4.106249998770976184 ) ) ;
#31522=CARTESIAN_POINT ( 'NONE',  ( 25.33771396574129042, -3.464101615137802348, 168.4225769768684131 ) ) ;
#31529=CARTESIAN_POINT ( 'NONE',  ( 25.17756528844239483, 0.000000000000000000, 166.5920692191248804 ) ) ;
#31534=CARTESIAN_POINT ( 'NONE',  ( 36.94067227134398479, 7.646167579472015790E-16, 160.5657900808910767 ) ) ;
#31535=CARTESIAN_POINT ( 'NONE',  ( 23.87821517812500005, -4.985214923628404016, -1.003124999385485161 ) ) ;
#31540=VERTEX_POINT ( 'NONE', #15885 ) ;
#31541=CARTESIAN_POINT ( 'NONE',  ( 26.99999999999999645, -3.464101615137751278, -7.406249998770965348 ) ) ;
#31542=CARTESIAN_POINT ( 'NONE',  ( 15.24356964374999990, 0.000000000000000000, -2.840624999385477079 ) ) ;
#31543=CARTESIAN_POINT ( 'NONE',  ( 36.56321044411491528, 7.347880794884117764E-16, 159.0460299011043901 ) ) ;
#31551=CARTESIAN_POINT ( 'NONE',  ( 25.06317337608610174, -3.464101615137757051, 165.2845636778794471 ) ) ;
#31555=CARTESIAN_POINT ( 'NONE',  ( 15.24356964375000167, -3.323476615752272600, -3.815624999385473615 ) ) ;
#31565=CARTESIAN_POINT ( 'NONE',  ( 27.71064018770612947, -5.407089921784865361, 162.5214321913800859 ) ) ;
#31577=ORIENTED_EDGE ( 'NONE', *, *, #31954, .F. ) ;
#31578=CARTESIAN_POINT ( 'NONE',  ( 24.00000000000000000, -5.196152422706629359, -4.349999999999992539 ) ) ;
#31579=( BOUNDED_SURFACE ( )  B_SPLINE_SURFACE ( 1, 2, ( 
 ( #17675, #2691, #23544, #2874, #11229, #23354, #11786, #29212, #3253, #14448, #14267, #14827, #28470, #8574, #35089, #20523, #14080, #8394, #34535, #37365, #11417, #32248, #9139, #25818, #5907, #20705, #16928, #26184, #31877, #20143, #32, #31689, #11597, #37186, #5718, #31506, #23172, #17299, #8761, #34906, #19963, #20335, #17487, #29020, #3065, #32063, #4006, #35656, #21089, #33007, #7057, #18434, #35465, #15202, #15580, #6288, #12733, #20896, #32438, #782, #21646, #1350, #6482, #32815, #36031, #10075, #27134, #21279, #12351, #3816, #18054, #29785, #12922, #26751, #29596, #971, #9516, #23924, #1161, #15009, #18628, #9702, #32629, #6858, #3633, #24300, #29975, #6666, #30168, #4195, #35843, #18241, #15393, #9885, #17864, #21467, #26941, #12547, #15772, #27322, #23732, #24113, #24485, #29409, #3440, #26561, #589, #12158, #35271, #9326, #9997, #1120, #15158, #930, #35235, #9659, #24442, #9472, #12504, #4338, #7202, #21607, #23883, #24068, #18386, #27277, #9285, #32585, #6438, #21047, #3964, #18774, #15348, #35614, #6811, #21236, #29936, #3774, #15727, #20859, #27096, #15538, #12686, #18201, #12116, #6625, #29741, #24258, #26902, #35801, #30125, #33156, #32775, #30314, #9844, #32398, #12309, #21422, #3594, #32963, #7014, #18583, #1306, #18011, #26707, #738, #12874, #4157, #35991, #10026, #15918, #550, #35422, #23689, #29555, #13633, #2240, #13068, #36546, #36172, #27837, #30693, #13819, #21792, #34082, #4529, #8133, #27656, #7382, #1493, #7752, #10961, #25183, #10218, #24806, #36913, #19703, #19334, #10406, #31243, #16664, #5272, #13257, #33345, #2056, #27467, #33526, #10588, #1868, #30509, #18954, #36358, #28023, #16105, #13438, #24624, #22167, #25366, #21980, #24988, #1682, #7568, #22535, #19143, #33711, #30873, #28210, #4710, #16290, #4896, #16477, #36736, #10775, #22349, #33898, #7940, #19516, #31062, #5086, #31984, #13999, #5828, #34634, #20251, #34455, #28389, #11338, #25738, #17407, #37290, #2985, #8864, #11889, #22909, #35011, #31791, #11152, #28571, #2798, #19887, #28948, #8497, #14554, #6012, #22725, #5450, #17033, #17596, #28759, #20065, #26107 ),
 ( #25926, #25551, #17221, #31610, #3169, #34271, #23457, #31429, #9054, #20625, #29127, #11520, #37103, #8680, #37469, #5636, #8316, #32167, #23090, #140, #2610, #11703, #23278, #14186, #14370, #34821, #20441, #14742, #26289, #324, #16852, #2426, #18157, #12830, #32540, #32731, #18343, #23650, #6395, #15305, #26857, #6582, #29890, #21566, #24397, #24210, #15494, #12075, #3552, #26475, #29698, #15114, #3921, #20814, #6768, #23837, #35944, #4113, #886, #3732, #3359, #27050, #6971, #12458, #18539, #508, #12646, #1076, #35193, #24027, #35572, #17968, #9617, #29320, #9241, #29511, #35378, #35756, #32356, #9428, #26665, #14929, #695, #21192, #6205, #12267, #21379, #17777, #30078, #21006, #15685, #9800, #32917, #27236, #1260, #9985, #33111, #16620, #22122, #21749, #36501, #7340, #13395, #1642, #22305, #33300, #5040, #7525, #27418, #2010, #16433, #7898, #19472, #19100, #30465, #31018, #7155, #24763, #28164, #36692, #30270, #24581, #13213, #16063, #27610, #10917, #2194, #18913, #33670, #25323, #36872, #30831, #10545, #36313, #30650, #4484, #4666, #13775, #10362, #10174, #27798, #21935, #33482, #4854, #4296, #18729, #24945, #16249, #1825, #15873, #7710, #19292, #27980, #33857, #1449, #13584, #25138, #10732, #13025, #36133, #28901, #37060, #11107, #16985, #34591, #17545, #11294, #25507, #11475, #5966, #22681, #2384, #34040, #2753, #29081, #20202, #5227, #19842, #31934, #3123, #14324, #5405, #14691, #11653, #276, #8269, #31202, #8634, #26241, #28527, #31565, #34412, #34226, #16805, #31385, #23046, #2569, #22863, #19659, #5588, #8820, #14140, #8451, #22493, #8085, #28347, #25694, #20019, #25878, #23229, #13957, #37245, #17175, #28716, #37426, #31751, #5781, #17359, #2936, #14506, #26061, #91, #34777, #20393, #838, #29652, #15255, #29462, #23411, #6348, #20762, #12406, #32307, #35523, #3873, #6917, #17918, #30028, #26808, #6154, #23598, #35327, #14881, #23979, #3497, #9567, #1024, #17728, #461, #12030, #12596, #23788, #15067, #21142, #9381, #32680, #35142, #26617, #646, #6723, #24161, #34961, #20957, #20575, #12217, #32488, #35705, #29270, #18488, #26427, #4060 ) ),
 .UNSPECIFIED., .F., .F., .F. ) 
 B_SPLINE_SURFACE_WITH_KNOTS ( ( 2, 2 ),
 ( 3, 2, 2, 2, 2, 2, 2, 2, 2, 2, 2, 2, 2, 2, 2, 2, 2, 2, 2, 2, 2, 2, 2, 2, 2, 2, 2, 2, 2, 2, 2, 2, 2, 2, 2, 2, 2, 2, 2, 2, 2, 2, 2, 2, 2, 2, 2, 2, 2, 2, 2, 2, 2, 2, 2, 2, 2, 2, 2, 2, 2, 2, 2, 2, 2, 2, 2, 2, 2, 2, 2, 2, 2, 2, 2, 2, 2, 2, 2, 2, 2, 2, 2, 2, 2, 2, 2, 2, 2, 2, 2, 2, 2, 2, 2, 2, 2, 2, 2, 2, 2, 2, 2, 2, 2, 2, 2, 2, 2, 2, 2, 2, 2, 2, 2, 2, 2, 2, 2, 2, 2, 2, 2, 2, 2, 2, 2, 2, 2, 2, 2, 2, 2, 2, 2, 3 ),
 ( 0.000000000000000000, 1.000000000000000000 ),
 ( 0.000000000000000000, 0.007246376811594202987, 0.01449275362318840597, 0.02173913043478260809, 0.02898550724637681195, 0.03623188405797101580, 0.04347826086956521618, 0.05072463768115942351, 0.05797101449275362389, 0.06521739130434782428, 0.07246376811594203160, 0.07971014492753622505, 0.08695652173913043237, 0.09420289855072463969, 0.1014492753623188470, 0.1086956521739130405, 0.1159420289855072478, 0.1231884057971014551, 0.1304347826086956486, 0.1376811594202898559, 0.1449275362318840632, 0.1521739130434782705, 0.1594202898550724501, 0.1666666666666666574, 0.1739130434782608647, 0.1811594202898550721, 0.1884057971014492794, 0.1956521739130434867, 0.2028985507246376940, 0.2101449275362318736, 0.2173913043478260809, 0.2246376811594202882, 0.2318840579710144956, 0.2391304347826087029, 0.2463768115942029102, 0.2536231884057971175, 0.2608695652173912971, 0.2681159420289855322, 0.2753623188405797118, 0.2826086956521738913, 0.2898550724637681264, 0.2971014492753623060, 0.3043478260869565410, 0.3115942028985507206, 0.3188405797101449002, 0.3260869565217391353, 0.3333333333333333148, 0.3405797101449275499, 0.3478260869565217295, 0.3550724637681159646, 0.3623188405797101441, 0.3695652173913043237, 0.3768115942028985588, 0.3840579710144927383, 0.3913043478260869734, 0.3985507246376811530, 0.4057971014492753881, 0.4130434782608695676, 0.4202898550724637472, 0.4275362318840579823, 0.4347826086956521618, 0.4420289855072463969, 0.4492753623188405765, 0.4565217391304347561, 0.4637681159420289911, 0.4710144927536231707, 0.4782608695652174058, 0.4855072463768115854, 0.4927536231884058204, 0.5000000000000000000, 0.5072463768115942351, 0.5144927536231883591, 0.5217391304347825942, 0.5289855072463768293, 0.5362318840579710644, 0.5434782608695651884, 0.5507246376811594235, 0.5579710144927536586, 0.5652173913043477826, 0.5724637681159420177, 0.5797101449275362528, 0.5869565217391304879, 0.5942028985507246119, 0.6014492753623188470, 0.6086956521739130821, 0.6159420289855072062, 0.6231884057971014412, 0.6304347826086956763, 0.6376811594202898004, 0.6449275362318840354, 0.6521739130434782705, 0.6594202898550725056, 0.6666666666666666297, 0.6739130434782608647, 0.6811594202898550998, 0.6884057971014492239, 0.6956521739130434590, 0.7028985507246376940, 0.7101449275362319291, 0.7173913043478260532, 0.7246376811594202882, 0.7318840579710145233, 0.7391304347826086474, 0.7463768115942028825, 0.7536231884057971175, 0.7608695652173913526, 0.7681159420289854767, 0.7753623188405797118, 0.7826086956521739468, 0.7898550724637680709, 0.7971014492753623060, 0.8043478260869565410, 0.8115942028985507761, 0.8188405797101449002, 0.8260869565217391353, 0.8333333333333333703, 0.8405797101449274944, 0.8478260869565217295, 0.8550724637681159646, 0.8623188405797101996, 0.8695652173913043237, 0.8768115942028985588, 0.8840579710144927938, 0.8913043478260869179, 0.8985507246376811530, 0.9057971014492753881, 0.9130434782608695121, 0.9202898550724637472, 0.9275362318840579823, 0.9347826086956522174, 0.9420289855072463414, 0.9492753623188405765, 0.9565217391304348116, 0.9637681159420289356, 0.9662082893573751274, 0.9758703722509488587 ),
 .UNSPECIFIED. ) 
 GEOMETRIC_REPRESENTATION_ITEM ( )  RATIONAL_B_SPLINE_SURFACE ( (
 ( 1.000000000000000000, 0.8660254037844387076, 1.000000000000000000, 0.8660254037844387076, 1.000000000000000000, 0.8660254037844387076, 1.000000000000000000, 0.8660254037844387076, 1.000000000000000000, 0.8660254037844387076, 1.000000000000000000, 0.8660254037844387076, 1.000000000000000000, 0.8660254037844387076, 1.000000000000000000, 0.8660254037844387076, 1.000000000000000000, 0.8660254037844387076, 1.000000000000000000, 0.8660254037844387076, 1.000000000000000000, 0.8660254037844387076, 1.000000000000000000, 0.8660254037844387076, 1.000000000000000000, 0.8660254037844387076, 1.000000000000000000, 0.8660254037844387076, 1.000000000000000000, 0.8660254037844387076, 1.000000000000000000, 0.8660254037844387076, 1.000000000000000000, 0.8660254037844387076, 1.000000000000000000, 0.8660254037844387076, 1.000000000000000000, 0.8660254037844387076, 1.000000000000000000, 0.8660254037844387076, 1.000000000000000000, 0.8660254037844387076, 1.000000000000000000, 0.8660254037844387076, 1.000000000000000000, 0.8660254037844387076, 1.000000000000000000, 0.8660254037844387076, 1.000000000000000000, 0.8660254037844387076, 1.000000000000000000, 0.8660254037844387076, 1.000000000000000000, 0.8660254037844387076, 1.000000000000000000, 0.8660254037844387076, 1.000000000000000000, 0.8660254037844387076, 1.000000000000000000, 0.8660254037844387076, 1.000000000000000000, 0.8660254037844387076, 1.000000000000000000, 0.8660254037844387076, 1.000000000000000000, 0.8660254037844387076, 1.000000000000000000, 0.8660254037844387076, 1.000000000000000000, 0.8660254037844387076, 1.000000000000000000, 0.8660254037844387076, 1.000000000000000000, 0.8660254037844387076, 1.000000000000000000, 0.8660254037844387076, 1.000000000000000000, 0.8660254037844387076, 1.000000000000000000, 0.8660254037844387076, 1.000000000000000000, 0.8660254037844387076, 1.000000000000000000, 0.8660254037844387076, 1.000000000000000000, 0.8660254037844387076, 1.000000000000000000, 0.8660254037844387076, 1.000000000000000000, 0.8660254037844387076, 1.000000000000000000, 0.8660254037844387076, 1.000000000000000000, 0.8660254037844387076, 1.000000000000000000, 0.8660254037844387076, 1.000000000000000000, 0.8660254037844387076, 1.000000000000000000, 0.8660254037844387076, 1.000000000000000000, 0.8660254037844387076, 1.000000000000000000, 0.8660254037844387076, 1.000000000000000000, 0.8660254037844387076, 1.000000000000000000, 0.8660254037844387076, 1.000000000000000000, 0.8660254037844387076, 1.000000000000000000, 0.8660254037844387076, 1.000000000000000000, 0.8660254037844387076, 1.000000000000000000, 0.8660254037844387076, 1.000000000000000000, 0.8660254037844387076, 1.000000000000000000, 0.8660254037844387076, 1.000000000000000000, 0.8660254037844387076, 1.000000000000000000, 0.8660254037844387076, 1.000000000000000000, 0.8660254037844387076, 1.000000000000000000, 0.8660254037844387076, 1.000000000000000000, 0.8660254037844387076, 1.000000000000000000, 0.8660254037844387076, 1.000000000000000000, 0.8660254037844387076, 1.000000000000000000, 0.8660254037844387076, 1.000000000000000000, 0.8660254037844387076, 1.000000000000000000, 0.8660254037844387076, 1.000000000000000000, 0.8660254037844387076, 1.000000000000000000, 0.8660254037844387076, 1.000000000000000000, 0.8660254037844387076, 1.000000000000000000, 0.8660254037844387076, 1.000000000000000000, 0.8660254037844387076, 1.000000000000000000, 0.8660254037844387076, 1.000000000000000000, 0.8660254037844387076, 1.000000000000000000, 0.8660254037844387076, 1.000000000000000000, 0.8660254037844387076, 1.000000000000000000, 0.8660254037844387076, 1.000000000000000000, 0.8660254037844387076, 1.000000000000000000, 0.8660254037844387076, 1.000000000000000000, 0.8660254037844387076, 1.000000000000000000, 0.8660254037844387076, 1.000000000000000000, 0.8660254037844387076, 1.000000000000000000, 0.8660254037844387076, 1.000000000000000000, 0.8660254037844387076, 1.000000000000000000, 0.8660254037844387076, 1.000000000000000000, 0.8660254037844387076, 1.000000000000000000, 0.8660254037844387076, 1.000000000000000000, 0.8660254037844387076, 1.000000000000000000, 0.8660254037844387076, 1.000000000000000000, 0.8660254037844387076, 1.000000000000000000, 0.8660254037844387076, 1.000000000000000000, 0.8660254037844387076, 1.000000000000000000, 0.8660254037844387076, 1.000000000000000000, 0.8660254037844387076, 1.000000000000000000, 0.8660254037844387076, 1.000000000000000000, 0.8660254037844387076, 1.000000000000000000, 0.8660254037844387076, 1.000000000000000000, 0.8660254037844387076, 1.000000000000000000, 0.8660254037844387076, 1.000000000000000000, 0.8660254037844387076, 1.000000000000000000, 0.8660254037844387076, 1.000000000000000000, 0.8660254037844387076, 1.000000000000000000, 0.8660254037844387076, 1.000000000000000000, 0.8660254037844387076, 1.000000000000000000, 0.8660254037844387076, 1.000000000000000000, 0.8660254037844387076, 1.000000000000000000, 0.8660254037844387076, 1.000000000000000000, 0.8660254037844387076, 1.000000000000000000, 0.8660254037844387076, 1.000000000000000000, 0.8660254037844387076, 1.000000000000000000, 0.8660254037844387076, 1.000000000000000000, 0.8660254037844387076, 1.000000000000000000, 0.8660254037844387076, 1.000000000000000000, 0.8660254037844387076, 1.000000000000000000, 0.8660254037844387076, 1.000000000000000000, 0.8660254037844387076, 1.000000000000000000, 0.8660254037844387076, 1.000000000000000000, 0.8660254037844387076, 1.000000000000000000, 0.8660254037844387076, 1.000000000000000000, 0.8660254037844387076, 1.000000000000000000, 0.8660254037844387076, 1.000000000000000000, 0.8660254037844387076, 1.000000000000000000, 0.8660254037844387076, 1.000000000000000000, 0.8660254037844387076, 1.000000000000000000, 0.8660254037844387076, 1.000000000000000000, 0.8660254037844387076, 1.000000000000000000, 0.8660254037844387076, 1.000000000000000000, 0.8660254037844387076, 1.000000000000000000, 0.8660254037844387076, 1.000000000000000000, 0.8660254037844387076, 1.000000000000000000, 0.9548848677736607726, 0.9401542295229587953, 0.9401542295229587953, 0.9401542295229587953),
 ( 1.000000000000000000, 0.8660254037844387076, 1.000000000000000000, 0.8660254037844387076, 1.000000000000000000, 0.8660254037844387076, 1.000000000000000000, 0.8660254037844387076, 1.000000000000000000, 0.8660254037844387076, 1.000000000000000000, 0.8660254037844387076, 1.000000000000000000, 0.8660254037844387076, 1.000000000000000000, 0.8660254037844387076, 1.000000000000000000, 0.8660254037844387076, 1.000000000000000000, 0.8660254037844387076, 1.000000000000000000, 0.8660254037844387076, 1.000000000000000000, 0.8660254037844387076, 1.000000000000000000, 0.8660254037844387076, 1.000000000000000000, 0.8660254037844387076, 1.000000000000000000, 0.8660254037844387076, 1.000000000000000000, 0.8660254037844387076, 1.000000000000000000, 0.8660254037844387076, 1.000000000000000000, 0.8660254037844387076, 1.000000000000000000, 0.8660254037844387076, 1.000000000000000000, 0.8660254037844387076, 1.000000000000000000, 0.8660254037844387076, 1.000000000000000000, 0.8660254037844387076, 1.000000000000000000, 0.8660254037844387076, 1.000000000000000000, 0.8660254037844387076, 1.000000000000000000, 0.8660254037844387076, 1.000000000000000000, 0.8660254037844387076, 1.000000000000000000, 0.8660254037844387076, 1.000000000000000000, 0.8660254037844387076, 1.000000000000000000, 0.8660254037844387076, 1.000000000000000000, 0.8660254037844387076, 1.000000000000000000, 0.8660254037844387076, 1.000000000000000000, 0.8660254037844387076, 1.000000000000000000, 0.8660254037844387076, 1.000000000000000000, 0.8660254037844387076, 1.000000000000000000, 0.8660254037844387076, 1.000000000000000000, 0.8660254037844387076, 1.000000000000000000, 0.8660254037844387076, 1.000000000000000000, 0.8660254037844387076, 1.000000000000000000, 0.8660254037844387076, 1.000000000000000000, 0.8660254037844387076, 1.000000000000000000, 0.8660254037844387076, 1.000000000000000000, 0.8660254037844387076, 1.000000000000000000, 0.8660254037844387076, 1.000000000000000000, 0.8660254037844387076, 1.000000000000000000, 0.8660254037844387076, 1.000000000000000000, 0.8660254037844387076, 1.000000000000000000, 0.8660254037844387076, 1.000000000000000000, 0.8660254037844387076, 1.000000000000000000, 0.8660254037844387076, 1.000000000000000000, 0.8660254037844387076, 1.000000000000000000, 0.8660254037844387076, 1.000000000000000000, 0.8660254037844387076, 1.000000000000000000, 0.8660254037844387076, 1.000000000000000000, 0.8660254037844387076, 1.000000000000000000, 0.8660254037844387076, 1.000000000000000000, 0.8660254037844387076, 1.000000000000000000, 0.8660254037844387076, 1.000000000000000000, 0.8660254037844387076, 1.000000000000000000, 0.8660254037844387076, 1.000000000000000000, 0.8660254037844387076, 1.000000000000000000, 0.8660254037844387076, 1.000000000000000000, 0.8660254037844387076, 1.000000000000000000, 0.8660254037844387076, 1.000000000000000000, 0.8660254037844387076, 1.000000000000000000, 0.8660254037844387076, 1.000000000000000000, 0.8660254037844387076, 1.000000000000000000, 0.8660254037844387076, 1.000000000000000000, 0.8660254037844387076, 1.000000000000000000, 0.8660254037844387076, 1.000000000000000000, 0.8660254037844387076, 1.000000000000000000, 0.8660254037844387076, 1.000000000000000000, 0.8660254037844387076, 1.000000000000000000, 0.8660254037844387076, 1.000000000000000000, 0.8660254037844387076, 1.000000000000000000, 0.8660254037844387076, 1.000000000000000000, 0.8660254037844387076, 1.000000000000000000, 0.8660254037844387076, 1.000000000000000000, 0.8660254037844387076, 1.000000000000000000, 0.8660254037844387076, 1.000000000000000000, 0.8660254037844387076, 1.000000000000000000, 0.8660254037844387076, 1.000000000000000000, 0.8660254037844387076, 1.000000000000000000, 0.8660254037844387076, 1.000000000000000000, 0.8660254037844387076, 1.000000000000000000, 0.8660254037844387076, 1.000000000000000000, 0.8660254037844387076, 1.000000000000000000, 0.8660254037844387076, 1.000000000000000000, 0.8660254037844387076, 1.000000000000000000, 0.8660254037844387076, 1.000000000000000000, 0.8660254037844387076, 1.000000000000000000, 0.8660254037844387076, 1.000000000000000000, 0.8660254037844387076, 1.000000000000000000, 0.8660254037844387076, 1.000000000000000000, 0.8660254037844387076, 1.000000000000000000, 0.8660254037844387076, 1.000000000000000000, 0.8660254037844387076, 1.000000000000000000, 0.8660254037844387076, 1.000000000000000000, 0.8660254037844387076, 1.000000000000000000, 0.8660254037844387076, 1.000000000000000000, 0.8660254037844387076, 1.000000000000000000, 0.8660254037844387076, 1.000000000000000000, 0.8660254037844387076, 1.000000000000000000, 0.8660254037844387076, 1.000000000000000000, 0.8660254037844387076, 1.000000000000000000, 0.8660254037844387076, 1.000000000000000000, 0.8660254037844387076, 1.000000000000000000, 0.8660254037844387076, 1.000000000000000000, 0.8660254037844387076, 1.000000000000000000, 0.8660254037844387076, 1.000000000000000000, 0.8660254037844387076, 1.000000000000000000, 0.8660254037844387076, 1.000000000000000000, 0.8660254037844387076, 1.000000000000000000, 0.8660254037844387076, 1.000000000000000000, 0.8660254037844387076, 1.000000000000000000, 0.8660254037844387076, 1.000000000000000000, 0.8660254037844387076, 1.000000000000000000, 0.8660254037844387076, 1.000000000000000000, 0.8660254037844387076, 1.000000000000000000, 0.8660254037844387076, 1.000000000000000000, 0.8660254037844387076, 1.000000000000000000, 0.8660254037844387076, 1.000000000000000000, 0.8660254037844387076, 1.000000000000000000, 0.8660254037844387076, 1.000000000000000000, 0.8660254037844387076, 1.000000000000000000, 0.8660254037844387076, 1.000000000000000000, 0.8660254037844387076, 1.000000000000000000, 0.8660254037844387076, 1.000000000000000000, 0.8660254037844387076, 1.000000000000000000, 0.8660254037844387076, 1.000000000000000000, 0.8660254037844387076, 1.000000000000000000, 0.8660254037844387076, 1.000000000000000000, 0.8660254037844387076, 1.000000000000000000, 0.8660254037844387076, 1.000000000000000000, 0.9548848677736607726, 0.9401542295229587953, 0.9401542295229587953, 0.9401542295229587953) ) ) 
 REPRESENTATION_ITEM ( '' )  SURFACE ( )  );
#31580=CARTESIAN_POINT ( 'NONE',  ( 25.17756528844239483, 0.000000000000000000, 166.5920692191248804 ) ) ;
#31581=CARTESIAN_POINT ( 'NONE',  ( 36.89981801693102170, 3.604726614523243278, 160.0988238161605750 ) ) ;
#31583=CARTESIAN_POINT ( 'NONE',  ( 24.61541074761292336, 3.464101615137757051, 160.1666134152087579 ) ) ;
#31589=CARTESIAN_POINT ( 'NONE',  ( 24.97492818644736445, -3.464101615137975543, 164.2759165448371732 ) ) ;
#31592=CARTESIAN_POINT ( 'NONE',  ( 25.46681340963260354, 0.000000000000000000, 169.8981903728046916 ) ) ;
#31594=CARTESIAN_POINT ( 'NONE',  ( 18.12178482187499640, 4.985214923628404904, -9.328124999385483562 ) ) ;
#31599=CARTESIAN_POINT ( 'NONE',  ( 36.93250142046140638, -3.604726614523238837, 160.4723968279450048 ) ) ;
#31610=CARTESIAN_POINT ( 'NONE',  ( 31.43172532185919721, 7.209453229046482114, 169.2351660368996420 ) ) ;
#31611=CARTESIAN_POINT ( 'NONE',  ( 23.99999999999999645, 5.196152422706631135, -2.793749998770966858 ) ) ;
#31620=CARTESIAN_POINT ( 'NONE',  ( 30.78949644248743667, -7.209453229046475009, 161.8944563553360183 ) ) ;
#31621=CARTESIAN_POINT ( 'NONE',  ( 18.12178482187499640, 4.985214923628404904, -6.515624999385460470 ) ) ;
#31623=CARTESIAN_POINT ( 'NONE',  ( 28.25972136701633630, -5.407089921784865361, 168.7974587893581315 ) ) ;
#31624=CARTESIAN_POINT ( 'NONE',  ( 28.11058759660888740, 5.196152422706636465, 165.6955278696240725 ) ) ;
#31625=CARTESIAN_POINT ( 'NONE',  ( 25.21678537267883868, 0.000000000000000000, 167.0403568332661450 ) ) ;
#31631=VERTEX_POINT ( 'NONE', #16633 ) ;
#31637=AXIS2_PLACEMENT_3D ( 'NONE', #17745, #29286, #3325 ) ;
#31639=CARTESIAN_POINT ( 'NONE',  ( 21.00000000000000000, 6.646953231504538984, -2.615624999385474325 ) ) ;
#31643=( BOUNDED_CURVE ( )  B_SPLINE_CURVE ( 2, ( #37485, #28774, #11536, #5287, #31808, #16867, #37119 ),
 .UNSPECIFIED., .F., .F. ) 
 B_SPLINE_CURVE_WITH_KNOTS ( ( 3, 2, 2, 3 ),
 ( 0.000000000000000000, 0.007246376811594299264, 0.01449275362318859853, 0.02173913043478289606 ),
 .UNSPECIFIED. ) 
 CURVE ( )  GEOMETRIC_REPRESENTATION_ITEM ( )  RATIONAL_B_SPLINE_CURVE ( ( 1.000000000000000000, 0.8660254037844387076, 1.000000000000000000, 0.8660254037844387076, 1.000000000000000000, 0.8660254037844333785, 1.000000000000005329 ) ) 
 REPRESENTATION_ITEM ( '' )  );
#31647=LINE ( 'NONE', #17255, #11561 ) ;
#31656=CARTESIAN_POINT ( 'NONE',  ( 18.00000000000000355, -5.196152422706632912, -2.568749998770964105 ) ) ;
#31660=CARTESIAN_POINT ( 'NONE',  ( 25.22662187717753568, 0.000000000000000000, 169.9474368419002985 ) ) ;
#31662=DIRECTION ( 'NONE',  ( 0.08715574274765150453, 0.000000000000000000, 0.9961946980917461003 ) ) ;
#31667=CARTESIAN_POINT ( 'NONE',  ( 15.00000000000000000, 0.000000000000000000, -3.093749998770961795 ) ) ;
#31668=DIRECTION ( 'NONE',  ( 0.8191520442889772546, 0.000000000000000000, -0.5735764363510669206 ) ) ;
#31672=ORIENTED_EDGE ( 'NONE', *, *, #34842, .F. ) ;
#31676=CARTESIAN_POINT ( 'NONE',  ( 23.87821517812499650, 4.985214923628404904, -0.2906249993854803648 ) ) ;
#31681=CARTESIAN_POINT ( 'NONE',  ( 24.87200694887302532, -3.604726614523244610, 165.8941696640395378 ) ) ;
#31686=CARTESIAN_POINT ( 'NONE',  ( 26.99999999999999289, 0.000000000000000000, 49.73803434254939759 ) ) ;
#31689=CARTESIAN_POINT ( 'NONE',  ( 37.56492527877403376, -3.604726614523235284, 167.7010346059732342 ) ) ;
#31690=ORIENTED_EDGE ( 'NONE', *, *, #33252, .F. ) ;
#31692=CARTESIAN_POINT ( 'NONE',  ( 31.29200377171331127, 6.928203230275514990, 167.6381414109090997 ) ) ;
#31697=EDGE_CURVE ( 'NONE', #19092, #12755, #13786, .T. ) ;
#31705=CARTESIAN_POINT ( 'NONE',  ( 36.86716609684025059, 7.347880794884125653E-16, 162.5202589094750181 ) ) ;
#31707=LINE ( 'NONE', #14463, #27336 ) ;
#31709=ADVANCED_FACE ( 'NONE', ( #25148 ), #31029, .T. ) ;
#31720=CARTESIAN_POINT ( 'NONE',  ( 33.78501001826630556, -5.407089921784855591, 160.3148693392417670 ) ) ;
#31721=CARTESIAN_POINT ( 'NONE',  ( 15.24356964375000167, -3.323476615752272600, -1.565624999385462957 ) ) ;
#31725=ORIENTED_EDGE ( 'NONE', *, *, #4364, .T. ) ;
#31727=CARTESIAN_POINT ( 'NONE',  ( 26.99999999999999645, 7.347880794884117764E-16, -6.468749998770951137 ) ) ;
#31728=CARTESIAN_POINT ( 'NONE',  ( 15.24356964374999990, 0.000000000000000000, -2.390624999385471128 ) ) ;
#31730=CARTESIAN_POINT ( 'NONE',  ( 26.97716818855048260, 0.000000000000000000, 49.47706554351410801 ) ) ;
#31737=CARTESIAN_POINT ( 'NONE',  ( 36.79526260918054703, -3.464101615137751278, 161.6983982847737025 ) ) ;
#31740=( BOUNDED_CURVE ( )  B_SPLINE_CURVE ( 2, ( #12503, #24067, #9658, #21235, #28022, #13998, #36545 ),
 .UNSPECIFIED., .F., .F. ) 
 B_SPLINE_CURVE_WITH_KNOTS ( ( 3, 2, 2, 3 ),
 ( 0.1304347826086947049, 0.1376811594202889955, 0.1449275362318833138, 0.1521739130434776044 ),
 .UNSPECIFIED. ) 
 CURVE ( )  GEOMETRIC_REPRESENTATION_ITEM ( )  RATIONAL_B_SPLINE_CURVE ( ( 1.000000000000017319, 0.8660254037844211661, 1.000000000000000000, 0.8660254037844387076, 1.000000000000000000, 0.8660254037844510311, 0.9999999999999876765 ) ) 
 REPRESENTATION_ITEM ( '' )  );
#31742=CARTESIAN_POINT ( 'NONE',  ( 20.99999999999999645, 6.646953231504538984, -4.865624999385484983 ) ) ;
#31751=CARTESIAN_POINT ( 'NONE',  ( 24.51902619074504130, -3.604726614523244610, 161.8595811367679573 ) ) ;
#31756=CARTESIAN_POINT ( 'NONE',  ( 28.38512818626399081, 5.196152422706636465, 168.8335411686130669 ) ) ;
#31763=CARTESIAN_POINT ( 'NONE',  ( 21.00000000000000000, -6.928203230275506996, -3.937500000000003109 ) ) ;
#31764=CARTESIAN_POINT ( 'NONE',  ( 30.66693367924855096, -7.209453229046482114, 160.4935575611445415 ) ) ;
#31766=CARTESIAN_POINT ( 'NONE',  ( 37.61068204371655099, 3.604726614523238837, 168.2240368224713620 ) ) ;
#31770=ORIENTED_EDGE ( 'NONE', *, *, #25170, .T. ) ;
#31771=CARTESIAN_POINT ( 'NONE',  ( 24.63175244948454434, -3.464101615137358703, 160.3533999223253943 ) ) ;
#31779=CARTESIAN_POINT ( 'NONE',  ( 24.39809759768267128, 0.000000000000000000, 160.4773609931656608 ) ) ;
#31784=CARTESIAN_POINT ( 'NONE',  ( 21.00000000000016342, 4.000000000000002665, 50.00000000000000000 ) ) ;
#31791=CARTESIAN_POINT ( 'NONE',  ( 30.61300606342344111, 7.209453229046475009, 159.8771620917002565 ) ) ;
#31792=CARTESIAN_POINT ( 'NONE',  ( 21.00000000000000000, 6.928203230275506996, -3.206249998770952292 ) ) ;
#31800=DIRECTION ( 'NONE',  ( 1.000000000000000000, 0.000000000000000000, 0.000000000000000000 ) ) ;
#31802=CARTESIAN_POINT ( 'NONE',  ( 37.05833252405330569, 7.646167579472015790E-16, 161.9106529233149274 ) ) ;
#31804=CARTESIAN_POINT ( 'NONE',  ( 15.24356964374999990, 0.000000000000000000, -6.890624999385474680 ) ) ;
#31806=CARTESIAN_POINT ( 'NONE',  ( 28.22050128277989245, -5.407089921784865361, 168.3491711752168385 ) ) ;
#31807=CARTESIAN_POINT ( 'NONE',  ( 37.06326651802246630, 7.347880794884125653E-16, 164.7616969801814548 ) ) ;
#31808=CARTESIAN_POINT ( 'NONE',  ( 23.99999999999999645, 5.196152422706631135, -0.1500000000000112355 ) ) ;
#31818=CARTESIAN_POINT ( 'NONE',  ( 15.00000000000000355, 7.347880794884112834E-16, -8.000000000000000000 ) ) ;
#31820=EDGE_CURVE ( 'NONE', #27666, #34054, #28357, .T. ) ;
#31821=CARTESIAN_POINT ( 'NONE',  ( 26.75643035624999655, 3.323476615752271712, -3.590624999385491734 ) ) ;
#31835=CARTESIAN_POINT ( 'NONE',  ( 27.71838675424445597, 5.196152422706636465, 161.2126517282112275 ) ) ;
#31839=DIRECTION ( 'NONE',  ( 0.08715574274765150453, 0.000000000000000000, 0.9961946980917461003 ) ) ;
#31845=CARTESIAN_POINT ( 'NONE',  ( 28.22540379330944660, -5.407089921784859143, 168.4052071269844930 ) ) ;
#31847=CARTESIAN_POINT ( 'NONE',  ( 21.00000000000000000, 6.646953231504538984, -1.153124999385464200 ) ) ;
#31861=CARTESIAN_POINT ( 'NONE',  ( 15.24356964374999990, 3.323476615752268604, -8.840624999385484628 ) ) ;
#31867=CARTESIAN_POINT ( 'NONE',  ( 25.06157068934916765, 3.604726614523240613, 168.0608931323890829 ) ) ;
#31872=AXIS2_PLACEMENT_3D ( 'NONE', #4480, #23688, #26148 ) ;
#31877=CARTESIAN_POINT ( 'NONE',  ( 34.46482481169798717, 5.407089921784857367, 168.0851879843573897 ) ) ;
#31878=ORIENTED_EDGE ( 'NONE', *, *, #10257, .T. ) ;
#31880=CARTESIAN_POINT ( 'NONE',  ( 34.27731952563551232, 5.196152422706637353, 167.3393168814877185 ) ) ;
#31886=ORIENTED_EDGE ( 'NONE', *, *, #27416, .T. ) ;
#31900=DIRECTION ( 'NONE',  ( 0.08715574274765150453, 0.000000000000000000, 0.9961946980917461003 ) ) ;
#31903=VERTEX_POINT ( 'NONE', #11664 ) ;
#31906=CARTESIAN_POINT ( 'NONE',  ( 36.86550044322413555, 3.604726614523238837, 159.7065721537869365 ) ) ;
#31907=CARTESIAN_POINT ( 'NONE',  ( 15.24356964375000167, -3.323476615752272600, -2.015624999385490668 ) ) ;
#31911=VERTEX_POINT ( 'NONE', #32315 ) ;
#31912=EDGE_LOOP ( 'NONE', ( #11067, #6325 ) ) ;
#31913=CARTESIAN_POINT ( 'NONE',  ( 20.99999999999999645, 6.646953231504538984, -4.753124999385462068 ) ) ;
#31921=CARTESIAN_POINT ( 'NONE',  ( 30.81155773992399460, -6.928203230275506996, 162.1466181389027099 ) ) ;
#31925=CARTESIAN_POINT ( 'NONE',  ( 23.87821517812500005, -4.985214923628404016, -3.253124999385486937 ) ) ;
#31934=CARTESIAN_POINT ( 'NONE',  ( 27.74986027194257332, -5.407089921784865361, 162.9697198055213789 ) ) ;
#31943=CARTESIAN_POINT ( 'NONE',  ( 26.99999999999952038, 3.464101615138031054, -3.731249998770935772 ) ) ;
#31947=CARTESIAN_POINT ( 'NONE',  ( 26.99999999999999645, -3.464101615137751278, -5.662499999999991651 ) ) ;
#31949=CARTESIAN_POINT ( 'NONE',  ( 20.99999999999999645, 0.000000000000000000, -8.000000000000000000 ) ) ;
#31950=CARTESIAN_POINT ( 'NONE',  ( 24.94224478302373527, 0.000000000000000000, 163.9023435342771506 ) ) ;
#31952=CARTESIAN_POINT ( 'NONE',  ( 28.09467017918796472, 5.407089921784856479, 166.9109150798468306 ) ) ;
#31954=EDGE_CURVE ( 'NONE', #26829, #1610, #15386, .T. ) ;
#31955=CARTESIAN_POINT ( 'NONE',  ( 25.33444562538816669, 0.000000000000000000, 168.3852196756899957 ) ) ;
#31960=CARTESIAN_POINT ( 'NONE',  ( 36.56321044411491528, 7.347880794884117764E-16, 159.0460299011043901 ) ) ;
#31962=CARTESIAN_POINT ( 'NONE',  ( 15.24356964375000167, -3.323476615752272600, -5.953124999385460470 ) ) ;
#31965=EDGE_CURVE ( 'NONE', #3146, #8675, #20479, .T. ) ;
#31971=CARTESIAN_POINT ( 'NONE',  ( 37.30839204460733782, 7.347880794884117764E-16, 167.5634945697888440 ) ) ;
#31979=VERTEX_POINT ( 'NONE', #20029 ) ;
#31984=CARTESIAN_POINT ( 'NONE',  ( 24.44548853280170775, -3.604726614523240613, 161.0190418602530258 ) ) ;
#31985=CARTESIAN_POINT ( 'NONE',  ( 15.00000000000000000, 3.464101615137752166, -1.781249998770938925 ) ) ;
#31993=VERTEX_POINT ( 'NONE', #14701 ) ;
#31994=CARTESIAN_POINT ( 'NONE',  ( 24.59583218904140978, 3.604726614523236616, 162.7374777144612494 ) ) ;
#31995=CARTESIAN_POINT ( 'NONE',  ( 23.87821517812499650, 4.985214923628404904, -8.390624999385476457 ) ) ;
#31997=CARTESIAN_POINT ( 'NONE',  ( 24.90469035240339934, 3.604726614523240613, 166.2677426758239108 ) ) ;
#31998=CARTESIAN_POINT ( 'NONE',  ( 33.92433876750752830, 5.196152422706637353, 163.3047283542161381 ) ) ;
#32003=VERTEX_POINT ( 'NONE', #20402 ) ;
#32008=CARTESIAN_POINT ( 'NONE',  ( 15.24356964374999990, 3.323476615752268604, -3.440624999385503813 ) ) ;
#32019=CARTESIAN_POINT ( 'NONE',  ( 20.99999999999999645, 6.928203230275506996, -7.256249998770945453 ) ) ;
#32026=CYLINDRICAL_SURFACE ( 'NONE', #27066, 3.999999999999996447 ) ;
#32031=CARTESIAN_POINT ( 'NONE',  ( 25.22662187717753568, 0.000000000000000000, 169.9474368419002985 ) ) ;
#32033=DIRECTION ( 'NONE',  ( 0.9961946980917462113, 0.000000000000000000, -0.08715574274765178209 ) ) ;
#32034=DIRECTION ( 'NONE',  ( 1.000000000000000000, 0.000000000000000000, 0.000000000000000000 ) ) ;
#32046=CARTESIAN_POINT ( 'NONE',  ( 18.12178482187499640, 4.985214923628404904, -10.22812499938549635 ) ) ;
#32054=CARTESIAN_POINT ( 'NONE',  ( 24.98966720158236043, -3.604726614523244610, 167.2390325064633885 ) ) ;
#32055=EDGE_CURVE ( 'NONE', #5932, #19565, #16836, .T. ) ;
#32062=CARTESIAN_POINT ( 'NONE',  ( 15.02283181144952628, 7.347880794884122694E-16, 50.52293445648592751 ) ) ;
#32063=CARTESIAN_POINT ( 'NONE',  ( 31.29935753756119965, -7.209453229046475009, 167.7221953391727709 ) ) ;
#32065=CARTESIAN_POINT ( 'NONE',  ( 37.29531868308838938, -3.464101615137579415, 167.4140653638507388 ) ) ;
#32091=CARTESIAN_POINT ( 'NONE',  ( 15.24356964375000167, -3.323476615752272600, -2.915624999385482141 ) ) ;
#32097=CARTESIAN_POINT ( 'NONE',  ( 15.24356964374999990, 3.323476615752268604, -6.028124999385455318 ) ) ;
#32104=CARTESIAN_POINT ( 'NONE',  ( 36.75604252494409963, -3.464101615137751278, 161.2501106706323810 ) ) ;
#32109=CARTESIAN_POINT ( 'NONE',  ( 26.75643035624999655, -3.323476615752267271, -5.465624999385501503 ) ) ;
#32112=EDGE_LOOP ( 'NONE', ( #18835, #29457, #25572, #1799 ) ) ;
#32113=CARTESIAN_POINT ( 'NONE',  ( 24.00000000000000000, -5.196152422706629359, -0.6937499987709483396 ) ) ;
#32117=FACE_OUTER_BOUND ( 'NONE', #29056, .T. ) ;
#32123=CARTESIAN_POINT ( 'NONE',  ( 15.00000000000000000, 0.000000000000000000, -4.049999999999998046 ) ) ;
#32130=ORIENTED_EDGE ( 'NONE', *, *, #21788, .F. ) ;
#32131=CARTESIAN_POINT ( 'NONE',  ( 26.99999999999999645, 7.347880794884117764E-16, -7.874999999999992895 ) ) ;
#32133=FACE_OUTER_BOUND ( 'NONE', #22094, .T. ) ;
#32135=CARTESIAN_POINT ( 'NONE',  ( 24.91286120328598841, 0.000000000000000000, 166.3611359287700395 ) ) ;
#32140=ORIENTED_EDGE ( 'NONE', *, *, #27204, .F. ) ;
#32141=DIRECTION ( 'NONE',  ( 0.000000000000000000, 0.000000000000000000, 1.000000000000000000 ) ) ;
#32142=FACE_OUTER_BOUND ( 'NONE', #4205, .T. ) ;
#32144=CARTESIAN_POINT ( 'NONE',  ( 18.12178482187500350, -4.985214923628407568, -5.465624999385465088 ) ) ;
#32147=CARTESIAN_POINT ( 'NONE',  ( 37.14497502684795904, 3.464101615138004409, 165.6956295096424583 ) ) ;
#32152=CARTESIAN_POINT ( 'NONE',  ( 30.58849351077567036, -7.209453229046482114, 159.5969823328619555 ) ) ;
#32165=CARTESIAN_POINT ( 'NONE',  ( 37.27244030072370151, 3.464101615137892942, 167.1525642568259968 ) ) ;
#32166=CARTESIAN_POINT ( 'NONE',  ( 22.38580703878232470, 5.599659159192138524, -8.000000000000000000 ) ) ;
#32167=CARTESIAN_POINT ( 'NONE',  ( 37.60577953318700395, 3.604726614523243278, 168.1680008707037075 ) ) ;
#32168=CARTESIAN_POINT ( 'NONE',  ( 26.99999999999999645, 3.464101615137755275, -1.931249998770958820 ) ) ;
#32179=LINE ( 'NONE', #3367, #30507 ) ;
#32181=CARTESIAN_POINT ( 'NONE',  ( 29.49486714975617474, 6.148716665048037378, 159.5363409456820136 ) ) ;
#32184=CARTESIAN_POINT ( 'NONE',  ( 26.75643035624999655, 3.323476615752271712, -6.628124999385471838 ) ) ;
#32185=CARTESIAN_POINT ( 'NONE',  ( 28.22824784931821895, 5.196152422706636465, 167.0403907120479232 ) ) ;
#32186=CARTESIAN_POINT ( 'NONE',  ( 24.91122703310947628, -3.604726614523244610, 166.3424572781808024 ) ) ;
#32187=CARTESIAN_POINT ( 'NONE',  ( 36.90965452142972225, 3.464101615137759271, 163.0059038247947285 ) ) ;
#32188=CARTESIAN_POINT ( 'NONE',  ( 20.99999999999999645, 0.000000000000000000, -8.000000000000000000 ) ) ;
#32198=CARTESIAN_POINT ( 'NONE',  ( 15.24356964374999990, 3.323476615752268604, -4.340624999385463312 ) ) ;
#32207=CARTESIAN_POINT ( 'NONE',  ( 24.90629303914081305, -3.464101615138032830, 163.4914132213142750 ) ) ;
#32212=CARTESIAN_POINT ( 'NONE',  ( 30.70370250816666058, 6.928203230275514990, 160.9138271987898463 ) ) ;
#32214=CARTESIAN_POINT ( 'NONE',  ( 26.99999999999999645, 7.347880794884117764E-16, -0.6750000000000089262 ) ) ;
#32215=DIRECTION ( 'NONE',  ( 0.9961946980917462113, 0.000000000000000000, -0.08715574274765118534 ) ) ;
#32216=CARTESIAN_POINT ( 'NONE',  ( 24.00000000000000000, -5.196152422706629359, -5.643749998770958065 ) ) ;
#32222=ORIENTED_EDGE ( 'NONE', *, *, #21463, .T. ) ;
#32223=CARTESIAN_POINT ( 'NONE',  ( 31.18169728485186454, -7.209453229046475009, 166.3773324967489202 ) ) ;
#32224=CARTESIAN_POINT ( 'NONE',  ( 18.12178482187499640, 4.985214923628404904, -1.565624999385478722 ) ) ;
#32229=CARTESIAN_POINT ( 'NONE',  ( 26.97716818855048260, 0.000000000000000000, 49.47706554351410801 ) ) ;
#32235=CARTESIAN_POINT ( 'NONE',  ( 18.12178482187500350, -4.985214923628407568, -8.278124999385488181 ) ) ;
#32238=EDGE_LOOP ( 'NONE', ( #6667, #11648, #19467, #2726 ) ) ;
#32240=EDGE_LOOP ( 'NONE', ( #6082, #8383, #22874, #288 ) ) ;
#32242=CARTESIAN_POINT ( 'NONE',  ( 34.25074851857407765, -5.407089921784861808, 165.6382847571695436 ) ) ;
#32248=CARTESIAN_POINT ( 'NONE',  ( 31.37779770603408380, -7.209453229046475009, 168.6187705674553285 ) ) ;
#32253=PRODUCT_DEFINITION_SHAPE ( 'NONE', 'NONE',  #7423 ) ;
#32257=VERTEX_POINT ( 'NONE', #845 ) ;
#32264=CARTESIAN_POINT ( 'NONE',  ( 21.00000000000000355, 0.000000000000000000, 50.00000000000001421 ) ) ;
#32265=CARTESIAN_POINT ( 'NONE',  ( 26.99999999999999289, 0.000000000000000000, -8.000000000000000000 ) ) ;
#32275=CARTESIAN_POINT ( 'NONE',  ( 36.86223210287109708, 7.646167579472015790E-16, 159.6692148526084907 ) ) ;
#32276=CARTESIAN_POINT ( 'NONE',  ( 15.24356964375000167, -3.323476615752272600, -3.365624999385478322 ) ) ;
#32282=CARTESIAN_POINT ( 'NONE',  ( 23.87821517812500005, -4.985214923628404016, -4.940624999385468286 ) ) ;
#32286=( BOUNDED_CURVE ( )  B_SPLINE_CURVE ( 2, ( #20660, #26143, #25770, #17441, #8899, #32207, #29358 ),
 .UNSPECIFIED., .F., .F. ) 
 B_SPLINE_CURVE_WITH_KNOTS ( ( 3, 2, 2, 3 ),
 ( 0.5869565217391293777, 0.5942028985507235017, 0.6014492753623178478, 0.6086956521739120829 ),
 .UNSPECIFIED. ) 
 CURVE ( )  GEOMETRIC_REPRESENTATION_ITEM ( )  RATIONAL_B_SPLINE_CURVE ( ( 1.000000000000020428, 0.8660254037844181685, 1.000000000000000000, 0.8660254037844387076, 1.000000000000000000, 0.8660254037844571373, 0.9999999999999815703 ) ) 
 REPRESENTATION_ITEM ( '' )  );
#32293=CARTESIAN_POINT ( 'NONE',  ( 27.89814547376861142, -5.196152422706632912, 163.2673032942497571 ) ) ;
#32296=AXIS2_PLACEMENT_3D ( 'NONE', #9586, #12427, #24368 ) ;
#32298=CARTESIAN_POINT ( 'NONE',  ( 18.12178482187500350, -4.985214923628407568, -6.928124999385470772 ) ) ;
#32299=CARTESIAN_POINT ( 'NONE',  ( 27.00000000000023448, 3.464101615137617163, -2.437499999999998224 ) ) ;
#32305=DIRECTION ( 'NONE',  ( 1.000000000000000000, 0.000000000000000000, 0.000000000000000000 ) ) ;
#32307=CARTESIAN_POINT ( 'NONE',  ( 33.79318086914889818, 5.407089921784862696, 160.4082625921878673 ) ) ;
#32315=CARTESIAN_POINT ( 'NONE',  ( 15.00000000000000000, 0.000000000000000000, -3.149999999999986144 ) ) ;
#32319=CARTESIAN_POINT ( 'NONE',  ( 15.00000000000000000, 3.464101615137752166, -5.887500000000005507 ) ) ;
#32324=CARTESIAN_POINT ( 'NONE',  ( 25.03052145599531997, 0.000000000000000000, 167.7059987711938902 ) ) ;
#32334=CARTESIAN_POINT ( 'NONE',  ( 23.87821517812500005, -4.985214923628404016, -6.740624999385463667 ) ) ;
#32341=CARTESIAN_POINT ( 'NONE',  ( 24.40136593803570975, -3.604726614523244610, 160.5147182943441067 ) ) ;
#32347=CARTESIAN_POINT ( 'NONE',  ( 26.75643035624999655, -3.323476615752267271, -0.5156249993854836733 ) ) ;
#32352=ORIENTED_EDGE ( 'NONE', *, *, #6458, .T. ) ;
#32355=CARTESIAN_POINT ( 'NONE',  ( 19.80074372294634344, 5.630122097104456991, -7.999999999999998224 ) ) ;
#32356=CARTESIAN_POINT ( 'NONE',  ( 37.40641077165175687, 7.646167579472024665E-16, 165.8892054988188534 ) ) ;
#32357=CARTESIAN_POINT ( 'NONE',  ( 18.00000000000000000, 5.196152422706630247, -3.168749998770953091 ) ) ;
#32367=CARTESIAN_POINT ( 'NONE',  ( 24.48144027668511669, 0.000000000000000000, 161.4299721732159014 ) ) ;
#32368=CARTESIAN_POINT ( 'NONE',  ( 26.75643035624999655, 3.323476615752271712, -9.778124999385472194 ) ) ;
#32370=CARTESIAN_POINT ( 'NONE',  ( 37.40314243129871841, -3.604726614523238837, 165.8518481976404360 ) ) ;
#32372=CARTESIAN_POINT ( 'NONE',  ( 24.93570810221054757, -3.464101615137761048, 163.8276289306958802 ) ) ;
#32373=CARTESIAN_POINT ( 'NONE',  ( 37.10248660225891371, 7.347880794884125653E-16, 165.2099845943227479 ) ) ;
#32383=CARTESIAN_POINT ( 'NONE',  ( 15.24356964374999990, 0.000000000000000000, -3.853124999385476812 ) ) ;
#32392=CARTESIAN_POINT ( 'NONE',  ( 36.86716609684025059, 7.347880794884125653E-16, 162.5202589094750181 ) ) ;
#32397=CARTESIAN_POINT ( 'NONE',  ( 26.99999999999999645, 7.347880794884117764E-16, -5.624999999999991118 ) ) ;
#32398=CARTESIAN_POINT ( 'NONE',  ( 24.72002912245681117, -3.604726614523240613, 164.1570551592420486 ) ) ;
#32410=CARTESIAN_POINT ( 'NONE',  ( 25.10896162446820412, 0.000000000000000000, 168.6025739994764479 ) ) ;
#32411=CARTESIAN_POINT ( 'NONE',  ( 26.75643035624999655, 7.049594010296217766E-16, -1.715624999385462202 ) ) ;
#32413=CARTESIAN_POINT ( 'NONE',  ( 26.99999999999999645, 7.347880794884117764E-16, -3.824999999999994849 ) ) ;
#32415=CARTESIAN_POINT ( 'NONE',  ( 34.06814574304114984, -5.196152422706635576, 164.9484496060674985 ) ) ;
#32416=CARTESIAN_POINT ( 'NONE',  ( 21.00000000000000355, 0.000000000000000000, 50.00000000000001421 ) ) ;
#32422=CARTESIAN_POINT ( 'NONE',  ( 15.24356964374999990, 0.000000000000000000, -1.940624999385465177 ) ) ;
#32425=CARTESIAN_POINT ( 'NONE',  ( 18.00000000000000000, 5.196152422706630247, -6.318749998770966769 ) ) ;
#32426=CARTESIAN_POINT ( 'NONE',  ( 28.39820154767614468, -5.196152422706638241, 168.9829703733268218 ) ) ;
#32430=CARTESIAN_POINT ( 'NONE',  ( 24.79356678040014117, -3.604726614523244610, 164.9975944357569517 ) ) ;
#32435=DIRECTION ( 'NONE',  ( 0.9961946980917462113, 0.000000000000000000, -0.08715574274765118534 ) ) ;
#32438=CARTESIAN_POINT ( 'NONE',  ( 28.14696362483655889, -5.407089921784859143, 167.5086318987019069 ) ) ;
#32447=EDGE_LOOP ( 'NONE', ( #1918, #16715, #19375, #16332 ) ) ;
#32456=CARTESIAN_POINT ( 'NONE',  ( 24.85399959338462139, 0.000000000000000000, 162.8936964012349051 ) ) ;
#32465=CARTESIAN_POINT ( 'NONE',  ( 21.00000000000000000, -6.646953231504538984, -5.540624999385494576 ) ) ;
#32468=ORIENTED_EDGE ( 'NONE', *, *, #33739, .F. ) ;
#32470=CARTESIAN_POINT ( 'NONE',  ( 15.24356964374999990, 3.323476615752268604, -5.128124999385462957 ) ) ;
#32476=CARTESIAN_POINT ( 'NONE',  ( 36.84101937412305716, 3.464101615137755275, 162.2214005012718587 ) ) ;
#32480=CARTESIAN_POINT ( 'NONE',  ( 15.24356964374999990, 3.323476615752268604, -7.940624999385462068 ) ) ;
#32488=CARTESIAN_POINT ( 'NONE',  ( 24.35560917309319251, 3.604726614523240613, 159.9917160778459220 ) ) ;
#32493=CARTESIAN_POINT ( 'NONE',  ( 15.00000000000000000, 0.000000000000000000, -2.193749998770949894 ) ) ;
#32496=CARTESIAN_POINT ( 'NONE',  ( 37.33780710767756972, 7.347880794884125653E-16, 167.8997102791704492 ) ) ;
#32501=VERTEX_POINT ( 'NONE', #21901 ) ;
#32502=CARTESIAN_POINT ( 'NONE',  ( 15.00000000000000178, -3.464101615137757051, -6.262500000000007283 ) ) ;
#32506=CARTESIAN_POINT ( 'NONE',  ( 31.24052741120653209, 7.209453229046475009, 167.0497639179608313 ) ) ;
#32515=CARTESIAN_POINT ( 'NONE',  ( 20.99999999999999645, -6.928203230275506996, -3.431249998770965703 ) ) ;
#32517=CARTESIAN_POINT ( 'NONE',  ( 26.75643035624999655, 3.323476615752271712, -5.278124999385452654 ) ) ;
#32521=ADVANCED_FACE ( 'NONE', ( #27202 ), #3704, .F. ) ;
#32526=CARTESIAN_POINT ( 'NONE',  ( 30.66693367924855096, -7.209453229046482114, 160.4935575611445415 ) ) ;
#32531=( BOUNDED_CURVE ( )  B_SPLINE_CURVE ( 2, ( #27918, #4795, #16373, #1949, #13519, #21689, #10670 ),
 .UNSPECIFIED., .F., .F. ) 
 B_SPLINE_CURVE_WITH_KNOTS ( ( 3, 2, 2, 3 ),
 ( 0.6521739130434789367, 0.6594202898550732828, 0.6666666666666675178, 0.6739130434782618639 ),
 .UNSPECIFIED. ) 
 CURVE ( )  GEOMETRIC_REPRESENTATION_ITEM ( )  RATIONAL_B_SPLINE_CURVE ( ( 0.9999999999999876765, 0.8660254037844510311, 1.000000000000000000, 0.8660254037844387076, 1.000000000000000000, 0.8660254037844202779, 1.000000000000018430 ) ) 
 REPRESENTATION_ITEM ( '' )  );
#32540=CARTESIAN_POINT ( 'NONE',  ( 28.22050128277989245, -5.407089921784865361, 168.3491711752168385 ) ) ;
#32550=ORIENTED_EDGE ( 'NONE', *, *, #17498, .T. ) ;
#32551=CARTESIAN_POINT ( 'NONE',  ( 30.59339602130522096, -7.209453229046475009, 159.6530182846296384 ) ) ;
#32552=CARTESIAN_POINT ( 'NONE',  ( 23.87821517812499650, 4.985214923628404904, -9.740624999385467220 ) ) ;
#32556=CARTESIAN_POINT ( 'NONE',  ( 31.07874456373120609, 7.209453229046482114, 165.2005775096280615 ) ) ;
#32557=CARTESIAN_POINT ( 'NONE',  ( 24.89648801797410727, -3.464101615137761048, 163.3793413165546440 ) ) ;
#32567=EDGE_CURVE ( 'NONE', #25042, #13953, #23132, .T. ) ;
#32569=CARTESIAN_POINT ( 'NONE',  ( 21.00000000000000000, -6.646953231504538984, -5.090624999385466865 ) ) ;
#32572=( BOUNDED_CURVE ( )  B_SPLINE_CURVE ( 3, ( #7115, #4069, #15641, #30227 ),
 .UNSPECIFIED., .F., .F. ) 
 B_SPLINE_CURVE_WITH_KNOTS ( ( 4, 4 ),
 ( 1.570796326794938302, 3.141592653589793116 ),
 .UNSPECIFIED. ) 
 CURVE ( )  GEOMETRIC_REPRESENTATION_ITEM ( )  RATIONAL_B_SPLINE_CURVE ( ( 1.000000000000000000, 0.8047378541243747074, 0.8047378541243747074, 1.000000000000000000 ) ) 
 REPRESENTATION_ITEM ( '' )  );
#32573=EDGE_CURVE ( 'NONE', #4816, #27974, #24351, .T. ) ;
#32579=CARTESIAN_POINT ( 'NONE',  ( 34.19561101691670757, -5.196152422706629359, 166.4053843532510371 ) ) ;
#32582=EDGE_CURVE ( 'NONE', #4196, #28188, #14169, .T. ) ;
#32585=CARTESIAN_POINT ( 'NONE',  ( 37.25116460488249004, -3.604726614523235284, 164.1147336928429468 ) ) ;
#32586=AXIS2_PLACEMENT_3D ( 'NONE', #5467, #11355, #6028 ) ;
#32590=CARTESIAN_POINT ( 'NONE',  ( 24.00000000000000000, -5.196152422706629359, -4.799999999999998934 ) ) ;
#32591=CYLINDRICAL_SURFACE ( 'NONE', #29662, 6.000000000000001776 ) ;
#32598=CARTESIAN_POINT ( 'NONE',  ( 34.41253136604939300, -5.407089921784855591, 167.4874711655023418 ) ) ;
#32599=CARTESIAN_POINT ( 'NONE',  ( 21.00000000000000000, 6.646953231504538984, -2.953124999385479565 ) ) ;
#32600=ADVANCED_FACE ( 'NONE', ( #36469 ), #11263, .T. ) ;
#32609=EDGE_LOOP ( 'NONE', ( #14378, #16032, #4906, #17280 ) ) ;
#32613=CARTESIAN_POINT ( 'NONE',  ( 21.00000000000000000, 6.646953231504538984, -1.153124999385464200 ) ) ;
#32615=CARTESIAN_POINT ( 'NONE',  ( 24.00000000000000000, -5.196152422706629359, -6.993749998770947940 ) ) ;
#32619=EDGE_CURVE ( 'NONE', #35077, #8427, #31350, .T. ) ;
#32622=CARTESIAN_POINT ( 'NONE',  ( 37.29201885929546023, 3.604726614523243278, 164.5816999575734201 ) ) ;
#32625=( LENGTH_UNIT ( ) NAMED_UNIT ( * ) SI_UNIT ( .MILLI., .METRE. ) );
#32629=CARTESIAN_POINT ( 'NONE',  ( 28.06852345636367119, -5.407089921784859143, 166.6120566704193493 ) ) ;
#32638=ORIENTED_EDGE ( 'NONE', *, *, #5005, .T. ) ;
#32641=DIRECTION ( 'NONE',  ( 0.08715574274765150453, 0.000000000000000000, 0.9961946980917461003 ) ) ;
#32644=PLANE ( 'NONE',  #26239 ) ;
#32656=CARTESIAN_POINT ( 'NONE',  ( 26.75643035624999655, 7.049594010296217766E-16, -3.628124999385473615 ) ) ;
#32661=CARTESIAN_POINT ( 'NONE',  ( 20.99999999999999645, 6.646953231504538984, -4.303124999385466332 ) ) ;
#32671=CARTESIAN_POINT ( 'NONE',  ( 18.12178482187500350, -4.985214923628407568, -6.478124999385492799 ) ) ;
#32680=CARTESIAN_POINT ( 'NONE',  ( 30.60810355289388696, 7.209453229046482114, 159.8211261399325736 ) ) ;
#32693=CARTESIAN_POINT ( 'NONE',  ( 18.00000000000000000, 5.196152422706630247, -5.925000000000013145 ) ) ;
#32695=CARTESIAN_POINT ( 'NONE',  ( 26.99999999999999645, 7.347880794884117764E-16, -6.918749998770956644 ) ) ;
#32697=CARTESIAN_POINT ( 'NONE',  ( 37.33614145406145468, 3.604726614523238837, 165.0860235234823392 ) ) ;
#32708=CARTESIAN_POINT ( 'NONE',  ( 15.24356964374999990, 3.323476615752268604, -9.178124999385456562 ) ) ;
#32709=VECTOR ( 'NONE', #3791, 1000.000000000000000 ) ;
#32716=CARTESIAN_POINT ( 'NONE',  ( 31.22336862440664618, 6.928203230275506996, 166.8536380873862015 ) ) ;
#32723=DIRECTION ( 'NONE',  ( -0.08715574274766001162, -2.055968571607451078E-14, -0.9961946980917453232 ) ) ;
#32731=CARTESIAN_POINT ( 'NONE',  ( 25.10732745429168489, -3.604726614523244610, 168.5838953488872676 ) ) ;
#32735=( BOUNDED_CURVE ( )  B_SPLINE_CURVE ( 2, ( #3252, #20895, #14826, #588, #12157, #23543, #26371 ),
 .UNSPECIFIED., .F., .F. ) 
 B_SPLINE_CURVE_WITH_KNOTS ( ( 3, 2, 2, 3 ),
 ( 0.4130434782608686795, 0.4202898550724629700, 0.4275362318840572606, 0.4347826086956515512 ),
 .UNSPECIFIED. ) 
 CURVE ( )  GEOMETRIC_REPRESENTATION_ITEM ( )  RATIONAL_B_SPLINE_CURVE ( ( 1.000000000000016431, 0.8660254037844222763, 1.000000000000000000, 0.8660254037844387076, 1.000000000000000000, 0.8660254037844500319, 0.9999999999999886757 ) ) 
 REPRESENTATION_ITEM ( '' )  );
#32745=CARTESIAN_POINT ( 'NONE',  ( 26.99999999999999645, 7.347880794884117764E-16, -1.068749998770962550 ) ) ;
#32746=CARTESIAN_POINT ( 'NONE',  ( 15.00000000000000000, 3.464101615137752166, -0.9375000000000204281 ) ) ;
#32748=CARTESIAN_POINT ( 'NONE',  ( 24.86547026816695904, 3.604726614523240613, 165.8194550616826461 ) ) ;
#32749=CARTESIAN_POINT ( 'NONE',  ( 36.94233792496010693, -3.464101615137755275, 163.3794768365791583 ) ) ;
#32754=ORIENTED_EDGE ( 'NONE', *, *, #5020, .F. ) ;
#32760=CARTESIAN_POINT ( 'NONE',  ( 21.00000000000000000, -6.646953231504538984, -5.540624999385494576 ) ) ;
#32762=( BOUNDED_CURVE ( )  B_SPLINE_CURVE ( 2, ( #37091, #16654, #16839, #22716, #28379, #27828, #7559 ),
 .UNSPECIFIED., .F., .F. ) 
 B_SPLINE_CURVE_WITH_KNOTS ( ( 3, 2, 2, 3 ),
 ( 0.6956521739130446802, 0.7028985507246381381, 0.7101449275362315960, 0.7173913043478249429 ),
 .UNSPECIFIED. ) 
 CURVE ( )  GEOMETRIC_REPRESENTATION_ITEM ( )  RATIONAL_B_SPLINE_CURVE ( ( 0.9999999999999774625, 0.8660254037844612451, 1.000000000000000000, 0.8660254037844387076, 1.000000000000000000, 0.8660254037844592467, 0.9999999999999794609 ) ) 
 REPRESENTATION_ITEM ( '' )  );
#32774=CARTESIAN_POINT ( 'NONE',  ( 15.00000000000000000, 0.000000000000000000, -0.3937499987709536242 ) ) ;
#32775=CARTESIAN_POINT ( 'NONE',  ( 34.05955060792140188, -5.407089921784855591, 163.4528826382307614 ) ) ;
#32780=CARTESIAN_POINT ( 'NONE',  ( 25.36386068845838082, 0.000000000000000000, 168.7214353850716293 ) ) ;
#32782=CARTESIAN_POINT ( 'NONE',  ( 18.00000000000000000, 5.196152422706630247, -2.268749998770941190 ) ) ;
#32788=CARTESIAN_POINT ( 'NONE',  ( 37.53224187524366329, 3.604726614523238837, 167.3274615941888044 ) ) ;
#32789=CARTESIAN_POINT ( 'NONE',  ( 26.75643035624999655, 7.049594010296217766E-16, -2.165624999385467930 ) ) ;
#32790=ADVANCED_FACE ( 'NONE', ( #30798 ), #34960, .T. ) ;
#32798=ORIENTED_EDGE ( 'NONE', *, *, #34596, .T. ) ;
#32801=CARTESIAN_POINT ( 'NONE',  ( 18.12178482187499640, 4.985214923628404904, -2.465624999385462868 ) ) ;
#32803=CARTESIAN_POINT ( 'NONE',  ( 21.00000000000000000, -6.928203230275506996, -8.381249998770950782 ) ) ;
#32809=CARTESIAN_POINT ( 'NONE',  ( 27.82830044041545747, -5.407089921784865361, 163.8662950338039650 ) ) ;
#32815=CARTESIAN_POINT ( 'NONE',  ( 31.24052741120653209, 7.209453229046475009, 167.0497639179608313 ) ) ;
#32816=ORIENTED_EDGE ( 'NONE', *, *, #10261, .T. ) ;
#32825=ORIENTED_EDGE ( 'NONE', *, *, #19589, .T. ) ;
#32834=CARTESIAN_POINT ( 'NONE',  ( 15.07120214184183737, -0.2399139898622077993, -8.000000000000019540 ) ) ;
#32835=CARTESIAN_POINT ( 'NONE',  ( 24.77229108455811257, 3.464101615137419543, 161.9597638717738732 ) ) ;
#32842=LINE ( 'NONE', #10102, #20955 ) ;
#32843=CARTESIAN_POINT ( 'NONE',  ( 18.12178482187500350, -4.985214923628407568, -4.678124999385496530 ) ) ;
#32845=ORIENTED_EDGE ( 'NONE', *, *, #5020, .T. ) ;
#32846=CARTESIAN_POINT ( 'NONE',  ( 26.75643035624999655, -3.323476615752267271, -6.703124999385464911 ) ) ;
#32853=CARTESIAN_POINT ( 'NONE',  ( 33.68574992184294103, -5.196152422706629359, 160.5776453694143129 ) ) ;
#32855=EDGE_CURVE ( 'NONE', #31903, #14365, #16600, .T. ) ;
#32861=CARTESIAN_POINT ( 'NONE',  ( 26.75643035624999655, 3.323476615752271268, -7.640624999385485339 ) ) ;
#32868=DIRECTION ( 'NONE',  ( 0.08715574274765150453, 0.000000000000000000, 0.9961946980917461003 ) ) ;
#32869=EDGE_CURVE ( 'NONE', #3429, #36284, #29651, .T. ) ;
#32883=CARTESIAN_POINT ( 'NONE',  ( 18.00000000000000355, -5.196152422706632912, -7.124999999999992895 ) ) ;
#32887=CARTESIAN_POINT ( 'NONE',  ( 24.79846929092969887, -3.604726614523240613, 165.0536303875245778 ) ) ;
#32888=CARTESIAN_POINT ( 'NONE',  ( 15.00000000000000000, 0.000000000000000000, -1.799999999999996048 ) ) ;
#32892=ORIENTED_EDGE ( 'NONE', *, *, #31372, .T. ) ;
#32893=CYLINDRICAL_SURFACE ( 'NONE', #6114, 5.999999999999994671 ) ;
#32894=CARTESIAN_POINT ( 'NONE',  ( 18.12178482187499640, 4.985214923628404904, -0.6656249993854668201 ) ) ;
#32897=CARTESIAN_POINT ( 'NONE',  ( 23.87821517812499650, 4.985214923628404904, -8.390624999385476457 ) ) ;
#32900=CARTESIAN_POINT ( 'NONE',  ( 24.78536444607796341, 0.000000000000000000, 162.1091930777120069 ) ) ;
#32904=CARTESIAN_POINT ( 'NONE',  ( 37.23322021648748859, 3.464101615137755275, 166.7042766426846754 ) ) ;
#32909=CARTESIAN_POINT ( 'NONE',  ( 36.75277418448325761, 3.464101615138157619, 161.2127533682296416 ) ) ;
#32916=CARTESIAN_POINT ( 'NONE',  ( 26.97716818855048260, 0.000000000000000000, 49.47706554351410801 ) ) ;
#32917=CARTESIAN_POINT ( 'NONE',  ( 34.25074851857407765, -5.407089921784861808, 165.6382847571695436 ) ) ;
#32924=CARTESIAN_POINT ( 'NONE',  ( 24.99999999999999289, 0.000000000000000000, 49.65004534589634488 ) ) ;
#32927=CYLINDRICAL_SURFACE ( 'NONE', #167, 6.000000000000001776 ) ;
#32934=CARTESIAN_POINT ( 'NONE',  ( 23.87821517812500005, -4.985214923628404016, -9.890624999385478233 ) ) ;
#32935=CARTESIAN_POINT ( 'NONE',  ( 34.06772145880400160, 5.407089921784862696, 163.5462758911768617 ) ) ;
#32936=CARTESIAN_POINT ( 'NONE',  ( 24.81151116879513907, 3.464101615137757051, 162.4080514859151663 ) ) ;
#32946=CARTESIAN_POINT ( 'NONE',  ( 23.87821517812500005, -4.985214923628404016, -5.953124999385495109 ) ) ;
#32950=PRODUCT_DEFINITION_FORMATION_WITH_SPECIFIED_SOURCE ( 'ANY', '', #11977, .NOT_KNOWN. ) ;
#32958=CARTESIAN_POINT ( 'NONE',  ( 15.00000000000000000, 0.000000000000000000, -3.149999999999986144 ) ) ;
#32959=( BOUNDED_CURVE ( )  B_SPLINE_CURVE ( 2, ( #12829, #18156, #29697, #3731, #21378, #16248, #2383 ),
 .UNSPECIFIED., .F., .F. ) 
 B_SPLINE_CURVE_WITH_KNOTS ( ( 3, 2, 2, 3 ),
 ( 0.02173913043478212584, 0.02898550724637647541, 0.03623188405797082151, 0.04347826086956516761 ),
 .UNSPECIFIED. ) 
 CURVE ( )  GEOMETRIC_REPRESENTATION_ITEM ( )  RATIONAL_B_SPLINE_CURVE ( ( 1.000000000000008882, 0.8660254037844299368, 1.000000000000000000, 0.8660254037844387076, 1.000000000000000000, 0.8660254037844395958, 0.9999999999999991118 ) ) 
 REPRESENTATION_ITEM ( '' )  );
#32963=CARTESIAN_POINT ( 'NONE',  ( 30.92676673731498482, 7.209453229046475009, 163.4634630048305439 ) ) ;
#32967=CARTESIAN_POINT ( 'NONE',  ( 28.35898146343970083, -5.196152422706638241, 168.5346827591855288 ) ) ;
#32974=CARTESIAN_POINT ( 'NONE',  ( 37.41458162253433528, 3.604726614523238837, 165.9825987517649253 ) ) ;
#32975=CARTESIAN_POINT ( 'NONE',  ( 15.24356964375000167, -3.323476615752272600, -3.253124999385455407 ) ) ;
#32977=CARTESIAN_POINT ( 'NONE',  ( 21.91998644642377769, -5.891742046770922059, -8.000000000000003553 ) ) ;
#32979=CARTESIAN_POINT ( 'NONE',  ( 25.09258843915658588, -3.464101615137914703, 165.6207793872610523 ) ) ;
#32989=CARTESIAN_POINT ( 'NONE',  ( 15.24356964375000167, -3.323476615752272600, -1.903124999385467753 ) ) ;
#32991=CARTESIAN_POINT ( 'NONE',  ( 18.00000000000000000, 5.196152422706630247, -9.918749998770959309 ) ) ;
#32999=CARTESIAN_POINT ( 'NONE',  ( 34.02850137456756130, 5.407089921784862696, 163.0979882770355971 ) ) ;
#33000=EDGE_CURVE ( 'NONE', #28137, #27706, #37382, .T. ) ;
#33004=CARTESIAN_POINT ( 'NONE',  ( 21.00000000000000355, 0.000000000000000000, 50.00000000000001421 ) ) ;
#33007=CARTESIAN_POINT ( 'NONE',  ( 25.06647319987872535, 3.604726614523236616, 168.1169290841567090 ) ) ;
#33009=VECTOR ( 'NONE', #14376, 1000.000000000000000 ) ;
#33018=( NAMED_UNIT ( * ) SI_UNIT ( $, .STERADIAN. ) SOLID_ANGLE_UNIT ( ) );
#33024=CARTESIAN_POINT ( 'NONE',  ( 24.00000000000000000, -5.196152422706629359, -2.099999999999990763 ) ) ;
#33027=CARTESIAN_POINT ( 'NONE',  ( 31.43172532185920076, 7.209453229046482114, 169.2351660368995852 ) ) ;
#33031=AXIS2_PLACEMENT_3D ( 'NONE', #14707, #23245, #14154 ) ;
#33036=DIRECTION ( 'NONE',  ( 0.08715574274765150453, 0.000000000000000000, 0.9961946980917461003 ) ) ;
#33037=CARTESIAN_POINT ( 'NONE',  ( 18.12178482187500350, -4.985214923628407568, -5.128124999385475391 ) ) ;
#33048=ADVANCED_FACE ( 'NONE', ( #3482 ), #11459, .T. ) ;
#33053=CARTESIAN_POINT ( 'NONE',  ( 20.99999999999999645, 6.646953231504538984, -6.215624999385504168 ) ) ;
#33054=CARTESIAN_POINT ( 'NONE',  ( 21.00000000000000355, 0.000000000000000000, 50.00000000000001421 ) ) ;
#33057=LINE ( 'NONE', #19234, #36503 ) ;
#33063=DIRECTION ( 'NONE',  ( 0.9961946980917462113, 0.000000000000000000, -0.08715574274765118534 ) ) ;
#33081=CARTESIAN_POINT ( 'NONE',  ( 27.93778984224218931, 5.407089921784856479, 165.1177646232817153 ) ) ;
#33086=ORIENTED_EDGE ( 'NONE', *, *, #36247, .T. ) ;
#33089=CARTESIAN_POINT ( 'NONE',  ( 15.24356964374999990, 0.000000000000000000, -1.490624999385459226 ) ) ;
#33091=CARTESIAN_POINT ( 'NONE',  ( 21.00000000000000000, -6.646953231504538984, -8.128124999385477167 ) ) ;
#33096=( BOUNDED_CURVE ( )  B_SPLINE_CURVE ( 2, ( #4461, #2172, #33459, #35922, #30808, #4644, #24926 ),
 .UNSPECIFIED., .F., .F. ) 
 B_SPLINE_CURVE_WITH_KNOTS ( ( 3, 2, 2, 3 ),
 ( 0.4347826086956526059, 0.4420289855072469520, 0.4492753623188412426, 0.4565217391304355332 ),
 .UNSPECIFIED. ) 
 CURVE ( )  GEOMETRIC_REPRESENTATION_ITEM ( )  RATIONAL_B_SPLINE_CURVE ( ( 0.9999999999999917843, 0.8660254037844469233, 1.000000000000000000, 0.8660254037844387076, 1.000000000000000000, 0.8660254037844243857, 1.000000000000014433 ) ) 
 REPRESENTATION_ITEM ( '' )  );
#33099=CARTESIAN_POINT ( 'NONE',  ( 28.25112623189659544, -5.196152422706632912, 167.3018918215213660 ) ) ;
#33103=CARTESIAN_POINT ( 'NONE',  ( 26.75643035624999655, 7.049594010296217766E-16, -0.4781249993854874702 ) ) ;
#33109=CARTESIAN_POINT ( 'NONE',  ( 26.97716818855048260, 0.000000000000000000, 49.47706554351410801 ) ) ;
#33111=CARTESIAN_POINT ( 'NONE',  ( 24.90795869275643426, 0.000000000000000000, 166.3050999770023850 ) ) ;
#33124=CARTESIAN_POINT ( 'NONE',  ( 26.99999999999999645, 7.347880794884117764E-16, -5.624999999999991118 ) ) ;
#33125=DIRECTION ( 'NONE',  ( 1.000000000000000000, 0.000000000000000000, 0.000000000000000000 ) ) ;
#33126=ORIENTED_EDGE ( 'NONE', *, *, #10754, .T. ) ;
#33128=CARTESIAN_POINT ( 'NONE',  ( 15.24356964375000167, -3.323476615752272600, -9.103124999385496352 ) ) ;
#33130=CARTESIAN_POINT ( 'NONE',  ( 27.69756682629397915, 5.407089921784862696, 162.3720029866663594 ) ) ;
#33131=CARTESIAN_POINT ( 'NONE',  ( 30.72331255028488428, -6.928203230275514990, 161.1379710058604644 ) ) ;
#33137=ORIENTED_EDGE ( 'NONE', *, *, #33000, .F. ) ;
#33142=AXIS2_PLACEMENT_3D ( 'NONE', #2512, #11232, #22804 ) ;
#33144=CARTESIAN_POINT ( 'NONE',  ( 15.24356964375000167, -3.323476615752272600, -5.615624999385488536 ) ) ;
#33147=CARTESIAN_POINT ( 'NONE',  ( 15.00000000000000178, -3.464101615137757051, -6.656249998770961795 ) ) ;
#33156=CARTESIAN_POINT ( 'NONE',  ( 37.17272443640959523, -3.604726614523235284, 163.2181584645603323 ) ) ;
#33158=CARTESIAN_POINT ( 'NONE',  ( 15.00000000000000000, 0.000000000000000000, -0.9000000000000119016 ) ) ;
#33159=CARTESIAN_POINT ( 'NONE',  ( 14.99999999999952394, -3.464101615137481716, -4.912499999999994316 ) ) ;
#33167=CARTESIAN_POINT ( 'NONE',  ( 27.83320295094501162, -5.407089921784859143, 163.9223309855715911 ) ) ;
#33169=CARTESIAN_POINT ( 'NONE',  ( 23.87821517812499650, 4.985214923628404904, -2.990624999385460558 ) ) ;
#33171=CARTESIAN_POINT ( 'NONE',  ( 28.17268606342371129, -5.196152422706632912, 166.4053165932387515 ) ) ;
#33172=CARTESIAN_POINT ( 'NONE',  ( 34.43419986258128773, 5.196152422706637353, 169.1324673380528623 ) ) ;
#33182=CARTESIAN_POINT ( 'NONE',  ( 15.24356964374999990, 3.323476615752268604, -1.078124999385470462 ) ) ;
#33184=CARTESIAN_POINT ( 'NONE',  ( 15.00000000000000178, -3.464101615137757051, -8.906249998770972454 ) ) ;
#33191=CARTESIAN_POINT ( 'NONE',  ( 27.89366724747619131, 5.407089921784862696, 164.6134410573727678 ) ) ;
#33195=( NAMED_UNIT ( * ) SI_UNIT ( $, .STERADIAN. ) SOLID_ANGLE_UNIT ( ) );
#33212=DIRECTION ( 'NONE',  ( 0.9961946980917462113, 0.000000000000000000, -0.08715574274765118534 ) ) ;
#33215=CARTESIAN_POINT ( 'NONE',  ( 27.00000000000003908, -3.464101615137728185, -2.062499999999993339 ) ) ;
#33218=EDGE_CURVE ( 'NONE', #4551, #11581, #34737, .T. ) ;
#33219=PLANE ( 'NONE',  #36917 ) ;
#33226=CARTESIAN_POINT ( 'NONE',  ( 18.12178482187500350, -4.985214923628407568, -4.228124999385491023 ) ) ;
#33229=VERTEX_POINT ( 'NONE', #35712 ) ;
#33230=CARTESIAN_POINT ( 'NONE',  ( 15.24356964374999990, 3.323476615752268604, -7.378124999385474503 ) ) ;
#33236=CARTESIAN_POINT ( 'NONE',  ( 30.61545731874177534, -6.928203230275506996, 159.9051800681962732 ) ) ;
#33243=( BOUNDED_CURVE ( )  B_SPLINE_CURVE ( 2, ( #11751, #23319, #5872, #7843, #31471, #26152, #22954 ),
 .UNSPECIFIED., .F., .F. ) 
 B_SPLINE_CURVE_WITH_KNOTS ( ( 3, 2, 2, 3 ),
 ( 0.5652173913043470055, 0.5724637681159410185, 0.5797101449275351426, 0.5869565217391291556 ),
 .UNSPECIFIED. ) 
 CURVE ( )  GEOMETRIC_REPRESENTATION_ITEM ( )  RATIONAL_B_SPLINE_CURVE ( ( 1.000000000000014433, 0.8660254037844243857, 1.000000000000000000, 0.8660254037844387076, 1.000000000000000000, 0.8660254037844633546, 0.9999999999999753530 ) ) 
 REPRESENTATION_ITEM ( '' )  );
#33252=EDGE_CURVE ( 'NONE', #33506, #25295, #27190, .T. ) ;
#33263=EDGE_CURVE ( 'NONE', #13931, #26175, #4966, .T. ) ;
#33264=CARTESIAN_POINT ( 'NONE',  ( 18.00000000000000355, -5.196152422706632912, -7.068749998770940124 ) ) ;
#33267=CARTESIAN_POINT ( 'NONE',  ( 34.03340388509710834, 5.407089921784857367, 163.1540242288032232 ) ) ;
#33275=CARTESIAN_POINT ( 'NONE',  ( 15.24356964375000167, -3.323476615752272600, -1.003124999385444305 ) ) ;
#33277=CARTESIAN_POINT ( 'NONE',  ( 15.00000000000000000, 0.000000000000000000, -5.849999999999994316 ) ) ;
#33278=CARTESIAN_POINT ( 'NONE',  ( 21.00000000000000000, 6.646953231504538984, -8.353124999385492799 ) ) ;
#33281=CARTESIAN_POINT ( 'NONE',  ( 27.78048522105927987, -5.196152422706632912, 161.9224404518259064 ) ) ;
#33285=CARTESIAN_POINT ( 'NONE',  ( 26.99999999999999289, 0.000000000000000000, 49.73803434254939759 ) ) ;
#33286=CARTESIAN_POINT ( 'NONE',  ( 37.18746345154497845, -3.464101615137751278, 166.1812744261865475 ) ) ;
#33290=CARTESIAN_POINT ( 'NONE',  ( 20.99999999999999645, 6.646953231504538984, -2.165624999385510563 ) ) ;
#33297=CARTESIAN_POINT ( 'NONE',  ( 30.73311757145110690, -6.928203230275506996, 161.2500429106201523 ) ) ;
#33300=CARTESIAN_POINT ( 'NONE',  ( 31.09835460584942624, -7.209453229046482114, 165.4247213166987081 ) ) ;
#33306=CARTESIAN_POINT ( 'NONE',  ( 15.00000000000000000, 0.000000000000000000, -2.643749998770955401 ) ) ;
#33308=DIRECTION ( 'NONE',  ( 0.08715574274765150453, 0.000000000000000000, 0.9961946980917461003 ) ) ;
#33316=CARTESIAN_POINT ( 'NONE',  ( 26.99999999999999645, 7.347880794884117764E-16, -2.925000000000010925 ) ) ;
#33317=CARTESIAN_POINT ( 'NONE',  ( 24.55824627498148160, -3.604726614523244610, 162.3078687509092788 ) ) ;
#33318=CARTESIAN_POINT ( 'NONE',  ( 36.70701741954144381, -3.464101615137755275, 160.6897511517314285 ) ) ;
#33320=CARTESIAN_POINT ( 'NONE',  ( 25.29522554115172639, 0.000000000000000000, 167.9369320615487311 ) ) ;
#33327=CYLINDRICAL_SURFACE ( 'NONE', #7182, 6.000000000000001776 ) ;
#33329=CARTESIAN_POINT ( 'NONE',  ( 18.12178482187500350, -4.985214923628407568, -6.478124999385492799 ) ) ;
#33334=EDGE_CURVE ( 'NONE', #22708, #25295, #12726, .T. ) ;
#33345=CARTESIAN_POINT ( 'NONE',  ( 24.56314878551103575, -3.604726614523240613, 162.3639047026768765 ) ) ;
#33347=CARTESIAN_POINT ( 'NONE',  ( 24.89648801797452293, -3.464101615138005741, 163.3793413165545587 ) ) ;
#33348=CARTESIAN_POINT ( 'NONE',  ( 15.00000000000000178, 0.000000000000000000, -3.993749998770945719 ) ) ;
#33356=EDGE_LOOP ( 'NONE', ( #34603, #15467, #6503, #36718 ) ) ;
#33357=CARTESIAN_POINT ( 'NONE',  ( 30.94637677943320497, -7.209453229046475009, 163.6876068119011904 ) ) ;
#33358=CARTESIAN_POINT ( 'NONE',  ( 26.75643035624999655, 3.323476615752271712, -5.278124999385452654 ) ) ;
#33360=CARTESIAN_POINT ( 'NONE',  ( 37.41624727615045742, 7.347880794884125653E-16, 168.7962855074530069 ) ) ;
#33361=CARTESIAN_POINT ( 'NONE',  ( 33.67594490067671842, -5.196152422706635576, 160.4655734646546534 ) ) ;
#33365=ORIENTED_EDGE ( 'NONE', *, *, #20123, .F. ) ;
#33369=CARTESIAN_POINT ( 'NONE',  ( 15.24356964375000167, -3.323476615752272600, -4.153124999385478411 ) ) ;
#33372=CARTESIAN_POINT ( 'NONE',  ( 26.99999999999999645, -3.464101615137751278, -10.10624999877097352 ) ) ;
#33375=EDGE_LOOP ( 'NONE', ( #34373, #22544, #11438, #26218 ) ) ;
#33380=CARTESIAN_POINT ( 'NONE',  ( 30.80420397407610622, 7.209453229046482114, 162.0625642106390671 ) ) ;
#33381=AXIS2_PLACEMENT_3D ( 'NONE', #13525, #31839, #32215 ) ;
#33388=ORIENTED_EDGE ( 'NONE', *, *, #26483, .T. ) ;
#33397=CARTESIAN_POINT ( 'NONE',  ( 29.49486714975617474, 6.148716665048037378, 159.5363409456820136 ) ) ;
#33401=CARTESIAN_POINT ( 'NONE',  ( 26.99999999999999645, 7.347880794884117764E-16, -2.024999999999999023 ) ) ;
#33407=VECTOR ( 'NONE', #17733, 1000.000000000000000 ) ;
#33412=CARTESIAN_POINT ( 'NONE',  ( 23.87821517812500005, -4.985214923628404016, -5.953124999385495109 ) ) ;
#33415=CARTESIAN_POINT ( 'NONE',  ( 18.12178482187500350, -4.985214923628407568, -6.365624999385477878 ) ) ;
#33417=CARTESIAN_POINT ( 'NONE',  ( 37.60577953318700395, 3.604726614523243278, 168.1680008707037075 ) ) ;
#33420=CARTESIAN_POINT ( 'NONE',  ( 29.51984228635672380, 5.908847293266075162, 159.3365288790247121 ) ) ;
#33431=DIRECTION ( 'NONE',  ( 0.000000000000000000, 0.000000000000000000, 1.000000000000000000 ) ) ;
#33444=CARTESIAN_POINT ( 'NONE',  ( 26.99999999999999289, 0.000000000000000000, -8.000000000000000000 ) ) ;
#33447=CARTESIAN_POINT ( 'NONE',  ( 34.13799077639428958, -5.407089921784855591, 164.3494578665133474 ) ) ;
#33456=CARTESIAN_POINT ( 'NONE',  ( 21.00000000000000000, -6.928203230275506996, -4.781249998770952914 ) ) ;
#33459=CARTESIAN_POINT ( 'NONE',  ( 18.00000000000000000, 5.196152422706630247, -4.574999999999995737 ) ) ;
#33460=CARTESIAN_POINT ( 'NONE',  ( 23.87821517812500005, -4.985214923628404016, -9.440624999385471838 ) ) ;
#33464=ADVANCED_FACE ( 'NONE', ( #29036 ), #14280, .T. ) ;
#33468=CARTESIAN_POINT ( 'NONE',  ( 34.27405118538959528, -5.196152422706629359, 167.3019595815335947 ) ) ;
#33472=CARTESIAN_POINT ( 'NONE',  ( 26.75643035624999655, 7.049594010296217766E-16, -1.828124999385477567 ) ) ;
#33476=EDGE_CURVE ( 'NONE', #10799, #30158, #20462, .T. ) ;
#33478=CARTESIAN_POINT ( 'NONE',  ( 36.71682244070834855, -3.464101615137353374, 160.8018230564910027 ) ) ;
#33482=CARTESIAN_POINT ( 'NONE',  ( 27.86752052465190133, -5.407089921784865361, 164.3145826479452296 ) ) ;
#33496=ORIENTED_EDGE ( 'NONE', *, *, #5464, .F. ) ;
#33497=CARTESIAN_POINT ( 'NONE',  ( 21.00000000000000000, 6.928203230275506996, -1.462500000000010125 ) ) ;
#33499=CARTESIAN_POINT ( 'NONE',  ( 24.63341810310133084, 0.000000000000000000, 163.1670866780133906 ) ) ;
#33500=CARTESIAN_POINT ( 'NONE',  ( 33.84589859903464060, 5.196152422706637353, 162.4081531259335804 ) ) ;
#33506=VERTEX_POINT ( 'NONE', #11431 ) ;
#33511=CARTESIAN_POINT ( 'NONE',  ( 21.00000000000000000, 6.646953231504538984, -6.215624999385504168 ) ) ;
#33513=AXIS2_PLACEMENT_3D ( 'NONE', #30185, #4772, #10458 ) ;
#33526=CARTESIAN_POINT ( 'NONE',  ( 27.66324925258708589, 5.407089921784856479, 161.9797513242927209 ) ) ;
#33527=CARTESIAN_POINT ( 'NONE',  ( 15.00000000000000000, 3.464101615137752166, -0.8812499987709473404 ) ) ;
#33529=CARTESIAN_POINT ( 'NONE',  ( 33.87204532185894124, -5.196152422706635576, 162.7070115353610618 ) ) ;
#33530=CARTESIAN_POINT ( 'NONE',  ( 15.00000000000000000, 0.000000000000000000, -4.049999999999998046 ) ) ;
#33539=CARTESIAN_POINT ( 'NONE',  ( 24.87037277869651319, 3.604726614523236616, 165.8754910134502722 ) ) ;
#33540=CARTESIAN_POINT ( 'NONE',  ( 23.87821517812499650, 4.985214923628404904, -5.690624999385468286 ) ) ;
#33556=CARTESIAN_POINT ( 'NONE',  ( 26.75643035624999655, -3.323476615752267715, -4.903124999385481964 ) ) ;
#33560=CARTESIAN_POINT ( 'NONE',  ( 21.00000000000000000, -6.928203230275506996, -9.731249998770937992 ) ) ;
#33567=CARTESIAN_POINT ( 'NONE',  ( 37.08938175740716758, -3.604726614523238837, 162.2655472845100917 ) ) ;
#33575=VERTEX_POINT ( 'NONE', #11245 ) ;
#33576=CARTESIAN_POINT ( 'NONE',  ( 15.00000000000000355, 7.347880794884112834E-16, -8.000000000000000000 ) ) ;
#33587=CARTESIAN_POINT ( 'NONE',  ( 18.00000000000000355, -5.196152422706632912, -5.775000000000002132 ) ) ;
#33591=DIRECTION ( 'NONE',  ( 0.000000000000000000, 0.000000000000000000, 1.000000000000000000 ) ) ;
#33593=CARTESIAN_POINT ( 'NONE',  ( 18.00000000000000355, -5.196152422706632912, -9.374999999999994671 ) ) ;
#33594=ORIENTED_EDGE ( 'NONE', *, *, #10257, .F. ) ;
#33599=CARTESIAN_POINT ( 'NONE',  ( 26.75643035624999655, 3.323476615752271712, -6.740624999385494753 ) ) ;
#33601=EDGE_CURVE ( 'NONE', #12755, #15590, #14713, .T. ) ;
#33603=CARTESIAN_POINT ( 'NONE',  ( 36.99463137071579411, 7.347880794884117764E-16, 163.9771936566585566 ) ) ;
#33605=VECTOR ( 'NONE', #12844, 1000.000000000000000 ) ;
#33606=CARTESIAN_POINT ( 'NONE',  ( 28.25972136701633630, -5.407089921784865361, 168.7974587893581315 ) ) ;
#33639=CARTESIAN_POINT ( 'NONE',  ( 37.25770128558855987, 3.604726614523238837, 164.1894482951998100 ) ) ;
#33640=CARTESIAN_POINT ( 'NONE',  ( 15.24356964374999990, 3.323476615752268604, -0.2906249993854697622 ) ) ;
#33644=VERTEX_POINT ( 'NONE', #5545 ) ;
#33646=CARTESIAN_POINT ( 'NONE',  ( 23.99999999999999645, 5.196152422706631135, -5.493749998770947052 ) ) ;
#33647=CARTESIAN_POINT ( 'NONE',  ( 15.24356964374999990, 0.000000000000000000, -0.5906249993854750802 ) ) ;
#33656=CARTESIAN_POINT ( 'NONE',  ( 25.05663669538002836, 3.464101615137752166, 165.2098490755225555 ) ) ;
#33660=CARTESIAN_POINT ( 'NONE',  ( 20.99999999999999645, -6.646953231504538984, -2.390624999385460914 ) ) ;
#33665=CARTESIAN_POINT ( 'NONE',  ( 36.72009078106068358, 7.347880794884117764E-16, 160.8391803576695622 ) ) ;
#33667=EDGE_CURVE ( 'NONE', #34407, #1229, #26498, .T. ) ;
#33669=CARTESIAN_POINT ( 'NONE',  ( 18.65685424949248628, 4.000000000000095035, 50.10230395283967653 ) ) ;
#33670=CARTESIAN_POINT ( 'NONE',  ( 34.13308826586474254, -5.407089921784861808, 164.2934219147456929 ) ) ;
#33679=DIRECTION ( 'NONE',  ( 0.000000000000000000, 0.000000000000000000, 1.000000000000000000 ) ) ;
#33684=ORIENTED_EDGE ( 'NONE', *, *, #33807, .T. ) ;
#33685=CARTESIAN_POINT ( 'NONE',  ( 21.00000000000000000, -6.928203230275506996, -1.237499999999996270 ) ) ;
#33686=CARTESIAN_POINT ( 'NONE',  ( 34.05464809739185483, -5.407089921784861808, 163.3968466864631068 ) ) ;
#33687=CARTESIAN_POINT ( 'NONE',  ( 30.78214267663955184, 6.928203230275514990, 161.8104024270723755 ) ) ;
#33691=VECTOR ( 'NONE', #12375, 1000.000000000000000 ) ;
#33699=CARTESIAN_POINT ( 'NONE',  ( 18.12178482187500350, -4.985214923628407568, -8.728124999385494576 ) ) ;
#33710=CARTESIAN_POINT ( 'NONE',  ( 31.05668326629465170, 6.928203230275514990, 164.9484157260613699 ) ) ;
#33711=CARTESIAN_POINT ( 'NONE',  ( 33.82423010250274586, -5.407089921784855591, 160.7631569533830600 ) ) ;
#33715=CARTESIAN_POINT ( 'NONE',  ( 36.58935716683290451, -3.464101615137295642, 159.3448883093075779 ) ) ;
#33717=CARTESIAN_POINT ( 'NONE',  ( 15.02283181144952628, 7.347880794884122694E-16, 50.52293445648592751 ) ) ;
#33723=VERTEX_POINT ( 'NONE', #29995 ) ;
#33724=CARTESIAN_POINT ( 'NONE',  ( 24.79520095057666396, 0.000000000000000000, 165.0162730863461604 ) ) ;
#33725=CARTESIAN_POINT ( 'NONE',  ( 23.87821517812500005, -4.985214923628404016, -4.940624999385468286 ) ) ;
#33729=CARTESIAN_POINT ( 'NONE',  ( 34.53836246964132073, 5.407089921784862696, 168.9257272608723213 ) ) ;
#33730=CARTESIAN_POINT ( 'NONE',  ( 25.32790894457497899, -3.464101615137761048, 168.3105050721087821 ) ) ;
#33737=ORIENTED_EDGE ( 'NONE', *, *, #35976, .F. ) ;
#33739=EDGE_CURVE ( 'NONE', #10799, #10052, #36951, .T. ) ;
#33741=CARTESIAN_POINT ( 'NONE',  ( 26.75643035624999655, -3.323476615752267715, -3.103124999385467486 ) ) ;
#33745=CARTESIAN_POINT ( 'NONE',  ( 18.12178482187499640, 4.985214923628404904, -1.678124999385494087 ) ) ;
#33751=ADVANCED_FACE ( 'NONE', ( #35861 ), #23940, .T. ) ;
#33761=FACE_OUTER_BOUND ( 'NONE', #30948, .T. ) ;
#33764=ADVANCED_FACE ( 'NONE', ( #4399 ), #12751, .T. ) ;
#33768=ORIENTED_EDGE ( 'NONE', *, *, #20856, .T. ) ;
#33779=CARTESIAN_POINT ( 'NONE',  ( 26.99999999999999645, 7.347880794884117764E-16, -9.674999999999990052 ) ) ;
#33786=CARTESIAN_POINT ( 'NONE',  ( 18.12178482187499640, 4.985214923628404904, -6.178124999385470772 ) ) ;
#33807=EDGE_CURVE ( 'NONE', #16979, #15182, #26548, .T. ) ;
#33818=CARTESIAN_POINT ( 'NONE',  ( 26.99999999999999645, 7.347880794884117764E-16, -4.725000000000006750 ) ) ;
#33828=CARTESIAN_POINT ( 'NONE',  ( 37.09428426793671463, -3.604726614523235284, 162.3215832362777746 ) ) ;
#33829=CARTESIAN_POINT ( 'NONE',  ( 23.87821517812499650, 4.985214923628404904, -0.8531249993854739255 ) ) ;
#33835=CARTESIAN_POINT ( 'NONE',  ( 15.00000000000000000, 3.464101615137752166, -4.031249998770949361 ) ) ;
#33836=CARTESIAN_POINT ( 'NONE',  ( 26.75643035624999655, 7.049594010296217766E-16, -3.065624999385479832 ) ) ;
#33838=CARTESIAN_POINT ( 'NONE',  ( 24.82131618996089273, 3.464101615137476831, 162.5201233906748826 ) ) ;
#33844=CARTESIAN_POINT ( 'NONE',  ( 30.98804811898798661, 6.928203230275506996, 164.1639124025385001 ) ) ;
#33848=CARTESIAN_POINT ( 'NONE',  ( 23.87821517812499650, 4.985214923628404904, -2.203124999385491556 ) ) ;
#33852=ORIENTED_EDGE ( 'NONE', *, *, #28922, .T. ) ;
#33853=CARTESIAN_POINT ( 'NONE',  ( 30.92921799263332261, -6.928203230275506996, 163.4914809813265606 ) ) ;
#33857=CARTESIAN_POINT ( 'NONE',  ( 30.94147426890365438, -7.209453229046482114, 163.6315708601335359 ) ) ;
#33862=DIRECTION ( 'NONE',  ( 0.9961946980917462113, 0.000000000000000000, -0.08715574274765118534 ) ) ;
#33867=DIRECTION ( 'NONE',  ( 0.000000000000000000, 0.000000000000000000, 1.000000000000000000 ) ) ;
#33872=CARTESIAN_POINT ( 'NONE',  ( 18.00000000000000000, 5.196152422706630247, -2.774999999999999467 ) ) ;
#33873=CARTESIAN_POINT ( 'NONE',  ( 36.98809468990209126, 3.464101615138066137, 163.9024790530773430 ) ) ;
#33874=CARTESIAN_POINT ( 'NONE',  ( 27.59297993499679791, -5.407089921784865361, 161.1765693489562352 ) ) ;
#33876=CARTESIAN_POINT ( 'NONE',  ( 33.63672481644027812, -5.196152422706635576, 160.0172858505133604 ) ) ;
#33884=CARTESIAN_POINT ( 'NONE',  ( 37.21687851461555852, -3.464101615137548773, 166.5174901355681243 ) ) ;
#33886=CARTESIAN_POINT ( 'NONE',  ( 26.75643035624999655, 3.323476615752271712, -9.890624999385464022 ) ) ;
#33898=CARTESIAN_POINT ( 'NONE',  ( 36.90145218710753738, 7.646167579472015790E-16, 160.1175024667497837 ) ) ;
#33903=CARTESIAN_POINT ( 'NONE',  ( 17.00000000000000000, 4.898587196589406912E-16, -8.000000000000000000 ) ) ;
#33910=CARTESIAN_POINT ( 'NONE',  ( 34.09877069215784218, -5.407089921784855591, 163.9011702523720544 ) ) ;
#33911=CARTESIAN_POINT ( 'NONE',  ( 21.00000000000000000, -6.646953231504538984, -5.878124999385467397 ) ) ;
#33913=CARTESIAN_POINT ( 'NONE',  ( 25.14001085782205891, 3.604726614523240613, 168.9574683606716974 ) ) ;
#33915=DIRECTION ( 'NONE',  ( 0.000000000000000000, 0.000000000000000000, 1.000000000000000000 ) ) ;
#33917=CARTESIAN_POINT ( 'NONE',  ( 26.99999999999999645, 7.347880794884117764E-16, -3.374999999999989342 ) ) ;
#33925=CARTESIAN_POINT ( 'NONE',  ( 15.24356964374999990, 3.323476615752268604, -5.128124999385462957 ) ) ;
#33928=EDGE_CURVE ( 'NONE', #9957, #941, #25120, .T. ) ;
#33929=CARTESIAN_POINT ( 'NONE',  ( 15.24356964375000167, -3.323476615752272600, -2.015624999385490668 ) ) ;
#33949=CARTESIAN_POINT ( 'NONE',  ( 25.01527935017339743, 2.343145750507547032, 50.00000000000000000 ) ) ;
#33955=CYLINDRICAL_SURFACE ( 'NONE', #18524, 6.000000000000001776 ) ;
#33960=CARTESIAN_POINT ( 'NONE',  ( 15.00000000000000000, 0.000000000000000000, -9.000000000000007105 ) ) ;
#33965=CARTESIAN_POINT ( 'NONE',  ( 18.12178482187500350, -4.985214923628407568, -6.928124999385470772 ) ) ;
#33972=CARTESIAN_POINT ( 'NONE',  ( 31.43172532185919721, 7.209453229046482114, 169.2351660368996420 ) ) ;
#33973=( BOUNDED_SURFACE ( )  B_SPLINE_SURFACE ( 1, 2, ( 
 ( #18968, #15933, #24821, #30523, #33172, #7956, #33360, #4543, #27482, #19349, #2073, #10793, #24637, #36752, #13646, #30709, #25199, #7584, #27293, #7216, #4172, #10420, #12892, #25005, #19160, #4729, #10044, #16304, #18788, #16119, #30329, #1884, #15742, #10232, #21621, #4353, #21807, #22366, #27670, #36374, #10602, #30888, #21995, #27851, #36561, #13455, #22182, #33730, #4911, #16492, #28040, #30142, #1324, #11719, #34650, #28403, #17235, #34470, #22739, #34289, #23293, #23106, #34838, #3000, #25941, #31078, #25382, #8332, #34098, #8694, #19531, #13835, #25566, #5101, #10978, #5286, #2256, #16680, #31260, #17422, #31443, #2624, #8148, #19902, #36932, #28773, #5466, #22549, #14570, #14383, #28962, #19720, #14200, #11166, #25751, #17048, #28586, #16866, #2813, #28227, #26122, #8513, #2442, #14016, #22925, #37118, #20268, #20080, #37304, #11354, #31624, #5652, #37484, #11535, #31807, #5844, #154, #8878, #20830, #35026, #17613, #12474, #29528, #6027, #9070, #12283, #3184, #12662, #23664, #711, #14760, #3375, #29143, #20456, #9633, #26873, #24043, #15322, #904, #35588, #21210, #18173, #26304, #341, #29714, #6786, #24230, #11906, #6221, #23473, #35395, #32749, #35208, #9443, #3747, #3568, #9258, #20640, #21022, #18360, #31998, #32187, #17794, #29337, #14944, #27069, #6410, #32372, #29909, #3938, #26491, #523, #15513, #17985, #12090, #1093, #15130, #26681, #23856, #32557, #6599, #27997, #13414, #7174, #33500, #13233, #1470, #13044, #2030, #1844, #13607, #19311, #4685, #9818, #4132, #24599, #12849, #24962, #35774, #30100, #4314, #21395, #27255, #21584, #18558, #32936, #10003, #33687, #10192, #18930, #24417, #36149, #15704, #7545, #21768, #1278, #30849, #30667, #7728, #35965, #30483, #27438, #4503, #33318, #7358, #33131, #19117, #6990, #4874, #24782, #18747, #30289, #1659, #15893, #36520, #36333, #16080, #27629, #10379, #21954, #16266, #27816, #10564, #22141, #16453, #25157, #37079, #13796, #33876, #28731, #8288, #22324, #25343, #28545, #19492, #28920, #2401, #17004, #31038, #19679, #7918, #36712, #25896, #5606, #2769, #31583, #17191, #14342, #37444 ),
 ( #11493, #17377, #23062, #34059, #22879, #2587, #28366, #13976, #2954, #34608, #10751, #8651, #20220, #5060, #16642, #25526, #2214, #31766, #28183, #36892, #31218, #10938, #22512, #8105, #5247, #16824, #11125, #5797, #22702, #19861, #34246, #31404, #5423, #34430, #14157, #25711, #37264, #20037, #11311, #8467, #9210, #6175, #20781, #26446, #12046, #8838, #35346, #11673, #35540, #3516, #14710, #29854, #17935, #3142, #29668, #15083, #293, #17747, #479, #23248, #32324, #6364, #23616, #32506, #14524, #26080, #35160, #26258, #34794, #18125, #29479, #20410, #11859, #26633, #31952, #18314, #29288, #662, #5984, #9022, #17564, #109, #15272, #6552, #3703, #20974, #26825, #855, #12426, #23805, #29099, #23428, #9585, #12234, #34980, #20594, #32135, #9399, #3327, #23995, #21159, #32697, #14898, #6739, #4263, #15652, #16029, #13176, #15463, #27200, #9770, #18507, #30046, #22089, #1416, #27386, #21899, #4635, #4080, #21348, #36281, #15838, #33081, #1226, #12798, #33639, #12994, #24549, #33447, #16214, #24367, #32887, #10329, #36100, #7124, #7490, #18696, #6938, #24179, #30429, #19066, #7678, #30618, #35911, #1607, #18878, #30237, #10143, #19258, #27764, #3892, #24916, #1794, #27017, #9954, #21716, #21535, #13361, #1042, #35724, #33267, #12613, #7306, #4449, #27578, #24731, #36468, #10509, #5195, #13926, #7865, #19627, #13549, #28498, #34006, #33828, #25847, #25660, #28680, #19439, #25476, #22459, #37027, #16770, #28316, #25102, #14108, #27947, #14294, #19815, #30989, #8601, #34194, #5007, #8421, #31349, #16588, #8051, #2354, #1977, #11073, #22648, #8240, #11261, #30797, #4820, #5376, #28133, #36660, #34380, #16955, #10698, #2162, #2541, #22275, #34562, #31173, #37214, #13745, #25291, #36843, #16401, #31534, #22832, #19990, #5559, #17144, #2718, #37395, #11445, #10886, #23012, #15229, #23571, #17327, #34748, #31720, #435, #2905, #15040, #35116, #20732, #14477, #14853, #20547, #31906, #32275, #29435, #5747, #5935, #26030, #3471, #28870, #3658, #9165, #20363, #35492, #6318, #8791, #35298, #17890, #17515, #23382, #6122, #58, #12000, #26402, #29240, #617 ) ),
 .UNSPECIFIED., .F., .F., .F. ) 
 B_SPLINE_SURFACE_WITH_KNOTS ( ( 2, 2 ),
 ( 3, 2, 2, 2, 2, 2, 2, 2, 2, 2, 2, 2, 2, 2, 2, 2, 2, 2, 2, 2, 2, 2, 2, 2, 2, 2, 2, 2, 2, 2, 2, 2, 2, 2, 2, 2, 2, 2, 2, 2, 2, 2, 2, 2, 2, 2, 2, 2, 2, 2, 2, 2, 2, 2, 2, 2, 2, 2, 2, 2, 2, 2, 2, 2, 2, 2, 2, 2, 2, 2, 2, 2, 2, 2, 2, 2, 2, 2, 2, 2, 2, 2, 2, 2, 2, 2, 2, 2, 2, 2, 2, 2, 2, 2, 2, 2, 2, 2, 2, 2, 2, 2, 2, 2, 2, 2, 2, 2, 2, 2, 2, 2, 2, 2, 2, 2, 2, 2, 2, 2, 2, 2, 2, 2, 2, 2, 2, 2, 2, 2, 2, 2, 2, 2, 3 ),
 ( 0.000000000000000000, 1.000000000000000000 ),
 ( 0.000000000000000000, 0.007246376811594202987, 0.01449275362318840597, 0.02173913043478260809, 0.02898550724637681195, 0.03623188405797101580, 0.04347826086956521618, 0.05072463768115942351, 0.05797101449275362389, 0.06521739130434782428, 0.07246376811594203160, 0.07971014492753622505, 0.08695652173913043237, 0.09420289855072463969, 0.1014492753623188470, 0.1086956521739130405, 0.1159420289855072478, 0.1231884057971014551, 0.1304347826086956486, 0.1376811594202898559, 0.1449275362318840632, 0.1521739130434782705, 0.1594202898550724501, 0.1666666666666666574, 0.1739130434782608647, 0.1811594202898550721, 0.1884057971014492794, 0.1956521739130434867, 0.2028985507246376940, 0.2101449275362318736, 0.2173913043478260809, 0.2246376811594202882, 0.2318840579710144956, 0.2391304347826087029, 0.2463768115942029102, 0.2536231884057971175, 0.2608695652173912971, 0.2681159420289855322, 0.2753623188405797118, 0.2826086956521738913, 0.2898550724637681264, 0.2971014492753623060, 0.3043478260869565410, 0.3115942028985507206, 0.3188405797101449002, 0.3260869565217391353, 0.3333333333333333148, 0.3405797101449275499, 0.3478260869565217295, 0.3550724637681159646, 0.3623188405797101441, 0.3695652173913043237, 0.3768115942028985588, 0.3840579710144927383, 0.3913043478260869734, 0.3985507246376811530, 0.4057971014492753881, 0.4130434782608695676, 0.4202898550724637472, 0.4275362318840579823, 0.4347826086956521618, 0.4420289855072463969, 0.4492753623188405765, 0.4565217391304347561, 0.4637681159420289911, 0.4710144927536231707, 0.4782608695652174058, 0.4855072463768115854, 0.4927536231884058204, 0.5000000000000000000, 0.5072463768115942351, 0.5144927536231883591, 0.5217391304347825942, 0.5289855072463768293, 0.5362318840579710644, 0.5434782608695651884, 0.5507246376811594235, 0.5579710144927536586, 0.5652173913043477826, 0.5724637681159420177, 0.5797101449275362528, 0.5869565217391304879, 0.5942028985507246119, 0.6014492753623188470, 0.6086956521739130821, 0.6159420289855072062, 0.6231884057971014412, 0.6304347826086956763, 0.6376811594202898004, 0.6449275362318840354, 0.6521739130434782705, 0.6594202898550725056, 0.6666666666666666297, 0.6739130434782608647, 0.6811594202898550998, 0.6884057971014492239, 0.6956521739130434590, 0.7028985507246376940, 0.7101449275362319291, 0.7173913043478260532, 0.7246376811594202882, 0.7318840579710145233, 0.7391304347826086474, 0.7463768115942028825, 0.7536231884057971175, 0.7608695652173913526, 0.7681159420289854767, 0.7753623188405797118, 0.7826086956521739468, 0.7898550724637680709, 0.7971014492753623060, 0.8043478260869565410, 0.8115942028985507761, 0.8188405797101449002, 0.8260869565217391353, 0.8333333333333333703, 0.8405797101449274944, 0.8478260869565217295, 0.8550724637681159646, 0.8623188405797101996, 0.8695652173913043237, 0.8768115942028985588, 0.8840579710144927938, 0.8913043478260869179, 0.8985507246376811530, 0.9057971014492753881, 0.9130434782608695121, 0.9202898550724637472, 0.9275362318840579823, 0.9347826086956522174, 0.9420289855072463414, 0.9492753623188405765, 0.9565217391304348116, 0.9637681159420289356, 0.9662082948456578446 ),
 .UNSPECIFIED. ) 
 GEOMETRIC_REPRESENTATION_ITEM ( )  RATIONAL_B_SPLINE_SURFACE ( (
 ( 1.000000000000000000, 0.8660254037844387076, 1.000000000000000000, 0.8660254037844387076, 1.000000000000000000, 0.8660254037844387076, 1.000000000000000000, 0.8660254037844387076, 1.000000000000000000, 0.8660254037844387076, 1.000000000000000000, 0.8660254037844387076, 1.000000000000000000, 0.8660254037844387076, 1.000000000000000000, 0.8660254037844387076, 1.000000000000000000, 0.8660254037844387076, 1.000000000000000000, 0.8660254037844387076, 1.000000000000000000, 0.8660254037844387076, 1.000000000000000000, 0.8660254037844387076, 1.000000000000000000, 0.8660254037844387076, 1.000000000000000000, 0.8660254037844387076, 1.000000000000000000, 0.8660254037844387076, 1.000000000000000000, 0.8660254037844387076, 1.000000000000000000, 0.8660254037844387076, 1.000000000000000000, 0.8660254037844387076, 1.000000000000000000, 0.8660254037844387076, 1.000000000000000000, 0.8660254037844387076, 1.000000000000000000, 0.8660254037844387076, 1.000000000000000000, 0.8660254037844387076, 1.000000000000000000, 0.8660254037844387076, 1.000000000000000000, 0.8660254037844387076, 1.000000000000000000, 0.8660254037844387076, 1.000000000000000000, 0.8660254037844387076, 1.000000000000000000, 0.8660254037844387076, 1.000000000000000000, 0.8660254037844387076, 1.000000000000000000, 0.8660254037844387076, 1.000000000000000000, 0.8660254037844387076, 1.000000000000000000, 0.8660254037844387076, 1.000000000000000000, 0.8660254037844387076, 1.000000000000000000, 0.8660254037844387076, 1.000000000000000000, 0.8660254037844387076, 1.000000000000000000, 0.8660254037844387076, 1.000000000000000000, 0.8660254037844387076, 1.000000000000000000, 0.8660254037844387076, 1.000000000000000000, 0.8660254037844387076, 1.000000000000000000, 0.8660254037844387076, 1.000000000000000000, 0.8660254037844387076, 1.000000000000000000, 0.8660254037844387076, 1.000000000000000000, 0.8660254037844387076, 1.000000000000000000, 0.8660254037844387076, 1.000000000000000000, 0.8660254037844387076, 1.000000000000000000, 0.8660254037844387076, 1.000000000000000000, 0.8660254037844387076, 1.000000000000000000, 0.8660254037844387076, 1.000000000000000000, 0.8660254037844387076, 1.000000000000000000, 0.8660254037844387076, 1.000000000000000000, 0.8660254037844387076, 1.000000000000000000, 0.8660254037844387076, 1.000000000000000000, 0.8660254037844387076, 1.000000000000000000, 0.8660254037844387076, 1.000000000000000000, 0.8660254037844387076, 1.000000000000000000, 0.8660254037844387076, 1.000000000000000000, 0.8660254037844387076, 1.000000000000000000, 0.8660254037844387076, 1.000000000000000000, 0.8660254037844387076, 1.000000000000000000, 0.8660254037844387076, 1.000000000000000000, 0.8660254037844387076, 1.000000000000000000, 0.8660254037844387076, 1.000000000000000000, 0.8660254037844387076, 1.000000000000000000, 0.8660254037844387076, 1.000000000000000000, 0.8660254037844387076, 1.000000000000000000, 0.8660254037844387076, 1.000000000000000000, 0.8660254037844387076, 1.000000000000000000, 0.8660254037844387076, 1.000000000000000000, 0.8660254037844387076, 1.000000000000000000, 0.8660254037844387076, 1.000000000000000000, 0.8660254037844387076, 1.000000000000000000, 0.8660254037844387076, 1.000000000000000000, 0.8660254037844387076, 1.000000000000000000, 0.8660254037844387076, 1.000000000000000000, 0.8660254037844387076, 1.000000000000000000, 0.8660254037844387076, 1.000000000000000000, 0.8660254037844387076, 1.000000000000000000, 0.8660254037844387076, 1.000000000000000000, 0.8660254037844387076, 1.000000000000000000, 0.8660254037844387076, 1.000000000000000000, 0.8660254037844387076, 1.000000000000000000, 0.8660254037844387076, 1.000000000000000000, 0.8660254037844387076, 1.000000000000000000, 0.8660254037844387076, 1.000000000000000000, 0.8660254037844387076, 1.000000000000000000, 0.8660254037844387076, 1.000000000000000000, 0.8660254037844387076, 1.000000000000000000, 0.8660254037844387076, 1.000000000000000000, 0.8660254037844387076, 1.000000000000000000, 0.8660254037844387076, 1.000000000000000000, 0.8660254037844387076, 1.000000000000000000, 0.8660254037844387076, 1.000000000000000000, 0.8660254037844387076, 1.000000000000000000, 0.8660254037844387076, 1.000000000000000000, 0.8660254037844387076, 1.000000000000000000, 0.8660254037844387076, 1.000000000000000000, 0.8660254037844387076, 1.000000000000000000, 0.8660254037844387076, 1.000000000000000000, 0.8660254037844387076, 1.000000000000000000, 0.8660254037844387076, 1.000000000000000000, 0.8660254037844387076, 1.000000000000000000, 0.8660254037844387076, 1.000000000000000000, 0.8660254037844387076, 1.000000000000000000, 0.8660254037844387076, 1.000000000000000000, 0.8660254037844387076, 1.000000000000000000, 0.8660254037844387076, 1.000000000000000000, 0.8660254037844387076, 1.000000000000000000, 0.8660254037844387076, 1.000000000000000000, 0.8660254037844387076, 1.000000000000000000, 0.8660254037844387076, 1.000000000000000000, 0.8660254037844387076, 1.000000000000000000, 0.8660254037844387076, 1.000000000000000000, 0.8660254037844387076, 1.000000000000000000, 0.8660254037844387076, 1.000000000000000000, 0.8660254037844387076, 1.000000000000000000, 0.8660254037844387076, 1.000000000000000000, 0.8660254037844387076, 1.000000000000000000, 0.8660254037844387076, 1.000000000000000000, 0.8660254037844387076, 1.000000000000000000, 0.8660254037844387076, 1.000000000000000000, 0.8660254037844387076, 1.000000000000000000, 0.8660254037844387076, 1.000000000000000000, 0.8660254037844387076, 1.000000000000000000, 0.8660254037844387076, 1.000000000000000000, 0.8660254037844387076, 1.000000000000000000, 0.8660254037844387076, 1.000000000000000000, 0.8660254037844387076, 1.000000000000000000, 0.8660254037844387076, 1.000000000000000000, 0.8660254037844387076, 1.000000000000000000, 0.8660254037844387076, 1.000000000000000000, 0.8660254037844387076, 1.000000000000000000, 0.8660254037844387076, 1.000000000000000000, 0.8660254037844387076, 1.000000000000000000, 0.8660254037844387076, 1.000000000000000000, 0.9548847663035771038, 0.9401541632606846832),
 ( 1.000000000000000000, 0.8660254037844387076, 1.000000000000000000, 0.8660254037844387076, 1.000000000000000000, 0.8660254037844387076, 1.000000000000000000, 0.8660254037844387076, 1.000000000000000000, 0.8660254037844387076, 1.000000000000000000, 0.8660254037844387076, 1.000000000000000000, 0.8660254037844387076, 1.000000000000000000, 0.8660254037844387076, 1.000000000000000000, 0.8660254037844387076, 1.000000000000000000, 0.8660254037844387076, 1.000000000000000000, 0.8660254037844387076, 1.000000000000000000, 0.8660254037844387076, 1.000000000000000000, 0.8660254037844387076, 1.000000000000000000, 0.8660254037844387076, 1.000000000000000000, 0.8660254037844387076, 1.000000000000000000, 0.8660254037844387076, 1.000000000000000000, 0.8660254037844387076, 1.000000000000000000, 0.8660254037844387076, 1.000000000000000000, 0.8660254037844387076, 1.000000000000000000, 0.8660254037844387076, 1.000000000000000000, 0.8660254037844387076, 1.000000000000000000, 0.8660254037844387076, 1.000000000000000000, 0.8660254037844387076, 1.000000000000000000, 0.8660254037844387076, 1.000000000000000000, 0.8660254037844387076, 1.000000000000000000, 0.8660254037844387076, 1.000000000000000000, 0.8660254037844387076, 1.000000000000000000, 0.8660254037844387076, 1.000000000000000000, 0.8660254037844387076, 1.000000000000000000, 0.8660254037844387076, 1.000000000000000000, 0.8660254037844387076, 1.000000000000000000, 0.8660254037844387076, 1.000000000000000000, 0.8660254037844387076, 1.000000000000000000, 0.8660254037844387076, 1.000000000000000000, 0.8660254037844387076, 1.000000000000000000, 0.8660254037844387076, 1.000000000000000000, 0.8660254037844387076, 1.000000000000000000, 0.8660254037844387076, 1.000000000000000000, 0.8660254037844387076, 1.000000000000000000, 0.8660254037844387076, 1.000000000000000000, 0.8660254037844387076, 1.000000000000000000, 0.8660254037844387076, 1.000000000000000000, 0.8660254037844387076, 1.000000000000000000, 0.8660254037844387076, 1.000000000000000000, 0.8660254037844387076, 1.000000000000000000, 0.8660254037844387076, 1.000000000000000000, 0.8660254037844387076, 1.000000000000000000, 0.8660254037844387076, 1.000000000000000000, 0.8660254037844387076, 1.000000000000000000, 0.8660254037844387076, 1.000000000000000000, 0.8660254037844387076, 1.000000000000000000, 0.8660254037844387076, 1.000000000000000000, 0.8660254037844387076, 1.000000000000000000, 0.8660254037844387076, 1.000000000000000000, 0.8660254037844387076, 1.000000000000000000, 0.8660254037844387076, 1.000000000000000000, 0.8660254037844387076, 1.000000000000000000, 0.8660254037844387076, 1.000000000000000000, 0.8660254037844387076, 1.000000000000000000, 0.8660254037844387076, 1.000000000000000000, 0.8660254037844387076, 1.000000000000000000, 0.8660254037844387076, 1.000000000000000000, 0.8660254037844387076, 1.000000000000000000, 0.8660254037844387076, 1.000000000000000000, 0.8660254037844387076, 1.000000000000000000, 0.8660254037844387076, 1.000000000000000000, 0.8660254037844387076, 1.000000000000000000, 0.8660254037844387076, 1.000000000000000000, 0.8660254037844387076, 1.000000000000000000, 0.8660254037844387076, 1.000000000000000000, 0.8660254037844387076, 1.000000000000000000, 0.8660254037844387076, 1.000000000000000000, 0.8660254037844387076, 1.000000000000000000, 0.8660254037844387076, 1.000000000000000000, 0.8660254037844387076, 1.000000000000000000, 0.8660254037844387076, 1.000000000000000000, 0.8660254037844387076, 1.000000000000000000, 0.8660254037844387076, 1.000000000000000000, 0.8660254037844387076, 1.000000000000000000, 0.8660254037844387076, 1.000000000000000000, 0.8660254037844387076, 1.000000000000000000, 0.8660254037844387076, 1.000000000000000000, 0.8660254037844387076, 1.000000000000000000, 0.8660254037844387076, 1.000000000000000000, 0.8660254037844387076, 1.000000000000000000, 0.8660254037844387076, 1.000000000000000000, 0.8660254037844387076, 1.000000000000000000, 0.8660254037844387076, 1.000000000000000000, 0.8660254037844387076, 1.000000000000000000, 0.8660254037844387076, 1.000000000000000000, 0.8660254037844387076, 1.000000000000000000, 0.8660254037844387076, 1.000000000000000000, 0.8660254037844387076, 1.000000000000000000, 0.8660254037844387076, 1.000000000000000000, 0.8660254037844387076, 1.000000000000000000, 0.8660254037844387076, 1.000000000000000000, 0.8660254037844387076, 1.000000000000000000, 0.8660254037844387076, 1.000000000000000000, 0.8660254037844387076, 1.000000000000000000, 0.8660254037844387076, 1.000000000000000000, 0.8660254037844387076, 1.000000000000000000, 0.8660254037844387076, 1.000000000000000000, 0.8660254037844387076, 1.000000000000000000, 0.8660254037844387076, 1.000000000000000000, 0.8660254037844387076, 1.000000000000000000, 0.8660254037844387076, 1.000000000000000000, 0.8660254037844387076, 1.000000000000000000, 0.8660254037844387076, 1.000000000000000000, 0.8660254037844387076, 1.000000000000000000, 0.8660254037844387076, 1.000000000000000000, 0.8660254037844387076, 1.000000000000000000, 0.8660254037844387076, 1.000000000000000000, 0.8660254037844387076, 1.000000000000000000, 0.8660254037844387076, 1.000000000000000000, 0.8660254037844387076, 1.000000000000000000, 0.8660254037844387076, 1.000000000000000000, 0.8660254037844387076, 1.000000000000000000, 0.8660254037844387076, 1.000000000000000000, 0.8660254037844387076, 1.000000000000000000, 0.8660254037844387076, 1.000000000000000000, 0.8660254037844387076, 1.000000000000000000, 0.8660254037844387076, 1.000000000000000000, 0.8660254037844387076, 1.000000000000000000, 0.8660254037844387076, 1.000000000000000000, 0.8660254037844387076, 1.000000000000000000, 0.8660254037844387076, 1.000000000000000000, 0.8660254037844387076, 1.000000000000000000, 0.8660254037844387076, 1.000000000000000000, 0.8660254037844387076, 1.000000000000000000, 0.8660254037844387076, 1.000000000000000000, 0.8660254037844387076, 1.000000000000000000, 0.8660254037844387076, 1.000000000000000000, 0.8660254037844387076, 1.000000000000000000, 0.9548847663035771038, 0.9401541632606846832) ) ) 
 REPRESENTATION_ITEM ( '' )  SURFACE ( )  );
#33976=CYLINDRICAL_SURFACE ( 'NONE', #29678, 5.999999999999994671 ) ;
#34006=CARTESIAN_POINT ( 'NONE',  ( 37.09755260828975310, 7.646167579472015790E-16, 162.3589405374562205 ) ) ;
#34007=CARTESIAN_POINT ( 'NONE',  ( 26.75643035624999655, -3.323476615752267715, -0.9656249993854794100 ) ) ;
#34009=VERTEX_POINT ( 'NONE', #25241 ) ;
#34012=CARTESIAN_POINT ( 'NONE',  ( 15.00000000000000178, -3.464101615137757051, -5.756249998770938348 ) ) ;
#34013=CARTESIAN_POINT ( 'NONE',  ( 23.87821517812500005, -4.985214923628404016, -1.790624999385481697 ) ) ;
#34016=DIRECTION ( 'NONE',  ( 0.08715574274765150453, 0.000000000000000000, 0.9961946980917461003 ) ) ;
#34019=EDGE_CURVE ( 'NONE', #18997, #36867, #1555, .T. ) ;
#34025=CARTESIAN_POINT ( 'NONE',  ( 36.99789971106883257, 3.464101615137755275, 164.0145509578369740 ) ) ;
#34031=CARTESIAN_POINT ( 'NONE',  ( 26.75643035624999655, -3.323476615752267271, -1.865624999385470772 ) ) ;
#34040=CARTESIAN_POINT ( 'NONE',  ( 33.98928129033111389, 5.407089921784862696, 162.6497006628943041 ) ) ;
#34045=CARTESIAN_POINT ( 'NONE',  ( 20.99999999999999645, -6.928203230275506996, -3.487500000000006928 ) ) ;
#34054=VERTEX_POINT ( 'NONE', #19571 ) ;
#34055=CARTESIAN_POINT ( 'NONE',  ( 21.00000000000000000, 6.928203230275506996, -4.612499999999980282 ) ) ;
#34057=CARTESIAN_POINT ( 'NONE',  ( 30.64732363713033081, 7.209453229046482114, 160.2694137540738950 ) ) ;
#34059=CARTESIAN_POINT ( 'NONE',  ( 31.43662783238875136, 7.209453229046475009, 169.2912019886672681 ) ) ;
#34068=CARTESIAN_POINT ( 'NONE',  ( 15.24356964374999990, 0.000000000000000000, -8.353124999385480365 ) ) ;
#34071=CARTESIAN_POINT ( 'NONE',  ( 37.34434378849091019, -3.464101615137651358, 167.9744248827516913 ) ) ;
#34082=CARTESIAN_POINT ( 'NONE',  ( 33.95496371662422064, 5.407089921784857367, 162.2574490005206655 ) ) ;
#34088=VECTOR ( 'NONE', #27414, 1000.000000000000000 ) ;
#34094=CARTESIAN_POINT ( 'NONE',  ( 24.64158895398392701, -3.604726614523240613, 163.2604799309594625 ) ) ;
#34095=CARTESIAN_POINT ( 'NONE',  ( 15.24356964375000167, -3.323476615752272600, -6.403124999385489069 ) ) ;
#34097=CARTESIAN_POINT ( 'NONE',  ( 31.27484498491342890, 7.209453229046482114, 167.4420155803344699 ) ) ;
#34098=CARTESIAN_POINT ( 'NONE',  ( 34.22502607998692525, -5.196152422706635576, 166.7416000626326422 ) ) ;
#34101=CARTESIAN_POINT ( 'NONE',  ( 31.02726820322443047, 6.928203230275506996, 164.6122000166797932 ) ) ;
#34104=VERTEX_POINT ( 'NONE', #30572 ) ;
#34106=LINE ( 'NONE', #5295, #24978 ) ;
#34107=CARTESIAN_POINT ( 'NONE',  ( 15.24356964374999990, 0.000000000000000000, -3.290624999385455496 ) ) ;
#34110=CARTESIAN_POINT ( 'NONE',  ( 23.87821517812499650, 4.985214923628404904, -2.653124999385497951 ) ) ;
#34133=ORIENTED_EDGE ( 'NONE', *, *, #36505, .T. ) ;
#34145=CARTESIAN_POINT ( 'NONE',  ( 18.00000000000000355, -5.196152422706632912, -8.924999999999988276 ) ) ;
#34150=CARTESIAN_POINT ( 'NONE',  ( 26.75643035624999655, 7.049594010296217766E-16, -6.328124999385481786 ) ) ;
#34160=CARTESIAN_POINT ( 'NONE',  ( 34.39171143809891618, -5.196152422706629359, 168.6468224239574454 ) ) ;
#34194=CARTESIAN_POINT ( 'NONE',  ( 24.59910052939444824, 0.000000000000000000, 162.7748350156397521 ) ) ;
#34201=CARTESIAN_POINT ( 'NONE',  ( 26.99999999999999645, -3.464101615137751278, -4.706249998770958953 ) ) ;
#34202=CARTESIAN_POINT ( 'NONE',  ( 18.12178482187499640, 4.985214923628404904, -3.365624999385474769 ) ) ;
#34203=CARTESIAN_POINT ( 'NONE',  ( 23.99999999999999645, 5.196152422706631135, -6.450000000000011724 ) ) ;
#34204=CARTESIAN_POINT ( 'NONE',  ( 34.26424616422337266, -5.196152422706635576, 167.1898876767739353 ) ) ;
#34211=CARTESIAN_POINT ( 'NONE',  ( 33.97336387291019122, 5.196152422706631135, 163.8650878731170906 ) ) ;
#34216=CARTESIAN_POINT ( 'NONE',  ( 23.87821517812499650, 4.985214923628404904, -4.003124999385487826 ) ) ;
#34220=ORIENTED_EDGE ( 'NONE', *, *, #29725, .F. ) ;
#34225=LINE ( 'NONE', #5226, #12619 ) ;
#34226=CARTESIAN_POINT ( 'NONE',  ( 24.59419801886489054, 0.000000000000000000, 162.7187990638720976 ) ) ;
#34228=EDGE_CURVE ( 'NONE', #31223, #31993, #11053, .T. ) ;
#34231=CARTESIAN_POINT ( 'NONE',  ( 18.00000000000000000, 5.196152422706630247, -4.124999999999989342 ) ) ;
#34241=CARTESIAN_POINT ( 'NONE',  ( 23.99999999999999645, 5.196152422706631135, -4.200000000000009059 ) ) ;
#34243=CARTESIAN_POINT ( 'NONE',  ( 37.14824336730885079, -3.464101615137567869, 165.7329868120451692 ) ) ;
#34244=CARTESIAN_POINT ( 'NONE',  ( 24.51575785039200284, 0.000000000000000000, 161.8222238355895399 ) ) ;
#34246=CARTESIAN_POINT ( 'NONE',  ( 37.56819361912707222, 7.646167579472015790E-16, 167.7383919071516516 ) ) ;
#34255=CARTESIAN_POINT ( 'NONE',  ( 26.75643035624999655, 7.049594010296217766E-16, -8.128124999385477167 ) ) ;
#34259=CARTESIAN_POINT ( 'NONE',  ( 23.99999999999999645, 5.196152422706631135, -6.393749998770958953 ) ) ;
#34260=CARTESIAN_POINT ( 'NONE',  ( 37.09591843811324452, 3.604726614523243278, 162.3402618868670118 ) ) ;
#34271=CARTESIAN_POINT ( 'NONE',  ( 37.64499961742345135, 3.604726614523243278, 168.6162884848450005 ) ) ;
#34273=CARTESIAN_POINT ( 'NONE',  ( 26.99999999999999645, 7.347880794884117764E-16, -0.6187499987709565996 ) ) ;
#34284=CARTESIAN_POINT ( 'NONE',  ( 30.76988640036921652, 7.209453229046475009, 161.6703125482654286 ) ) ;
#34285=CARTESIAN_POINT ( 'NONE',  ( 15.24356964375000167, -3.323476615752272600, -7.753124999385476279 ) ) ;
#34287=CARTESIAN_POINT ( 'NONE',  ( 28.18128119854344860, -5.407089921784865361, 167.9008835610755455 ) ) ;
#34289=CARTESIAN_POINT ( 'NONE',  ( 25.28868886033853158, -3.464101615137761048, 167.8622174579674606 ) ) ;
#34295=ORIENTED_EDGE ( 'NONE', *, *, #5154, .T. ) ;
#34301=CARTESIAN_POINT ( 'NONE',  ( 26.75643035624999655, -3.323476615752267715, -1.415624999385507232 ) ) ;
#34319=CARTESIAN_POINT ( 'NONE',  ( 27.88507211235645400, 5.196152422706630247, 163.1178740895360306 ) ) ;
#34321=CARTESIAN_POINT ( 'NONE',  ( 37.61068204371655099, 3.604726614523238837, 168.2240368224713620 ) ) ;
#34323=CARTESIAN_POINT ( 'NONE',  ( 15.24356964375000167, -3.323476615752272600, -0.5531249993854806535 ) ) ;
#34331=CARTESIAN_POINT ( 'NONE',  ( 24.00000000000000000, -5.196152422706629359, -8.849999999999996092 ) ) ;
#34332=ORIENTED_EDGE ( 'NONE', *, *, #751, .F. ) ;
#34336=CARTESIAN_POINT ( 'NONE',  ( 15.24356964375000167, -3.323476615752272600, -10.11562499938547788 ) ) ;
#34338=EDGE_LOOP ( 'NONE', ( #33737, #9738, #21351, #10097 ) ) ;
#34343=CARTESIAN_POINT ( 'NONE',  ( 31.23562490067698150, 7.209453229046482114, 166.9937279661931768 ) ) ;
#34364=CARTESIAN_POINT ( 'NONE',  ( 36.87043443719270641, 3.464101615138096335, 162.5576162106535492 ) ) ;
#34373=ORIENTED_EDGE ( 'NONE', *, *, #16773, .F. ) ;
#34380=CARTESIAN_POINT ( 'NONE',  ( 36.98316069593346356, 3.604726614523238837, 161.0514349962108156 ) ) ;
#34381=CARTESIAN_POINT ( 'NONE',  ( 33.91126540609537443, -5.196152422706635576, 163.1552991495023548 ) ) ;
#34386=CARTESIAN_POINT ( 'NONE',  ( 23.99999999999999645, 5.196152422706631135, -7.293749998770943321 ) ) ;
#34387=CARTESIAN_POINT ( 'NONE',  ( 15.24356964374999990, 0.000000000000000000, -3.740624999385461003 ) ) ;
#34388=CARTESIAN_POINT ( 'NONE',  ( 33.58116303054575269, 5.196152422706631135, 159.3822117317042455 ) ) ;
#34391=EDGE_CURVE ( 'NONE', #30763, #23933, #18612, .T. ) ;
#34398=CARTESIAN_POINT ( 'NONE',  ( 30.92921799263331906, -6.928203230275506996, 163.4914809813265606 ) ) ;
#34401=( BOUNDED_CURVE ( )  B_SPLINE_CURVE ( 2, ( #14844, #424, #11990, #23562, #35107, #9155, #20722 ),
 .UNSPECIFIED., .F., .F. ) 
 B_SPLINE_CURVE_WITH_KNOTS ( ( 3, 2, 2, 3 ),
 ( 0.000000000000000000, 0.007246376811594097168, 0.01449275362318819434, 0.02173913043478229237 ),
 .UNSPECIFIED. ) 
 CURVE ( )  GEOMETRIC_REPRESENTATION_ITEM ( )  RATIONAL_B_SPLINE_CURVE ( ( 1.000000000000000000, 0.8660254037844387076, 1.000000000000000000, 0.8660254037844387076, 1.000000000000000000, 0.8660254037844445918, 0.9999999999999941158 ) ) 
 REPRESENTATION_ITEM ( '' )  );
#34403=CARTESIAN_POINT ( 'NONE',  ( 20.99999999999999645, 6.646953231504538984, -3.965624999385493510 ) ) ;
#34404=CYLINDRICAL_SURFACE ( 'NONE', #5870, 5.999999999999994671 ) ;
#34407=VERTEX_POINT ( 'NONE', #36007 ) ;
#34412=CARTESIAN_POINT ( 'NONE',  ( 24.59746635921792546, -3.604726614523244610, 162.7561563650505150 ) ) ;
#34425=VERTEX_POINT ( 'NONE', #26537 ) ;
#34426=CARTESIAN_POINT ( 'NONE',  ( 26.99999999999999645, 3.464101615137755275, -3.787500000000015188 ) ) ;
#34428=CARTESIAN_POINT ( 'NONE',  ( 33.70166733926387082, -5.407089921784861808, 159.3622581591915548 ) ) ;
#34430=CARTESIAN_POINT ( 'NONE',  ( 31.33857762179763995, -7.209453229046475009, 168.1704829533140355 ) ) ;
#34434=ORIENTED_EDGE ( 'NONE', *, *, #36268, .T. ) ;
#34435=ORIENTED_EDGE ( 'NONE', *, *, #22237, .F. ) ;
#34439=CARTESIAN_POINT ( 'NONE',  ( 15.24356964375000167, -3.323476615752272600, -9.215624999385486404 ) ) ;
#34443=EDGE_CURVE ( 'NONE', #805, #8055, #9304, .T. ) ;
#34444=CARTESIAN_POINT ( 'NONE',  ( 36.97825818540390941, 3.604726614523243278, 160.9953990444431611 ) ) ;
#34455=CARTESIAN_POINT ( 'NONE',  ( 33.75886329544200493, 5.407089921784857367, 160.0160109298142288 ) ) ;
#34456=CARTESIAN_POINT ( 'NONE',  ( 15.00000000000000000, 0.000000000000000000, -2.193749998770949894 ) ) ;
#34457=( BOUNDED_CURVE ( )  B_SPLINE_CURVE ( 2, ( #27283, #3780, #35620, #21243, #1313, #30320, #3600 ),
 .UNSPECIFIED., .F., .F. ) 
 B_SPLINE_CURVE_WITH_KNOTS ( ( 3, 2, 2, 3 ),
 ( 0.3695652173913039351, 0.3768115942028982257, 0.3840579710144925163, 0.3913043478260868069 ),
 .UNSPECIFIED. ) 
 CURVE ( )  GEOMETRIC_REPRESENTATION_ITEM ( )  RATIONAL_B_SPLINE_CURVE ( ( 1.000000000000007105, 0.8660254037844313801, 1.000000000000000000, 0.8660254037844387076, 1.000000000000000000, 0.8660254037844418162, 0.9999999999999968914 ) ) 
 REPRESENTATION_ITEM ( '' )  );
#34466=CARTESIAN_POINT ( 'NONE',  ( 24.63505227327785718, 3.604726614523236616, 163.1857653286025709 ) ) ;
#34467=CARTESIAN_POINT ( 'NONE',  ( 23.87821517812499650, 4.985214923628404904, -7.040624999385459049 ) ) ;
#34469=CARTESIAN_POINT ( 'NONE',  ( 37.48811928047767594, 3.604726614523243278, 166.8231380282798568 ) ) ;
#34470=CARTESIAN_POINT ( 'NONE',  ( 31.27239372959508756, -6.928203230275514990, 167.4139976038384532 ) ) ;
#34477=ORIENTED_EDGE ( 'NONE', *, *, #30400, .F. ) ;
#34484=CARTESIAN_POINT ( 'NONE',  ( 18.12178482187500350, -4.985214923628407568, -2.428124999385494753 ) ) ;
#34499=CARTESIAN_POINT ( 'NONE',  ( 15.00000000000000000, 0.000000000000000000, -0.4500000000000059508 ) ) ;
#34505=ORIENTED_EDGE ( 'NONE', *, *, #33218, .F. ) ;
#34506=CARTESIAN_POINT ( 'NONE',  ( 34.53019161875872101, -5.407089921784855591, 168.8323340079261925 ) ) ;
#34508=CARTESIAN_POINT ( 'NONE',  ( 18.12178482187500350, -4.985214923628407568, -0.5156249993854555846 ) ) ;
#34509=CARTESIAN_POINT ( 'NONE',  ( 20.99999999999999645, 6.928203230275506996, -5.062500000000007994 ) ) ;
#34510=DIRECTION ( 'NONE',  ( 1.000000000000000000, 0.000000000000000000, 0.000000000000000000 ) ) ;
#34516=ORIENTED_EDGE ( 'NONE', *, *, #15497, .F. ) ;
#34517=ORIENTED_EDGE ( 'NONE', *, *, #24524, .F. ) ;
#34522=CARTESIAN_POINT ( 'NONE',  ( 21.00000000000000000, 6.646953231504538984, -0.2531249993854407521 ) ) ;
#34524=( BOUNDED_CURVE ( )  B_SPLINE_CURVE ( 2, ( #17853, #11083, #11271, #31360, #32426, #11961, #31182 ),
 .UNSPECIFIED., .F., .F. ) 
 B_SPLINE_CURVE_WITH_KNOTS ( ( 3, 2, 2, 3 ),
 ( 0.06521739130434729692, 0.07246376811594164302, 0.07971014492753598912, 0.08695652173913033522 ),
 .UNSPECIFIED. ) 
 CURVE ( )  GEOMETRIC_REPRESENTATION_ITEM ( )  RATIONAL_B_SPLINE_CURVE ( ( 1.000000000000009770, 0.8660254037844290487, 1.000000000000000000, 0.8660254037844387076, 1.000000000000000000, 0.8660254037844404840, 0.9999999999999982236 ) ) 
 REPRESENTATION_ITEM ( '' )  );
#34525=ORIENTED_EDGE ( 'NONE', *, *, #26272, .F. ) ;
#34528=CARTESIAN_POINT ( 'NONE',  ( 24.94717877699287811, 0.000000000000000000, 166.7533875911436780 ) ) ;
#34529=AXIS2_PLACEMENT_3D ( 'NONE', #11762, #22961, #14983 ) ;
#34535=CARTESIAN_POINT ( 'NONE',  ( 37.60741370336351252, 7.646167579472015790E-16, 168.1866795212929446 ) ) ;
#34538=CARTESIAN_POINT ( 'NONE',  ( 18.00000000000000355, -5.196152422706632912, -7.124999999999992895 ) ) ;
#34562=CARTESIAN_POINT ( 'NONE',  ( 24.52392870127459545, -3.604726614523240613, 161.9156170885356403 ) ) ;
#34563=CARTESIAN_POINT ( 'NONE',  ( 26.75643035624999655, -3.323476615752267715, -1.865624999385470772 ) ) ;
#34568=ORIENTED_EDGE ( 'NONE', *, *, #1070, .T. ) ;
#34569=CARTESIAN_POINT ( 'NONE',  ( 15.00000000000000178, -3.464101615137757051, -6.656249998770961795 ) ) ;
#34570=CARTESIAN_POINT ( 'NONE',  ( 20.99999999999999645, -6.646953231504538984, -1.828124999385473792 ) ) ;
#34578=CARTESIAN_POINT ( 'NONE',  ( 27.76741185964712244, 5.196152422706630247, 161.7730112471121799 ) ) ;
#34582=CARTESIAN_POINT ( 'NONE',  ( 20.99999999999999645, -6.646953231504538984, -5.090624999385466865 ) ) ;
#34590=CARTESIAN_POINT ( 'NONE',  ( 26.99999999999962341, 3.464101615137969770, -5.981249998770948650 ) ) ;
#34591=CARTESIAN_POINT ( 'NONE',  ( 34.01542801315541453, -5.407089921784861808, 162.9485590723218422 ) ) ;
#34596=EDGE_CURVE ( 'NONE', #34054, #972, #26323, .T. ) ;
#34603=ORIENTED_EDGE ( 'NONE', *, *, #8492, .F. ) ;
#34604=CARTESIAN_POINT ( 'NONE',  ( 18.00000000000000000, 5.196152422706630247, -4.574999999999995737 ) ) ;
#34606=CARTESIAN_POINT ( 'NONE',  ( 33.74088742350031822, -5.407089921784861808, 159.8105457733328478 ) ) ;
#34608=CARTESIAN_POINT ( 'NONE',  ( 31.41701779027052766, -7.209453229046475009, 169.0670581815966216 ) ) ;
#34614=EDGE_LOOP ( 'NONE', ( #10059, #860, #28371, #10972 ) ) ;
#34616=CARTESIAN_POINT ( 'NONE',  ( 26.99999999999999645, 7.347880794884117764E-16, -5.118749998770960374 ) ) ;
#34618=CARTESIAN_POINT ( 'NONE',  ( 19.00081547855239350, 5.492723509887031952, -10.23957780870842882 ) ) ;
#34621=EDGE_CURVE ( 'NONE', #11581, #16861, #26771, .T. ) ;
#34623=CARTESIAN_POINT ( 'NONE',  ( 24.51575785039200284, 0.000000000000000000, 161.8222238355895399 ) ) ;
#34626=PRODUCT_CONTEXT ( 'NONE', #19249, 'mechanical' ) ;
#34634=CARTESIAN_POINT ( 'NONE',  ( 27.54558899987776144, 5.407089921784856479, 160.6348884818688418 ) ) ;
#34635=CARTESIAN_POINT ( 'NONE',  ( 15.00000000000000178, -3.464101615137757051, -2.606249998770968190 ) ) ;
#34645=CARTESIAN_POINT ( 'NONE',  ( 33.86345018673919327, -5.407089921784855591, 161.2114445675243530 ) ) ;
#34646=CARTESIAN_POINT ( 'NONE',  ( 23.87821517812500005, -4.985214923628404016, -7.640624999385475569 ) ) ;
#34648=EDGE_CURVE ( 'NONE', #2079, #3146, #9623, .T. ) ;
#34649=CARTESIAN_POINT ( 'NONE',  ( 31.21601485855875779, -7.209453229046482114, 166.7695841591225587 ) ) ;
#34650=CARTESIAN_POINT ( 'NONE',  ( 37.25936693920468201, 7.347880794884125653E-16, 167.0031350508878631 ) ) ;
#34657=ORIENTED_EDGE ( 'NONE', *, *, #16103, .T. ) ;
#34664=CARTESIAN_POINT ( 'NONE',  ( 23.87821517812499650, 4.985214923628404904, -3.553124999385481875 ) ) ;
#34686=CARTESIAN_POINT ( 'NONE',  ( 37.56492527877403376, -3.604726614523235284, 167.7010346059732058 ) ) ;
#34690=FACE_OUTER_BOUND ( 'NONE', #25086, .T. ) ;
#34691=CARTESIAN_POINT ( 'NONE',  ( 18.00000000000000000, 5.196152422706630247, -2.774999999999999467 ) ) ;
#34702=CARTESIAN_POINT ( 'NONE',  ( 15.24356964374999990, 3.323476615752268604, -9.290624999385480365 ) ) ;
#34707=CARTESIAN_POINT ( 'NONE',  ( 37.48811928047766884, 3.604726614523243278, 166.8231380282798568 ) ) ;
#34716=CARTESIAN_POINT ( 'NONE',  ( 25.37039736927151878, 3.464101615137721524, 168.7961499886528713 ) ) ;
#34719=CARTESIAN_POINT ( 'NONE',  ( 23.99999999999999645, 5.196152422706631135, -1.443749998770949006 ) ) ;
#34722=( GEOMETRIC_REPRESENTATION_CONTEXT ( 3 ) GLOBAL_UNCERTAINTY_ASSIGNED_CONTEXT ( ( #15321 ) ) GLOBAL_UNIT_ASSIGNED_CONTEXT ( ( #32625, #23920, #18237 ) ) REPRESENTATION_CONTEXT ( 'NONE', 'WORKASPACE' ) );
#34732=CARTESIAN_POINT ( 'NONE',  ( 25.29522554115172639, 0.000000000000000000, 167.9369320615487311 ) ) ;
#34737=( BOUNDED_CURVE ( )  B_SPLINE_CURVE ( 2, ( #11142, #10953, #28747, #16656, #25176, #8306, #31235 ),
 .UNSPECIFIED., .F., .F. ) 
 B_SPLINE_CURVE_WITH_KNOTS ( ( 3, 2, 2, 3 ),
 ( 0.3913043478260864738, 0.3985507246376804869, 0.4057971014492746109, 0.4130434782608686239 ),
 .UNSPECIFIED. ) 
 CURVE ( )  GEOMETRIC_REPRESENTATION_ITEM ( )  RATIONAL_B_SPLINE_CURVE ( ( 1.000000000000009326, 0.8660254037844296038, 1.000000000000000000, 0.8660254037844387076, 1.000000000000000000, 0.8660254037844561381, 0.9999999999999825695 ) ) 
 REPRESENTATION_ITEM ( '' )  );
#34740=CARTESIAN_POINT ( 'NONE',  ( 24.81804784950163878, -3.464101615138005741, 162.4827660882720295 ) ) ;
#34748=CARTESIAN_POINT ( 'NONE',  ( 36.89818384675449892, -3.604726614523235284, 160.0801451655713663 ) ) ;
#34749=CARTESIAN_POINT ( 'NONE',  ( 18.12178482187499640, 4.985214923628404904, -1.678124999385494087 ) ) ;
#34752=ORIENTED_EDGE ( 'NONE', *, *, #22237, .T. ) ;
#34755=CARTESIAN_POINT ( 'NONE',  ( 15.24356964374999990, 0.000000000000000000, -4.640624999385472904 ) ) ;
#34765=CARTESIAN_POINT ( 'NONE',  ( 30.88999790839687876, -6.928203230275506996, 163.0431933671852676 ) ) ;
#34769=CARTESIAN_POINT ( 'NONE',  ( 15.24356964374999990, 0.000000000000000000, -3.403124999385470417 ) ) ;
#34770=CARTESIAN_POINT ( 'NONE',  ( 18.00000000000000355, -5.196152422706632912, -1.725000000000004308 ) ) ;
#34773=EDGE_LOOP ( 'NONE', ( #4321, #5253, #7764, #37032 ) ) ;
#34777=CARTESIAN_POINT ( 'NONE',  ( 36.93576976081443775, 7.646167579472024665E-16, 160.5097541291234506 ) ) ;
#34786=CARTESIAN_POINT ( 'NONE',  ( 23.99999999999999645, 5.196152422706631135, -7.743749998770948828 ) ) ;
#34789=ORIENTED_EDGE ( 'NONE', *, *, #25867, .F. ) ;
#34790=CARTESIAN_POINT ( 'NONE',  ( 23.99999999999999645, 5.196152422706631135, -5.549999999999998934 ) ) ;
#34794=CARTESIAN_POINT ( 'NONE',  ( 34.33409119757650529, -5.407089921784855591, 166.5908959372197558 ) ) ;
#34796=CARTESIAN_POINT ( 'NONE',  ( 27.00000000000041567, 3.464101615137513690, -1.031249998770972454 ) ) ;
#34802=CARTESIAN_POINT ( 'NONE',  ( 23.87821517812500005, -4.985214923628404016, -7.190624999385470062 ) ) ;
#34808=CARTESIAN_POINT ( 'NONE',  ( 25.40961745350801948, 3.464101615137752166, 169.2444376027941360 ) ) ;
#34821=CARTESIAN_POINT ( 'NONE',  ( 25.14001085782205891, 3.604726614523240613, 168.9574683606716690 ) ) ;
#34822=CARTESIAN_POINT ( 'NONE',  ( 18.00000000000000000, 5.196152422706630247, -1.818749998770963217 ) ) ;
#34833=CARTESIAN_POINT ( 'NONE',  ( 33.91574363238778034, 5.407089921784857367, 161.8091613863793725 ) ) ;
#34835=CARTESIAN_POINT ( 'NONE',  ( 15.24356964374999990, 3.323476615752268604, -8.278124999385466865 ) ) ;
#34837=CARTESIAN_POINT ( 'NONE',  ( 37.32470226282583781, -3.604726614523238837, 164.9552729693578215 ) ) ;
#34838=CARTESIAN_POINT ( 'NONE',  ( 28.26746793355466281, 5.196152422706636465, 167.4886783261892162 ) ) ;
#34842=EDGE_CURVE ( 'NONE', #4816, #941, #15934, .T. ) ;
#34846=ORIENTED_EDGE ( 'NONE', *, *, #29725, .T. ) ;
#34847=ORIENTED_EDGE ( 'NONE', *, *, #33928, .F. ) ;
#34851=CARTESIAN_POINT ( 'NONE',  ( 15.24356964374999990, 3.323476615752268604, -3.890624999385467575 ) ) ;
#34862=VECTOR ( 'NONE', #21844, 1000.000000000000000 ) ;
#34865=CARTESIAN_POINT ( 'NONE',  ( 36.67433401601032017, 3.464101615138187817, 160.3161781399470840 ) ) ;
#34875=ORIENTED_EDGE ( 'NONE', *, *, #25253, .F. ) ;
#34876=CARTESIAN_POINT ( 'NONE',  ( 28.25155051613373658, 5.407089921784856479, 168.7040655364119743 ) ) ;
#34878=CARTESIAN_POINT ( 'NONE',  ( 15.24356964375000167, -3.323476615752272600, -1.003124999385444527 ) ) ;
#34887=EDGE_LOOP ( 'NONE', ( #26783, #24100, #10138, #25447 ) ) ;
#34892=CARTESIAN_POINT ( 'NONE',  ( 26.75643035624999655, 7.049594010296217766E-16, -8.578124999385483562 ) ) ;
#34897=VERTEX_POINT ( 'NONE', #30330 ) ;
#34898=CARTESIAN_POINT ( 'NONE',  ( 25.06810737005524459, -3.604726614523244610, 168.1356077347459461 ) ) ;
#34906=CARTESIAN_POINT ( 'NONE',  ( 31.31896757967941625, 7.209453229046475009, 167.9463391462434174 ) ) ;
#34907=ORIENTED_EDGE ( 'NONE', *, *, #15614, .F. ) ;
#34919=CARTESIAN_POINT ( 'NONE',  ( 26.99999999999967670, 3.464101615137938683, -1.537500000000000311 ) ) ;
#34921=CARTESIAN_POINT ( 'NONE',  ( 34.20868437832884013, 5.196152422706631135, 166.5548135579648488 ) ) ;
#34922=CARTESIAN_POINT ( 'NONE',  ( 37.30512370425449120, -3.464101615137641144, 167.5261372686103698 ) ) ;
#34932=CARTESIAN_POINT ( 'NONE',  ( 23.87821517812500005, -4.985214923628404016, -2.803124999385481431 ) ) ;
#34937=CARTESIAN_POINT ( 'NONE',  ( 26.75643035624999655, 7.049594010296217766E-16, -5.315624999385482496 ) ) ;
#34946=CARTESIAN_POINT ( 'NONE',  ( 30.83116778204221475, 6.928203230275506996, 162.3707619459733564 ) ) ;
#34950=EDGE_CURVE ( 'NONE', #6148, #20636, #17604, .T. ) ;
#34951=CARTESIAN_POINT ( 'NONE',  ( 20.99999999999999645, 6.646953231504538984, -3.515624999385498217 ) ) ;
#34955=ORIENTED_EDGE ( 'NONE', *, *, #5536, .T. ) ;
#34956=CARTESIAN_POINT ( 'NONE',  ( 26.99999999999999645, 7.347880794884117764E-16, -0.6187499987709565996 ) ) ;
#34959=FACE_OUTER_BOUND ( 'NONE', #6692, .T. ) ;
#34960=( BOUNDED_SURFACE ( )  B_SPLINE_SURFACE ( 1, 2, ( 
 ( #19440, #33640, #14109, #25661, #36844, #10887, #22833, #13550, #25103, #13746, #4821, #22276, #7679, #16402, #27948, #2163, #33829, #30990, #22460, #34007, #31535, #26212, #6319, #2720, #14478, #8422, #37396, #3472, #3282, #59, #23572, #17891, #20364, #29050, #23013, #31721, #17328, #19991, #34749, #11446, #15041, #14854, #29436, #34563, #3094, #11626, #14662, #31907, #26589, #35117, #5937, #17701, #9166, #249, #5560, #619, #20548, #28681, #29241, #8977, #5749, #23201, #17516, #12188, #25848, #17145, #11813, #23383, #34932, #26403, #23760, #32091, #14295, #8603, #20173, #6123, #26031, #28871, #436, #2906, #20733, #12001, #8792, #32276, #29812, #35493, #4221, #18268, #18654, #24328, #32656, #15607, #26969, #6697, #35870, #1186, #35683, #9735, #21496, #24511, #3846, #24141, #18840, #12950, #27349, #12760, #33226, #30005, #21307, #9543, #9912, #18464, #15423, #35299, #30386, #12381, #23951, #15990, #32843, #998, #10103, #21117, #6508, #20926, #12574, #7265, #27163, #6888, #27538, #4035, #33037, #7086, #30195, #15799, #1563, #36059, #4407, #1379, #21672, #13135, #9355, #32465, #18083, #29624, #15230, #3659, #26780, #810, #13700, #31132, #5338, #10844, #33412, #16174, #19024, #22418, #4783, #27724, #33786, #22605, #25435, #7824, #34150, #30581, #19215, #24878, #5149, #7638, #8007, #25251, #22048, #4963, #16357, #33599, #36801, #28091, #25062, #36615, #33965, #13886, #30761, #13504, #8197, #2312, #16730, #2123, #19773, #19401, #10656, #36427, #19580, #30945, #27905, #24690, #31310, #1754, #13320, #16916, #22235, #1936, #36987, #10470, #7450, #10285, #16545, #28457, #28276, #11030, #2493, #36243, #21859, #4597, #20320, #8562, #32235, #3239, #23528, #17662, #392, #14253, #14622, #17101, #34892, #11585, #29390, #6274, #25989, #19, #37174, #31861, #11958, #8381, #20129, #14068, #5516, #9123, #8932, #5705, #29197, #35074, #23160, #34702, #28640, #37351, #22974, #25617, #2861, #2678, #20690, #20509, #17851, #25802, #8749, #17285, #5895, #17473, #11215, #14811, #29008, #23341, #26356, #3052, #22787, #34336, #26173, #19952, #32046, #209, #11775 ),
 ( #6077, #31493, #11403, #34522, #31676, #28826, #14435, #35828, #21262, #9312, #9868, #12141, #21075, #36016, #1335, #18037, #7226, #18415, #10055, #29767, #18799, #15753, #23908, #21631, #3426, #33182, #23717, #32613, #14994, #21449, #12713, #30153, #9498, #26545, #27120, #29581, #18227, #4181, #15185, #574, #24469, #35257, #20883, #27304, #35639, #26732, #12905, #32989, #32422, #6467, #7042, #29961, #3798, #955, #15376, #3619, #766, #26925, #12334, #35450, #6651, #9685, #32801, #24283, #12530, #24093, #6837, #3989, #15563, #1143, #18609, #10431, #8159, #1894, #4365, #36762, #36573, #19359, #10615, #33741, #27497, #10988, #19171, #10804, #34107, #19541, #2085, #36197, #30719, #30340, #25017, #7781, #15944, #1518, #31088, #13092, #5112, #24647, #7595, #16130, #10241, #30535, #16691, #25211, #13465, #21817, #30900, #33369, #4921, #7406, #13278, #18978, #2268, #16502, #28050, #4555, #22560, #24832, #28239, #13845, #36384, #27680, #13658, #1706, #4739, #25393, #22004, #33556, #36943, #16315, #27862, #22194, #22377, #33925, #7967, #673, #17388, #32517, #12244, #9219, #9033, #17757, #32144, #28928, #29677, #20604, #11684, #15282, #26836, #26455, #12055, #29490, #14721, #3151, #14905, #31962, #26268, #303, #6184, #11868, #35551, #29298, #31271, #26643, #489, #20790, #23627, #35171, #2965, #865, #3336, #23815, #24005, #9408, #3528, #26089, #32334, #19733, #6372, #17945, #5806, #14533, #20984, #119, #6561, #23258, #34989, #5994, #34802, #20419, #18136, #15094, #35357, #8847, #3712, #17574, #12436, #29107, #23437, #1051, #19077, #10153, #21728, #13372, #27775, #30057, #10340, #27397, #35923, #24378, #29867, #9965, #18890, #33091, #27589, #9781, #7136, #15473, #24189, #33278, #32897, #18708, #7317, #4462, #1428, #27027, #16040, #18323, #27214, #4645, #7502, #35734, #24927, #24561, #16225, #21545, #9596, #21910, #4091, #1805, #21169, #32708, #3901, #1237, #6749, #1618, #30441, #12625, #33460, #21357, #30248, #6949, #18518, #15663, #36292, #13188, #4275, #12808, #36111, #15849, #24743, #13005, #30629, #27958, #8431, #37037, #11084, #2730, #17154 ) ),
 .UNSPECIFIED., .F., .F., .F. ) 
 B_SPLINE_SURFACE_WITH_KNOTS ( ( 2, 2 ),
 ( 3, 2, 2, 2, 2, 2, 2, 2, 2, 2, 2, 2, 2, 2, 2, 2, 2, 2, 2, 2, 2, 2, 2, 2, 2, 2, 2, 2, 2, 2, 2, 2, 2, 2, 2, 2, 2, 2, 2, 2, 2, 2, 2, 2, 2, 2, 2, 2, 2, 2, 2, 2, 2, 2, 2, 2, 2, 2, 2, 2, 2, 2, 2, 2, 2, 2, 2, 2, 2, 2, 2, 2, 2, 2, 2, 2, 2, 2, 2, 2, 2, 2, 2, 2, 2, 2, 2, 2, 2, 2, 2, 2, 2, 2, 2, 2, 2, 2, 2, 2, 2, 2, 2, 2, 2, 2, 2, 2, 2, 2, 2, 2, 2, 2, 2, 2, 2, 2, 2, 2, 2, 2, 2, 2, 2, 2, 2, 2, 2, 2, 2, 2, 2, 2, 3 ),
 ( 0.000000000000000000, 1.000000000000000000 ),
 ( 0.000000000000000000, 0.007246376811594202987, 0.01449275362318840597, 0.02173913043478260809, 0.02898550724637681195, 0.03623188405797101580, 0.04347826086956521618, 0.05072463768115942351, 0.05797101449275362389, 0.06521739130434782428, 0.07246376811594203160, 0.07971014492753622505, 0.08695652173913043237, 0.09420289855072463969, 0.1014492753623188470, 0.1086956521739130405, 0.1159420289855072478, 0.1231884057971014551, 0.1304347826086956486, 0.1376811594202898559, 0.1449275362318840632, 0.1521739130434782705, 0.1594202898550724501, 0.1666666666666666574, 0.1739130434782608647, 0.1811594202898550721, 0.1884057971014492794, 0.1956521739130434867, 0.2028985507246376940, 0.2101449275362318736, 0.2173913043478260809, 0.2246376811594202882, 0.2318840579710144956, 0.2391304347826087029, 0.2463768115942029102, 0.2536231884057971175, 0.2608695652173912971, 0.2681159420289855322, 0.2753623188405797118, 0.2826086956521738913, 0.2898550724637681264, 0.2971014492753623060, 0.3043478260869565410, 0.3115942028985507206, 0.3188405797101449002, 0.3260869565217391353, 0.3333333333333333148, 0.3405797101449275499, 0.3478260869565217295, 0.3550724637681159646, 0.3623188405797101441, 0.3695652173913043237, 0.3768115942028985588, 0.3840579710144927383, 0.3913043478260869734, 0.3985507246376811530, 0.4057971014492753881, 0.4130434782608695676, 0.4202898550724637472, 0.4275362318840579823, 0.4347826086956521618, 0.4420289855072463969, 0.4492753623188405765, 0.4565217391304347561, 0.4637681159420289911, 0.4710144927536231707, 0.4782608695652174058, 0.4855072463768115854, 0.4927536231884058204, 0.5000000000000000000, 0.5072463768115942351, 0.5144927536231883591, 0.5217391304347825942, 0.5289855072463768293, 0.5362318840579710644, 0.5434782608695651884, 0.5507246376811594235, 0.5579710144927536586, 0.5652173913043477826, 0.5724637681159420177, 0.5797101449275362528, 0.5869565217391304879, 0.5942028985507246119, 0.6014492753623188470, 0.6086956521739130821, 0.6159420289855072062, 0.6231884057971014412, 0.6304347826086956763, 0.6376811594202898004, 0.6449275362318840354, 0.6521739130434782705, 0.6594202898550725056, 0.6666666666666666297, 0.6739130434782608647, 0.6811594202898550998, 0.6884057971014492239, 0.6956521739130434590, 0.7028985507246376940, 0.7101449275362319291, 0.7173913043478260532, 0.7246376811594202882, 0.7318840579710145233, 0.7391304347826086474, 0.7463768115942028825, 0.7536231884057971175, 0.7608695652173913526, 0.7681159420289854767, 0.7753623188405797118, 0.7826086956521739468, 0.7898550724637680709, 0.7971014492753623060, 0.8043478260869565410, 0.8115942028985507761, 0.8188405797101449002, 0.8260869565217391353, 0.8333333333333333703, 0.8405797101449274944, 0.8478260869565217295, 0.8550724637681159646, 0.8623188405797101996, 0.8695652173913043237, 0.8768115942028985588, 0.8840579710144927938, 0.8913043478260869179, 0.8985507246376811530, 0.9057971014492753881, 0.9130434782608695121, 0.9202898550724637472, 0.9275362318840579823, 0.9347826086956522174, 0.9420289855072463414, 0.9492753623188405765, 0.9565217391304348116, 0.9637681159420289356, 0.9662082973083875315 ),
 .UNSPECIFIED. ) 
 GEOMETRIC_REPRESENTATION_ITEM ( )  RATIONAL_B_SPLINE_SURFACE ( (
 ( 1.000000000000000000, 0.8660254037844387076, 1.000000000000000000, 0.8660254037844387076, 1.000000000000000000, 0.8660254037844387076, 1.000000000000000000, 0.8660254037844387076, 1.000000000000000000, 0.8660254037844387076, 1.000000000000000000, 0.8660254037844387076, 1.000000000000000000, 0.8660254037844387076, 1.000000000000000000, 0.8660254037844387076, 1.000000000000000000, 0.8660254037844387076, 1.000000000000000000, 0.8660254037844387076, 1.000000000000000000, 0.8660254037844387076, 1.000000000000000000, 0.8660254037844387076, 1.000000000000000000, 0.8660254037844387076, 1.000000000000000000, 0.8660254037844387076, 1.000000000000000000, 0.8660254037844387076, 1.000000000000000000, 0.8660254037844387076, 1.000000000000000000, 0.8660254037844387076, 1.000000000000000000, 0.8660254037844387076, 1.000000000000000000, 0.8660254037844387076, 1.000000000000000000, 0.8660254037844387076, 1.000000000000000000, 0.8660254037844387076, 1.000000000000000000, 0.8660254037844387076, 1.000000000000000000, 0.8660254037844387076, 1.000000000000000000, 0.8660254037844387076, 1.000000000000000000, 0.8660254037844387076, 1.000000000000000000, 0.8660254037844387076, 1.000000000000000000, 0.8660254037844387076, 1.000000000000000000, 0.8660254037844387076, 1.000000000000000000, 0.8660254037844387076, 1.000000000000000000, 0.8660254037844387076, 1.000000000000000000, 0.8660254037844387076, 1.000000000000000000, 0.8660254037844387076, 1.000000000000000000, 0.8660254037844387076, 1.000000000000000000, 0.8660254037844387076, 1.000000000000000000, 0.8660254037844387076, 1.000000000000000000, 0.8660254037844387076, 1.000000000000000000, 0.8660254037844387076, 1.000000000000000000, 0.8660254037844387076, 1.000000000000000000, 0.8660254037844387076, 1.000000000000000000, 0.8660254037844387076, 1.000000000000000000, 0.8660254037844387076, 1.000000000000000000, 0.8660254037844387076, 1.000000000000000000, 0.8660254037844387076, 1.000000000000000000, 0.8660254037844387076, 1.000000000000000000, 0.8660254037844387076, 1.000000000000000000, 0.8660254037844387076, 1.000000000000000000, 0.8660254037844387076, 1.000000000000000000, 0.8660254037844387076, 1.000000000000000000, 0.8660254037844387076, 1.000000000000000000, 0.8660254037844387076, 1.000000000000000000, 0.8660254037844387076, 1.000000000000000000, 0.8660254037844387076, 1.000000000000000000, 0.8660254037844387076, 1.000000000000000000, 0.8660254037844387076, 1.000000000000000000, 0.8660254037844387076, 1.000000000000000000, 0.8660254037844387076, 1.000000000000000000, 0.8660254037844387076, 1.000000000000000000, 0.8660254037844387076, 1.000000000000000000, 0.8660254037844387076, 1.000000000000000000, 0.8660254037844387076, 1.000000000000000000, 0.8660254037844387076, 1.000000000000000000, 0.8660254037844387076, 1.000000000000000000, 0.8660254037844387076, 1.000000000000000000, 0.8660254037844387076, 1.000000000000000000, 0.8660254037844387076, 1.000000000000000000, 0.8660254037844387076, 1.000000000000000000, 0.8660254037844387076, 1.000000000000000000, 0.8660254037844387076, 1.000000000000000000, 0.8660254037844387076, 1.000000000000000000, 0.8660254037844387076, 1.000000000000000000, 0.8660254037844387076, 1.000000000000000000, 0.8660254037844387076, 1.000000000000000000, 0.8660254037844387076, 1.000000000000000000, 0.8660254037844387076, 1.000000000000000000, 0.8660254037844387076, 1.000000000000000000, 0.8660254037844387076, 1.000000000000000000, 0.8660254037844387076, 1.000000000000000000, 0.8660254037844387076, 1.000000000000000000, 0.8660254037844387076, 1.000000000000000000, 0.8660254037844387076, 1.000000000000000000, 0.8660254037844387076, 1.000000000000000000, 0.8660254037844387076, 1.000000000000000000, 0.8660254037844387076, 1.000000000000000000, 0.8660254037844387076, 1.000000000000000000, 0.8660254037844387076, 1.000000000000000000, 0.8660254037844387076, 1.000000000000000000, 0.8660254037844387076, 1.000000000000000000, 0.8660254037844387076, 1.000000000000000000, 0.8660254037844387076, 1.000000000000000000, 0.8660254037844387076, 1.000000000000000000, 0.8660254037844387076, 1.000000000000000000, 0.8660254037844387076, 1.000000000000000000, 0.8660254037844387076, 1.000000000000000000, 0.8660254037844387076, 1.000000000000000000, 0.8660254037844387076, 1.000000000000000000, 0.8660254037844387076, 1.000000000000000000, 0.8660254037844387076, 1.000000000000000000, 0.8660254037844387076, 1.000000000000000000, 0.8660254037844387076, 1.000000000000000000, 0.8660254037844387076, 1.000000000000000000, 0.8660254037844387076, 1.000000000000000000, 0.8660254037844387076, 1.000000000000000000, 0.8660254037844387076, 1.000000000000000000, 0.8660254037844387076, 1.000000000000000000, 0.8660254037844387076, 1.000000000000000000, 0.8660254037844387076, 1.000000000000000000, 0.8660254037844387076, 1.000000000000000000, 0.8660254037844387076, 1.000000000000000000, 0.8660254037844387076, 1.000000000000000000, 0.8660254037844387076, 1.000000000000000000, 0.8660254037844387076, 1.000000000000000000, 0.8660254037844387076, 1.000000000000000000, 0.8660254037844387076, 1.000000000000000000, 0.8660254037844387076, 1.000000000000000000, 0.8660254037844387076, 1.000000000000000000, 0.8660254037844387076, 1.000000000000000000, 0.8660254037844387076, 1.000000000000000000, 0.8660254037844387076, 1.000000000000000000, 0.8660254037844387076, 1.000000000000000000, 0.8660254037844387076, 1.000000000000000000, 0.8660254037844387076, 1.000000000000000000, 0.8660254037844387076, 1.000000000000000000, 0.8660254037844387076, 1.000000000000000000, 0.8660254037844387076, 1.000000000000000000, 0.8660254037844387076, 1.000000000000000000, 0.8660254037844387076, 1.000000000000000000, 0.8660254037844387076, 1.000000000000000000, 0.8660254037844387076, 1.000000000000000000, 0.8660254037844387076, 1.000000000000000000, 0.8660254037844387076, 1.000000000000000000, 0.8660254037844387076, 1.000000000000000000, 0.8660254037844387076, 1.000000000000000000, 0.8660254037844387076, 1.000000000000000000, 0.9548847207714133978, 0.9401541335272454170),
 ( 1.000000000000000000, 0.8660254037844387076, 1.000000000000000000, 0.8660254037844387076, 1.000000000000000000, 0.8660254037844387076, 1.000000000000000000, 0.8660254037844387076, 1.000000000000000000, 0.8660254037844387076, 1.000000000000000000, 0.8660254037844387076, 1.000000000000000000, 0.8660254037844387076, 1.000000000000000000, 0.8660254037844387076, 1.000000000000000000, 0.8660254037844387076, 1.000000000000000000, 0.8660254037844387076, 1.000000000000000000, 0.8660254037844387076, 1.000000000000000000, 0.8660254037844387076, 1.000000000000000000, 0.8660254037844387076, 1.000000000000000000, 0.8660254037844387076, 1.000000000000000000, 0.8660254037844387076, 1.000000000000000000, 0.8660254037844387076, 1.000000000000000000, 0.8660254037844387076, 1.000000000000000000, 0.8660254037844387076, 1.000000000000000000, 0.8660254037844387076, 1.000000000000000000, 0.8660254037844387076, 1.000000000000000000, 0.8660254037844387076, 1.000000000000000000, 0.8660254037844387076, 1.000000000000000000, 0.8660254037844387076, 1.000000000000000000, 0.8660254037844387076, 1.000000000000000000, 0.8660254037844387076, 1.000000000000000000, 0.8660254037844387076, 1.000000000000000000, 0.8660254037844387076, 1.000000000000000000, 0.8660254037844387076, 1.000000000000000000, 0.8660254037844387076, 1.000000000000000000, 0.8660254037844387076, 1.000000000000000000, 0.8660254037844387076, 1.000000000000000000, 0.8660254037844387076, 1.000000000000000000, 0.8660254037844387076, 1.000000000000000000, 0.8660254037844387076, 1.000000000000000000, 0.8660254037844387076, 1.000000000000000000, 0.8660254037844387076, 1.000000000000000000, 0.8660254037844387076, 1.000000000000000000, 0.8660254037844387076, 1.000000000000000000, 0.8660254037844387076, 1.000000000000000000, 0.8660254037844387076, 1.000000000000000000, 0.8660254037844387076, 1.000000000000000000, 0.8660254037844387076, 1.000000000000000000, 0.8660254037844387076, 1.000000000000000000, 0.8660254037844387076, 1.000000000000000000, 0.8660254037844387076, 1.000000000000000000, 0.8660254037844387076, 1.000000000000000000, 0.8660254037844387076, 1.000000000000000000, 0.8660254037844387076, 1.000000000000000000, 0.8660254037844387076, 1.000000000000000000, 0.8660254037844387076, 1.000000000000000000, 0.8660254037844387076, 1.000000000000000000, 0.8660254037844387076, 1.000000000000000000, 0.8660254037844387076, 1.000000000000000000, 0.8660254037844387076, 1.000000000000000000, 0.8660254037844387076, 1.000000000000000000, 0.8660254037844387076, 1.000000000000000000, 0.8660254037844387076, 1.000000000000000000, 0.8660254037844387076, 1.000000000000000000, 0.8660254037844387076, 1.000000000000000000, 0.8660254037844387076, 1.000000000000000000, 0.8660254037844387076, 1.000000000000000000, 0.8660254037844387076, 1.000000000000000000, 0.8660254037844387076, 1.000000000000000000, 0.8660254037844387076, 1.000000000000000000, 0.8660254037844387076, 1.000000000000000000, 0.8660254037844387076, 1.000000000000000000, 0.8660254037844387076, 1.000000000000000000, 0.8660254037844387076, 1.000000000000000000, 0.8660254037844387076, 1.000000000000000000, 0.8660254037844387076, 1.000000000000000000, 0.8660254037844387076, 1.000000000000000000, 0.8660254037844387076, 1.000000000000000000, 0.8660254037844387076, 1.000000000000000000, 0.8660254037844387076, 1.000000000000000000, 0.8660254037844387076, 1.000000000000000000, 0.8660254037844387076, 1.000000000000000000, 0.8660254037844387076, 1.000000000000000000, 0.8660254037844387076, 1.000000000000000000, 0.8660254037844387076, 1.000000000000000000, 0.8660254037844387076, 1.000000000000000000, 0.8660254037844387076, 1.000000000000000000, 0.8660254037844387076, 1.000000000000000000, 0.8660254037844387076, 1.000000000000000000, 0.8660254037844387076, 1.000000000000000000, 0.8660254037844387076, 1.000000000000000000, 0.8660254037844387076, 1.000000000000000000, 0.8660254037844387076, 1.000000000000000000, 0.8660254037844387076, 1.000000000000000000, 0.8660254037844387076, 1.000000000000000000, 0.8660254037844387076, 1.000000000000000000, 0.8660254037844387076, 1.000000000000000000, 0.8660254037844387076, 1.000000000000000000, 0.8660254037844387076, 1.000000000000000000, 0.8660254037844387076, 1.000000000000000000, 0.8660254037844387076, 1.000000000000000000, 0.8660254037844387076, 1.000000000000000000, 0.8660254037844387076, 1.000000000000000000, 0.8660254037844387076, 1.000000000000000000, 0.8660254037844387076, 1.000000000000000000, 0.8660254037844387076, 1.000000000000000000, 0.8660254037844387076, 1.000000000000000000, 0.8660254037844387076, 1.000000000000000000, 0.8660254037844387076, 1.000000000000000000, 0.8660254037844387076, 1.000000000000000000, 0.8660254037844387076, 1.000000000000000000, 0.8660254037844387076, 1.000000000000000000, 0.8660254037844387076, 1.000000000000000000, 0.8660254037844387076, 1.000000000000000000, 0.8660254037844387076, 1.000000000000000000, 0.8660254037844387076, 1.000000000000000000, 0.8660254037844387076, 1.000000000000000000, 0.8660254037844387076, 1.000000000000000000, 0.8660254037844387076, 1.000000000000000000, 0.8660254037844387076, 1.000000000000000000, 0.8660254037844387076, 1.000000000000000000, 0.8660254037844387076, 1.000000000000000000, 0.8660254037844387076, 1.000000000000000000, 0.8660254037844387076, 1.000000000000000000, 0.8660254037844387076, 1.000000000000000000, 0.8660254037844387076, 1.000000000000000000, 0.8660254037844387076, 1.000000000000000000, 0.8660254037844387076, 1.000000000000000000, 0.8660254037844387076, 1.000000000000000000, 0.8660254037844387076, 1.000000000000000000, 0.8660254037844387076, 1.000000000000000000, 0.8660254037844387076, 1.000000000000000000, 0.8660254037844387076, 1.000000000000000000, 0.8660254037844387076, 1.000000000000000000, 0.8660254037844387076, 1.000000000000000000, 0.8660254037844387076, 1.000000000000000000, 0.8660254037844387076, 1.000000000000000000, 0.8660254037844387076, 1.000000000000000000, 0.8660254037844387076, 1.000000000000000000, 0.9548847207714133978, 0.9401541335272454170) ) ) 
 REPRESENTATION_ITEM ( '' )  SURFACE ( )  );
#34961=CARTESIAN_POINT ( 'NONE',  ( 30.58849351077567036, -7.209453229046482114, 159.5969823328619555 ) ) ;
#34975=CARTESIAN_POINT ( 'NONE',  ( 21.00000000000000000, 6.928203230275506996, -7.762500000000014388 ) ) ;
#34977=CARTESIAN_POINT ( 'NONE',  ( 25.21024869186586059, -3.464101615137884060, 166.9656422296849030 ) ) ;
#34980=CARTESIAN_POINT ( 'NONE',  ( 28.02930337212723089, -5.407089921784859143, 166.1637690562780278 ) ) ;
#34984=ORIENTED_EDGE ( 'NONE', *, *, #26533, .F. ) ;
#34987=CARTESIAN_POINT ( 'NONE',  ( 28.51246655749191561, 5.725135026351853007, 159.7765254096146919 ) ) ;
#34989=CARTESIAN_POINT ( 'NONE',  ( 26.75643035624999655, 7.049594010296217766E-16, -7.115624999385477878 ) ) ;
#34992=CARTESIAN_POINT ( 'NONE',  ( 26.99999999999999645, 7.347880794884117764E-16, -5.118749998770960374 ) ) ;
#34997=CARTESIAN_POINT ( 'NONE',  ( 24.43404934156608022, 3.604726614523240613, 160.8882913061285080 ) ) ;
#35006=( BOUNDED_CURVE ( )  B_SPLINE_CURVE ( 2, ( #36831, #10314, #13349, #4624, #21704, #12981, #7852 ),
 .UNSPECIFIED., .F., .F. ) 
 B_SPLINE_CURVE_WITH_KNOTS ( ( 3, 2, 2, 3 ),
 ( 0.3695652173913033800, 0.3768115942028977816, 0.3840579710144920722, 0.3913043478260864738 ),
 .UNSPECIFIED. ) 
 CURVE ( )  GEOMETRIC_REPRESENTATION_ITEM ( )  RATIONAL_B_SPLINE_CURVE ( ( 1.000000000000017319, 0.8660254037844211661, 1.000000000000000000, 0.8660254037844387076, 1.000000000000000000, 0.8660254037844479225, 0.9999999999999907851 ) ) 
 REPRESENTATION_ITEM ( '' )  );
#35009=CARTESIAN_POINT ( 'NONE',  ( 26.99999999999999645, 7.347880794884117764E-16, -6.074999999999997513 ) ) ;
#35010=CARTESIAN_POINT ( 'NONE',  ( 26.52314049301468657, 1.665113505852782616, -8.000000000000000000 ) ) ;
#35011=CARTESIAN_POINT ( 'NONE',  ( 27.50636891564131759, 5.407089921784856479, 160.1866008677275772 ) ) ;
#35012=CARTESIAN_POINT ( 'NONE',  ( 15.00000000000000000, 0.000000000000000000, -1.743749998770943721 ) ) ;
#35019=CARTESIAN_POINT ( 'NONE',  ( 25.01741661114323634, 3.464101615137552770, 164.7615614613813193 ) ) ;
#35020=DIRECTION ( 'NONE',  ( 0.000000000000000000, 0.000000000000000000, 1.000000000000000000 ) ) ;
#35021=ORIENTED_EDGE ( 'NONE', *, *, #14244, .T. ) ;
#35023=CARTESIAN_POINT ( 'NONE',  ( 21.00000000000000000, -6.646953231504538984, -8.578124999385442706 ) ) ;
#35025=CARTESIAN_POINT ( 'NONE',  ( 31.05913452161298949, -7.209453229046482114, 164.9764337025573866 ) ) ;
#35026=CARTESIAN_POINT ( 'NONE',  ( 25.09258843915631587, -3.464101615137761048, 165.6207793872610523 ) ) ;
#35037=CARTESIAN_POINT ( 'NONE',  ( 23.87821517812500005, -4.985214923628404016, -3.703124999385493332 ) ) ;
#35049=CARTESIAN_POINT ( 'NONE',  ( 25.00761158997698175, 3.464101615137542112, 164.6494895566216314 ) ) ;
#35052=CARTESIAN_POINT ( 'NONE',  ( 21.00000000000000355, 0.000000000000000000, 50.00000000000001421 ) ) ;
#35055=CARTESIAN_POINT ( 'NONE',  ( 35.44346792208517627, 0.000000000000000000, 169.1947408000190194 ) ) ;
#35060=CARTESIAN_POINT ( 'NONE',  ( 31.43662783238875136, 7.209453229046475009, 169.2912019886672681 ) ) ;
#35062=CARTESIAN_POINT ( 'NONE',  ( 21.00000000000000000, 6.646953231504538984, -0.2531249993854407521 ) ) ;
#35064=CARTESIAN_POINT ( 'NONE',  ( 18.00000000000000355, -5.196152422706632912, -4.818749998770965881 ) ) ;
#35067=ADVANCED_FACE ( 'NONE', ( #20457 ), #11720, .T. ) ;
#35068=CARTESIAN_POINT ( 'NONE',  ( 15.00000000000000000, 0.000000000000000000, -0.4500000000000059508 ) ) ;
#35070=CARTESIAN_POINT ( 'NONE',  ( 15.00000000000000355, 7.347880794884112834E-16, -8.000000000000000000 ) ) ;
#35074=CARTESIAN_POINT ( 'NONE',  ( 15.24356964375000167, -3.323476615752272600, -9.215624999385486404 ) ) ;
#35077=VERTEX_POINT ( 'NONE', #37305 ) ;
#35079=VERTEX_POINT ( 'NONE', #17049 ) ;
#35081=CARTESIAN_POINT ( 'NONE',  ( 34.26382187998621731, 5.407089921784862696, 165.7877139618832985 ) ) ;
#35089=CARTESIAN_POINT ( 'NONE',  ( 28.29077060037018043, 5.407089921784856479, 169.1523531505532674 ) ) ;
#35106=CARTESIAN_POINT ( 'NONE',  ( 25.25273711656209841, 3.464101615137667789, 167.4512871462289638 ) ) ;
#35107=CARTESIAN_POINT ( 'NONE',  ( 34.40478479951106294, 5.196152422706631135, 168.7962516286712571 ) ) ;
#35116=CARTESIAN_POINT ( 'NONE',  ( 24.44222019244867283, 0.000000000000000000, 160.9816845590745800 ) ) ;
#35117=CARTESIAN_POINT ( 'NONE',  ( 15.24356964374999990, 3.323476615752268604, -2.090624999385484628 ) ) ;
#35122=CARTESIAN_POINT ( 'NONE',  ( 18.12178482187500350, -4.985214923628407568, -5.465624999385465088 ) ) ;
#35128=CARTESIAN_POINT ( 'NONE',  ( 30.71350752933288675, 6.928203230275506996, 161.0258991035495058 ) ) ;
#35132=CARTESIAN_POINT ( 'NONE',  ( 15.24356964375000167, -3.323476615752272600, -5.615624999385488536 ) ) ;
#35136=ORIENTED_EDGE ( 'NONE', *, *, #1006, .F. ) ;
#35142=CARTESIAN_POINT ( 'NONE',  ( 33.71474070067601048, 5.407089921784862696, 159.5116873639053097 ) ) ;
#35143=VECTOR ( 'NONE', #1158, 1000.000000000000000 ) ;
#35147=CARTESIAN_POINT ( 'NONE',  ( 27.00000000000031619, -3.464101615137567869, -2.006249998770949006 ) ) ;
#35155=CARTESIAN_POINT ( 'NONE',  ( 23.99999999999999645, 5.196152422706631135, -8.250000000000007105 ) ) ;
#35157=EDGE_CURVE ( 'NONE', #6148, #7924, #20081, .T. ) ;
#35158=CARTESIAN_POINT ( 'NONE',  ( 23.99999999999999645, 5.196152422706631135, -6.843749998770965348 ) ) ;
#35160=CARTESIAN_POINT ( 'NONE',  ( 37.45053336641773711, 7.646167579472015790E-16, 166.3935290647278009 ) ) ;
#35166=EDGE_LOOP ( 'NONE', ( #10516, #3604, #6289, #35644 ) ) ;
#35168=CARTESIAN_POINT ( 'NONE',  ( 21.00000000000016342, -4.000000000000002665, 50.00000000000000000 ) ) ;
#35169=DIRECTION ( 'NONE',  ( 0.9961946980917462113, 0.000000000000000000, -0.08715574274765118534 ) ) ;
#35171=CARTESIAN_POINT ( 'NONE',  ( 15.24356964375000167, -3.323476615752272600, -6.403124999385489069 ) ) ;
#35176=AXIS2_PLACEMENT_3D ( 'NONE', #35052, #14413, #17264 ) ;
#35179=CARTESIAN_POINT ( 'NONE',  ( 24.44058602227215005, -3.604726614523244610, 160.9630059084853997 ) ) ;
#35192=CARTESIAN_POINT ( 'NONE',  ( 25.00000000000001421, -2.343145750507543035, 49.82535622836641664 ) ) ;
#35193=CARTESIAN_POINT ( 'NONE',  ( 34.32918868704696536, -5.407089921784861808, 166.5348599854521296 ) ) ;
#35194=CARTESIAN_POINT ( 'NONE',  ( 18.00000000000000355, -5.196152422706632912, -1.668749998770951981 ) ) ;
#35203=CARTESIAN_POINT ( 'NONE',  ( 27.46714883140487373, 5.407089921784856479, 159.7383132535862842 ) ) ;
#35204=VECTOR ( 'NONE', #35528, 1000.000000000000000 ) ;
#35205=CARTESIAN_POINT ( 'NONE',  ( 18.12178482187500350, -4.985214923628407568, -9.065624999385457627 ) ) ;
#35206=CARTESIAN_POINT ( 'NONE',  ( 25.41288579386105440, 0.000000000000000000, 169.2817949039725818 ) ) ;
#35207=CARTESIAN_POINT ( 'NONE',  ( 27.89366724747619131, 5.407089921784862696, 164.6134410573727678 ) ) ;
#35208=CARTESIAN_POINT ( 'NONE',  ( 33.95048549033182184, -5.196152422706635576, 163.6035867636436478 ) ) ;
#35216=VERTEX_POINT ( 'NONE', #31625 ) ;
#35220=CARTESIAN_POINT ( 'NONE',  ( 21.00000000000000000, -6.646953231504538984, -3.290624999385483918 ) ) ;
#35223=( BOUNDED_CURVE ( )  B_SPLINE_CURVE ( 2, ( #7904, #13593, #13030, #34045, #10737, #1647, #16628 ),
 .UNSPECIFIED., .F., .F. ) 
 B_SPLINE_CURVE_WITH_KNOTS ( ( 3, 2, 2, 3 ),
 ( 0.3260869565217381361, 0.3333333333333324267, 0.3405797101449267172, 0.3478260869565210078 ),
 .UNSPECIFIED. ) 
 CURVE ( )  GEOMETRIC_REPRESENTATION_ITEM ( )  RATIONAL_B_SPLINE_CURVE ( ( 1.000000000000018430, 0.8660254037844202779, 1.000000000000000000, 0.8660254037844387076, 1.000000000000000000, 0.8660254037844520303, 0.9999999999999866773 ) ) 
 REPRESENTATION_ITEM ( '' )  );
#35234=DIRECTION ( 'NONE',  ( 0.08715574274765143514, 0.000000000000000000, 0.9961946980917462113 ) ) ;
#35235=CARTESIAN_POINT ( 'NONE',  ( 37.29365302947196881, 7.646167579472015790E-16, 164.6003786081626572 ) ) ;
#35245=ORIENTED_EDGE ( 'NONE', *, *, #25170, .F. ) ;
#35246=CARTESIAN_POINT ( 'NONE',  ( 28.17311034766084887, 5.407089921784856479, 167.8074903081294167 ) ) ;
#35247=CARTESIAN_POINT ( 'NONE',  ( 21.00000000000000000, -6.646953231504538984, -4.078124999385484450 ) ) ;
#35249=CARTESIAN_POINT ( 'NONE',  ( 15.00000000000000000, 0.000000000000000000, -4.893749998770957177 ) ) ;
#35257=CARTESIAN_POINT ( 'NONE',  ( 26.75643035624999655, 3.323476615752271712, -1.678124999385453897 ) ) ;
#35259=CARTESIAN_POINT ( 'NONE',  ( 18.00000000000000355, -5.196152422706632912, -6.618749998770962151 ) ) ;
#35261=ORIENTED_EDGE ( 'NONE', *, *, #5154, .F. ) ;
#35264=CARTESIAN_POINT ( 'NONE',  ( 37.25279877505902704, 3.604726614523243278, 164.1334123434321270 ) ) ;
#35271=CARTESIAN_POINT ( 'NONE',  ( 24.87364111904954811, 0.000000000000000000, 165.9128483146287465 ) ) ;
#35289=EDGE_CURVE ( 'NONE', #18997, #24079, #31643, .T. ) ;
#35290=CARTESIAN_POINT ( 'NONE',  ( 36.63838227223424582, -3.464101615138058143, 159.9052478282085588 ) ) ;
#35293=LINE ( 'NONE', #11617, #37215 ) ;
#35298=CARTESIAN_POINT ( 'NONE',  ( 36.81974367828161121, -3.604726614523235284, 159.1835699372887802 ) ) ;
#35299=CARTESIAN_POINT ( 'NONE',  ( 26.75643035624999655, 3.323476615752271712, -4.490624999385484095 ) ) ;
#35303=VERTEX_POINT ( 'NONE', #712 ) ;
#35306=CARTESIAN_POINT ( 'NONE',  ( 26.75643035624999655, 3.323476615752271268, -4.828124999385488003 ) ) ;
#35313=CARTESIAN_POINT ( 'NONE',  ( 36.75931086529713099, 7.347880794884117764E-16, 161.2874679718108553 ) ) ;
#35316=AXIS2_PLACEMENT_3D ( 'NONE', #23467, #35020, #20635 ) ;
#35318=CARTESIAN_POINT ( 'NONE',  ( 26.75643035624999655, 7.049594010296217766E-16, -7.678124999385471661 ) ) ;
#35322=EDGE_CURVE ( 'NONE', #27062, #27666, #30446, .T. ) ;
#35327=CARTESIAN_POINT ( 'NONE',  ( 24.43404934156608022, 3.604726614523240613, 160.8882913061285080 ) ) ;
#35329=ADVANCED_FACE ( 'NONE', ( #16026 ), #26682, .T. ) ;
#35333=CARTESIAN_POINT ( 'NONE',  ( 25.39981243234174002, 3.464101615137729517, 169.1323656980344481 ) ) ;
#35338=ORIENTED_EDGE ( 'NONE', *, *, #664, .F. ) ;
#35339=CARTESIAN_POINT ( 'NONE',  ( 21.00000000000000000, -6.928203230275506996, -6.187500000000013323 ) ) ;
#35342=EDGE_CURVE ( 'NONE', #4247, #18435, #870, .T. ) ;
#35346=CARTESIAN_POINT ( 'NONE',  ( 28.18618370907300275, -5.407089921784859143, 167.9569195128432000 ) ) ;
#35351=ORIENTED_EDGE ( 'NONE', *, *, #5464, .T. ) ;
#35352=ORIENTED_EDGE ( 'NONE', *, *, #4037, .F. ) ;
#35357=CARTESIAN_POINT ( 'NONE',  ( 15.24356964374999990, 0.000000000000000000, -7.340624999385481075 ) ) ;
#35360=CYLINDRICAL_SURFACE ( 'NONE', #18196, 6.000000000000001776 ) ;
#35364=CARTESIAN_POINT ( 'NONE',  ( 37.35088046919680949, 3.464101615137755275, 168.0491394851085545 ) ) ;
#35374=ORIENTED_EDGE ( 'NONE', *, *, #9725, .F. ) ;
#35378=CARTESIAN_POINT ( 'NONE',  ( 34.30304196422265761, 5.407089921784862696, 166.2360015760246199 ) ) ;
#35385=CARTESIAN_POINT ( 'NONE',  ( 26.99999999999999645, 7.347880794884117764E-16, -5.175000000000013145 ) ) ;
#35388=DIRECTION ( 'NONE',  ( 0.000000000000000000, 0.000000000000000000, 1.000000000000000000 ) ) ;
#35389=CARTESIAN_POINT ( 'NONE',  ( 23.99999999999999645, 5.196152422706631135, -5.549999999999998934 ) ) ;
#35390=CARTESIAN_POINT ( 'NONE',  ( 33.75886329544200493, 5.407089921784857367, 160.0160109298142288 ) ) ;
#35391=CARTESIAN_POINT ( 'NONE',  ( 26.99999999999999645, -3.464101615137751278, -0.7125000000000065725 ) ) ;
#35392=CARTESIAN_POINT ( 'NONE',  ( 28.39493320743021698, 5.196152422706630247, 168.9456130733727548 ) ) ;
#35393=CARTESIAN_POINT ( 'NONE',  ( 24.94717877699287811, 0.000000000000000000, 166.7533875911436780 ) ) ;
#35395=CARTESIAN_POINT ( 'NONE',  ( 36.94560626531313829, 7.347880794884125653E-16, 163.4168341377576041 ) ) ;
#35406=CARTESIAN_POINT ( 'NONE',  ( 26.75643035624999655, 7.049594010296217766E-16, -4.978124999385491023 ) ) ;
#35408=( BOUNDED_CURVE ( )  B_SPLINE_CURVE ( 2, ( #6290, #32065, #27136, #1163, #6094, #24115, #23546 ),
 .UNSPECIFIED., .F., .F. ) 
 B_SPLINE_CURVE_WITH_KNOTS ( ( 3, 2, 2, 3 ),
 ( 0.1521739130434776321, 0.1594202898550719505, 0.1666666666666662966, 0.1739130434782606427 ),
 .UNSPECIFIED. ) 
 CURVE ( )  GEOMETRIC_REPRESENTATION_ITEM ( )  RATIONAL_B_SPLINE_CURVE ( ( 1.000000000000011768, 0.8660254037844269392, 1.000000000000000000, 0.8660254037844387076, 1.000000000000000000, 0.8660254037844428154, 0.9999999999999958922 ) ) 
 REPRESENTATION_ITEM ( '' )  );
#35416=CARTESIAN_POINT ( 'NONE',  ( 37.38683221308021842, 7.347880794884117764E-16, 168.4600697980714017 ) ) ;
#35422=CARTESIAN_POINT ( 'NONE',  ( 33.99418380086066804, 5.407089921784857367, 162.7057366146619586 ) ) ;
#35431=CARTESIAN_POINT ( 'NONE',  ( 26.99999999999999645, 7.347880794884117764E-16, -2.418749998770952647 ) ) ;
#35435=EDGE_LOOP ( 'NONE', ( #13315, #11629, #25419, #27907 ) ) ;
#35436=CARTESIAN_POINT ( 'NONE',  ( 31.20130732697009535, 7.209453229046475009, 166.6014763038195383 ) ) ;
#35438=CARTESIAN_POINT ( 'NONE',  ( 26.75643035624999655, 3.323476615752271712, -2.578124999385477345 ) ) ;
#35442=CARTESIAN_POINT ( 'NONE',  ( 14.99999999999941380, -3.464101615137419543, -7.556249998770961263 ) ) ;
#35446=ORIENTED_EDGE ( 'NONE', *, *, #21771, .F. ) ;
#35450=CARTESIAN_POINT ( 'NONE',  ( 15.24356964375000167, -3.323476615752272600, -2.353124999385463489 ) ) ;
#35452=CARTESIAN_POINT ( 'NONE',  ( 21.00000000000000000, -6.928203230275506996, -7.931249998770954157 ) ) ;
#35458=CARTESIAN_POINT ( 'NONE',  ( 34.18538171151332961, 5.407089921784862696, 164.8911387336007408 ) ) ;
#35465=CARTESIAN_POINT ( 'NONE',  ( 34.38638464322509947, 5.407089921784857367, 167.1886127560748321 ) ) ;
#35470=CIRCLE ( 'NONE', #16128, 4.000000000000000888 ) ;
#35476=ORIENTED_EDGE ( 'NONE', *, *, #34621, .F. ) ;
#35483=CARTESIAN_POINT ( 'NONE',  ( 21.00000000000016342, -4.000000000000002665, 50.00000000000000000 ) ) ;
#35485=FACE_OUTER_BOUND ( 'NONE', #5054, .T. ) ;
#35487=CARTESIAN_POINT ( 'NONE',  ( 26.97716818855048260, 0.000000000000000000, 49.47706554351410801 ) ) ;
#35492=CARTESIAN_POINT ( 'NONE',  ( 33.71964321120555752, 5.407089921784857367, 159.5677233156729642 ) ) ;
#35493=CARTESIAN_POINT ( 'NONE',  ( 15.24356964374999990, 3.323476615752268604, -3.440624999385503813 ) ) ;
#35500=CARTESIAN_POINT ( 'NONE',  ( 18.12178482187499640, 4.985214923628404904, -5.615624999385476990 ) ) ;
#35508=CARTESIAN_POINT ( 'NONE',  ( 36.64165061258780298, 7.347880794884117764E-16, 159.9426051293869477 ) ) ;
#35513=CARTESIAN_POINT ( 'NONE',  ( 23.87821517812500005, -4.985214923628404016, -6.853124999385479477 ) ) ;
#35523=CARTESIAN_POINT ( 'NONE',  ( 36.89981801693102170, 3.604726614523243278, 160.0988238161606034 ) ) ;
#35528=DIRECTION ( 'NONE',  ( 0.000000000000000000, 0.000000000000000000, 1.000000000000000000 ) ) ;
#35535=VERTEX_POINT ( 'NONE', #6600 ) ;
#35536=CARTESIAN_POINT ( 'NONE',  ( 15.00000000000000000, 3.464101615137752166, -6.337500000000001243 ) ) ;
#35538=CARTESIAN_POINT ( 'NONE',  ( 15.00000000000000000, 3.464101615137752610, -6.731249998770955756 ) ) ;
#35540=CARTESIAN_POINT ( 'NONE',  ( 25.06974154023176382, 0.000000000000000000, 168.1542863853351548 ) ) ;
#35546=ORIENTED_EDGE ( 'NONE', *, *, #16773, .T. ) ;
#35551=CARTESIAN_POINT ( 'NONE',  ( 23.87821517812499650, 4.985214923628404904, -6.140624999385474680 ) ) ;
#35555=CARTESIAN_POINT ( 'NONE',  ( 36.79853094953357129, 7.347880794884117764E-16, 161.7357555859521199 ) ) ;
#35558=CARTESIAN_POINT ( 'NONE',  ( 15.00000000000000000, 0.000000000000000000, -3.599999999999992095 ) ) ;
#35559=CARTESIAN_POINT ( 'NONE',  ( 28.13346597918727099, -5.196152422706632912, 165.9570289790974869 ) ) ;
#35567=EDGE_CURVE ( 'NONE', #10985, #30542, #21896, .T. ) ;
#35571=DIRECTION ( 'NONE',  ( 0.08715574274765150453, 0.000000000000000000, 0.9961946980917461003 ) ) ;
#35572=CARTESIAN_POINT ( 'NONE',  ( 28.10284103007056089, -5.407089921784865361, 167.0043083327929878 ) ) ;
#35583=CARTESIAN_POINT ( 'NONE',  ( 36.90145218710753738, 7.646167579472015790E-16, 160.1175024667497837 ) ) ;
#35584=CARTESIAN_POINT ( 'NONE',  ( 23.99999999999999645, 5.196152422706631135, -0.1500000000000112355 ) ) ;
#35587=CARTESIAN_POINT ( 'NONE',  ( 31.15718473220409379, 7.209453229046482114, 166.0971527379105908 ) ) ;
#35588=CARTESIAN_POINT ( 'NONE',  ( 36.98155800919654723, -3.464101615137755275, 163.8277644507203945 ) ) ;
#35599=CARTESIAN_POINT ( 'NONE',  ( 15.24356964375000167, -3.323476615752272600, -7.415624999385471483 ) ) ;
#35610=( BOUNDED_CURVE ( )  B_SPLINE_CURVE ( 2, ( #25182, #22348, #36735, #33710, #10774, #13437, #8315 ),
 .UNSPECIFIED., .F., .F. ) 
 B_SPLINE_CURVE_WITH_KNOTS ( ( 3, 2, 2, 3 ),
 ( 0.4347826086956516067, 0.4420289855072456753, 0.4492753623188397438, 0.4565217391304337569 ),
 .UNSPECIFIED. ) 
 CURVE ( )  GEOMETRIC_REPRESENTATION_ITEM ( )  RATIONAL_B_SPLINE_CURVE ( ( 1.000000000000010214, 0.8660254037844284936, 1.000000000000000000, 0.8660254037844387076, 1.000000000000000000, 0.8660254037844571373, 0.9999999999999815703 ) ) 
 REPRESENTATION_ITEM ( '' )  );
#35614=CARTESIAN_POINT ( 'NONE',  ( 24.79193261022362549, 3.604726614523236616, 164.9789157851677146 ) ) ;
#35618=CARTESIAN_POINT ( 'NONE',  ( 21.00000000000000355, 0.000000000000000000, 50.00000000000001421 ) ) ;
#35620=CARTESIAN_POINT ( 'NONE',  ( 24.00000000000000000, -5.196152422706629359, -4.293749998770940657 ) ) ;
#35625=CARTESIAN_POINT ( 'NONE',  ( 37.44726502606470575, -3.604726614523235284, 166.3561717635493551 ) ) ;
#35626=CARTESIAN_POINT ( 'NONE',  ( 15.24356964374999990, 0.000000000000000000, -2.390624999385471128 ) ) ;
#35639=CARTESIAN_POINT ( 'NONE',  ( 23.87821517812500005, -4.985214923628404016, -1.790624999385481697 ) ) ;
#35642=CARTESIAN_POINT ( 'NONE',  ( 26.99999999999999645, -3.464101615137751278, -8.306249998770956822 ) ) ;
#35644=ORIENTED_EDGE ( 'NONE', *, *, #11558, .F. ) ;
#35649=CARTESIAN_POINT ( 'NONE',  ( 37.13513852234969193, 3.604726614523243278, 162.7885495010082764 ) ) ;
#35656=CARTESIAN_POINT ( 'NONE',  ( 25.07300988058480229, -3.604726614523240613, 168.1916436865136291 ) ) ;
#35665=ORIENTED_EDGE ( 'NONE', *, *, #6147, .T. ) ;
#35667=( BOUNDED_CURVE ( )  B_SPLINE_CURVE ( 2, ( #2608, #37288, #14182, #11336, #20063, #32165, #35753 ),
 .UNSPECIFIED., .F., .F. ) 
 B_SPLINE_CURVE_WITH_KNOTS ( ( 3, 2, 2, 3 ),
 ( 0.1304347826086954820, 0.1376811594202895783, 0.1449275362318836746, 0.1521739130434777709 ),
 .UNSPECIFIED. ) 
 CURVE ( )  GEOMETRIC_REPRESENTATION_ITEM ( )  RATIONAL_B_SPLINE_CURVE ( ( 1.000000000000002887, 0.8660254037844354880, 1.000000000000000000, 0.8660254037844387076, 1.000000000000000000, 0.8660254037844479225, 0.9999999999999907851 ) ) 
 REPRESENTATION_ITEM ( '' )  );
#35673=CARTESIAN_POINT ( 'NONE',  ( 18.65685424949248628, -4.000000000000095923, 50.10230395283967653 ) ) ;
#35674=CARTESIAN_POINT ( 'NONE',  ( 15.94236039944520833, 2.966254577781769264, -8.000000000000001776 ) ) ;
#35683=CARTESIAN_POINT ( 'NONE',  ( 15.24356964374999990, 0.000000000000000000, -3.853124999385476812 ) ) ;
#35686=CARTESIAN_POINT ( 'NONE',  ( 26.75643035624999655, 3.323476615752271268, -7.528124999385462424 ) ) ;
#35692=CARTESIAN_POINT ( 'NONE',  ( 33.58116303054575269, 5.196152422706631135, 159.3822117317042455 ) ) ;
#35696=CARTESIAN_POINT ( 'NONE',  ( 15.24356964375000167, -3.323476615752272600, -7.415624999385472371 ) ) ;
#35701=DIRECTION ( 'NONE',  ( 0.08715574274765150453, 0.000000000000000000, 0.9961946980917461003 ) ) ;
#35705=CARTESIAN_POINT ( 'NONE',  ( 27.46224632087531958, 5.407089921784862696, 159.6822773018186297 ) ) ;
#35706=ORIENTED_EDGE ( 'NONE', *, *, #14263, .F. ) ;
#35710=( BOUNDED_CURVE ( )  B_SPLINE_CURVE ( 2, ( #35726, #18127, #17937, #15085, #6177, #26448, #29290 ),
 .UNSPECIFIED., .F., .F. ) 
 B_SPLINE_CURVE_WITH_KNOTS ( ( 3, 2, 2, 3 ),
 ( 0.8695652173913057670, 0.8768115942028998910, 0.8840579710144940151, 0.8913043478260880281 ),
 .UNSPECIFIED. ) 
 CURVE ( )  GEOMETRIC_REPRESENTATION_ITEM ( )  RATIONAL_B_SPLINE_CURVE ( ( 0.9999999999999733546, 0.8660254037844653530, 1.000000000000000000, 0.8660254037844387076, 1.000000000000000000, 0.8660254037844181685, 1.000000000000020428 ) ) 
 REPRESENTATION_ITEM ( '' )  );
#35712=CARTESIAN_POINT ( 'NONE',  ( 15.00000000000000000, 0.000000000000000000, -4.950000000000009948 ) ) ;
#35720=CARTESIAN_POINT ( 'NONE',  ( 21.00000000000000000, -6.928203230275506996, -7.537500000000000533 ) ) ;
#35721=CARTESIAN_POINT ( 'NONE',  ( 18.00000000000000000, 5.196152422706630247, -3.225000000000005862 ) ) ;
#35724=CARTESIAN_POINT ( 'NONE',  ( 30.92676673731498482, 7.209453229046475009, 163.4634630048305439 ) ) ;
#35726=CARTESIAN_POINT ( 'NONE',  ( 24.66770419336863185, 0.000000000000000000, 160.7643302352881278 ) ) ;
#35729=EDGE_LOOP ( 'NONE', ( #9265, #35546, #18593, #20825 ) ) ;
#35730=FACE_OUTER_BOUND ( 'NONE', #27332, .T. ) ;
#35731=CARTESIAN_POINT ( 'NONE',  ( 18.12178482187500350, -4.985214923628407568, -0.5156249993854555846 ) ) ;
#35732=CARTESIAN_POINT ( 'NONE',  ( 33.56808966913361303, -5.196152422706629359, 159.2327825269904622 ) ) ;
#35734=CARTESIAN_POINT ( 'NONE',  ( 21.00000000000000000, 6.646953231504538984, -8.803124999385454785 ) ) ;
#35742=CARTESIAN_POINT ( 'NONE',  ( 34.31327126962603558, -5.196152422706629359, 167.7502471956748877 ) ) ;
#35753=CARTESIAN_POINT ( 'NONE',  ( 37.26917196037089042, 7.347880794884117764E-16, 167.1152069556475510 ) ) ;
#35756=CARTESIAN_POINT ( 'NONE',  ( 37.40967911200478824, 3.604726614523243278, 165.9265627999972992 ) ) ;
#35764=EDGE_CURVE ( 'NONE', #24506, #10376, #9641, .T. ) ;
#35770=CARTESIAN_POINT ( 'NONE',  ( 27.48022219281702405, -5.407089921784859143, 159.8877424583000391 ) ) ;
#35771=CARTESIAN_POINT ( 'NONE',  ( 21.00000000000000000, 6.646953231504538984, -9.703124999385480010 ) ) ;
#35772=CARTESIAN_POINT ( 'NONE',  ( 25.24620043574905282, 0.000000000000000000, 167.3765725426477502 ) ) ;
#35773=CARTESIAN_POINT ( 'NONE',  ( 33.89776776044609363, -5.407089921784861808, 161.6036962298979915 ) ) ;
#35774=CARTESIAN_POINT ( 'NONE',  ( 36.78872592836736288, 7.347880794884125653E-16, 161.6236836811924604 ) ) ;
#35784=CARTESIAN_POINT ( 'NONE',  ( 27.96351228082934171, 5.196152422706630247, 164.0144493178186167 ) ) ;
#35785=EDGE_CURVE ( 'NONE', #31993, #30479, #17381, .T. ) ;
#35787=CARTESIAN_POINT ( 'NONE',  ( 23.87821517812500005, -4.985214923628404016, -6.403124999385473082 ) ) ;
#35801=CARTESIAN_POINT ( 'NONE',  ( 37.17926111711567927, 3.604726614523238837, 163.2928730669172523 ) ) ;
#35812=EDGE_LOOP ( 'NONE', ( #30029, #3563, #30716, #22747 ) ) ;
#35813=CARTESIAN_POINT ( 'NONE',  ( 31.27974749544297595, 7.209453229046475009, 167.4980515321021244 ) ) ;
#35814=CARTESIAN_POINT ( 'NONE',  ( 18.12178482187500350, -4.985214923628407568, -1.865624999385473437 ) ) ;
#35816=EDGE_CURVE ( 'NONE', #33644, #19092, #6979, .T. ) ;
#35819=CARTESIAN_POINT ( 'NONE',  ( 31.12531841381553477, -6.928203230275506996, 165.7329190520329973 ) ) ;
#35828=CARTESIAN_POINT ( 'NONE',  ( 26.75643035624999655, -3.323476615752267715, -0.4031249993854607028 ) ) ;
#35830=CARTESIAN_POINT ( 'NONE',  ( 15.24356964374999990, 0.000000000000000000, -0.2531249993854844949 ) ) ;
#35832=ORIENTED_EDGE ( 'NONE', *, *, #2979, .T. ) ;
#35834=EDGE_LOOP ( 'NONE', ( #1285, #12526 ) ) ;
#35837=CARTESIAN_POINT ( 'NONE',  ( 37.21031035046954116, 7.646167579472024665E-16, 163.6477674281124450 ) ) ;
#35843=CARTESIAN_POINT ( 'NONE',  ( 37.37209319794485651, 7.646167579472015790E-16, 165.4969538364452148 ) ) ;
#35844=ORIENTED_EDGE ( 'NONE', *, *, #11897, .F. ) ;
#35861=FACE_OUTER_BOUND ( 'NONE', #8338, .T. ) ;
#35870=CARTESIAN_POINT ( 'NONE',  ( 18.12178482187500350, -4.985214923628407568, -3.778124999385484628 ) ) ;
#35879=CARTESIAN_POINT ( 'NONE',  ( 30.63506736085999549, 6.928203230275506996, 160.1293238752668913 ) ) ;
#35882=EDGE_CURVE ( 'NONE', #33723, #29149, #21265, .T. ) ;
#35884=CARTESIAN_POINT ( 'NONE',  ( 26.75643035624999655, 7.049594010296217766E-16, -5.878124999385475391 ) ) ;
#35891=EDGE_CURVE ( 'NONE', #33506, #24506, #29199, .T. ) ;
#35908=CARTESIAN_POINT ( 'NONE',  ( 26.99999999999952038, 3.464101615138031054, -3.337499999999980815 ) ) ;
#35911=CARTESIAN_POINT ( 'NONE',  ( 24.75924920669326212, -3.604726614523240613, 164.6053427733833132 ) ) ;
#35918=CARTESIAN_POINT ( 'NONE',  ( 28.48305061405702787, 5.725134515572933402, 159.4403097883559894 ) ) ;
#35919=CARTESIAN_POINT ( 'NONE',  ( 26.75643035624999655, 7.049594010296217766E-16, -1.265624999385456251 ) ) ;
#35922=CARTESIAN_POINT ( 'NONE',  ( 20.99999999999999645, 6.928203230275506996, -4.612499999999980282 ) ) ;
#35923=CARTESIAN_POINT ( 'NONE',  ( 23.87821517812499650, 4.985214923628404904, -7.940624999385470062 ) ) ;
#35926=DIRECTION ( 'NONE',  ( 0.9961946980917459893, 0.000000000000000000, -0.08715574274765348906 ) ) ;
#35930=CARTESIAN_POINT ( 'NONE',  ( 34.28712454680172783, 5.196152422706631135, 167.4513887862474064 ) ) ;
#35941=( BOUNDED_CURVE ( )  B_SPLINE_CURVE ( 2, ( #14753, #35019, #9063, #3740, #3561, #703, #20634 ),
 .UNSPECIFIED., .F., .F. ) 
 B_SPLINE_CURVE_WITH_KNOTS ( ( 3, 2, 2, 3 ),
 ( 0.4782608695652166841, 0.4855072463768107527, 0.4927536231884049323, 0.4999999999999990008 ),
 .UNSPECIFIED. ) 
 CURVE ( )  GEOMETRIC_REPRESENTATION_ITEM ( )  RATIONAL_B_SPLINE_CURVE ( ( 1.000000000000013545, 0.8660254037844254960, 1.000000000000000000, 0.8660254037844387076, 1.000000000000000000, 0.8660254037844571373, 0.9999999999999815703 ) ) 
 REPRESENTATION_ITEM ( '' )  );
#35944=CARTESIAN_POINT ( 'NONE',  ( 34.36840877128340566, -5.407089921784861808, 166.9831475995933943 ) ) ;
#35959=CARTESIAN_POINT ( 'NONE',  ( 15.00000000000000000, 0.000000000000000000, -5.399999999999987921 ) ) ;
#35962=CARTESIAN_POINT ( 'NONE',  ( 23.99999999999999645, 5.196152422706631135, -1.049999999999995381 ) ) ;
#35964=CARTESIAN_POINT ( 'NONE',  ( 24.67263818733777470, 0.000000000000000000, 163.6153742921546836 ) ) ;
#35965=CARTESIAN_POINT ( 'NONE',  ( 30.74292259240310443, 6.928203230275514990, 161.3621148129311109 ) ) ;
#35976=EDGE_CURVE ( 'NONE', #31911, #30763, #31047, .T. ) ;
#35977=CARTESIAN_POINT ( 'NONE',  ( 26.75643035624999655, 3.323476615752271712, -6.740624999385494753 ) ) ;
#35981=CARTESIAN_POINT ( 'NONE',  ( 24.00000000000000000, -5.196152422706629359, -6.543749998770942433 ) ) ;
#35991=CARTESIAN_POINT ( 'NONE',  ( 24.67754069786733240, 0.000000000000000000, 163.6714102439223097 ) ) ;
#35996=CARTESIAN_POINT ( 'NONE',  ( 26.99999999999995737, 3.464101615137778811, -2.381249998770954779 ) ) ;
#35997=ADVANCED_FACE ( 'NONE', ( #4323 ), #33327, .T. ) ;
#35999=CARTESIAN_POINT ( 'NONE',  ( 20.99999999999999645, 0.000000000000000000, -8.000000000000000000 ) ) ;
#36002=CARTESIAN_POINT ( 'NONE',  ( 24.87364111904954811, 0.000000000000000000, 165.9128483146287465 ) ) ;
#36003=CARTESIAN_POINT ( 'NONE',  ( 21.00000000000000000, 6.646953231504538984, -2.503124999385450966 ) ) ;
#36004=CARTESIAN_POINT ( 'NONE',  ( 36.83775103377001869, 7.347880794884117764E-16, 162.1840432000934129 ) ) ;
#36005=FACE_OUTER_BOUND ( 'NONE', #9506, .T. ) ;
#36007=CARTESIAN_POINT ( 'NONE',  ( 37.43585731826866692, 0.000000000000000000, 169.0204293145237102 ) ) ;
#36016=CARTESIAN_POINT ( 'NONE',  ( 15.24356964374999990, 3.323476615752268604, -0.6281249993854746139 ) ) ;
#36018=CARTESIAN_POINT ( 'NONE',  ( 18.91622474583366653, 5.725135026351895640, -10.38020280809387863 ) ) ;
#36024=CARTESIAN_POINT ( 'NONE',  ( 37.13187018199665346, 7.646167579472024665E-16, 162.7511921998298590 ) ) ;
#36031=CARTESIAN_POINT ( 'NONE',  ( 34.34716455898865206, 5.407089921784857367, 166.7403251419335390 ) ) ;
#36033=AXIS2_PLACEMENT_3D ( 'NONE', #11495, #31406, #20222 ) ;
#36037=ADVANCED_FACE ( 'NONE', ( #5805 ), #25534, .T. ) ;
#36059=CARTESIAN_POINT ( 'NONE',  ( 21.00000000000000000, 6.646953231504538984, -5.315624999385480720 ) ) ;
#36063=CARTESIAN_POINT ( 'NONE',  ( 18.12178482187499640, 4.985214923628404904, -6.515624999385460470 ) ) ;
#36066=EDGE_CURVE ( 'NONE', #8199, #1229, #5431, .T. ) ;
#36073=CARTESIAN_POINT ( 'NONE',  ( 20.99999999999999645, 0.000000000000000000, -8.000000000000000000 ) ) ;
#36074=CARTESIAN_POINT ( 'NONE',  ( 18.00000000000000355, -5.196152422706632912, -3.018749998770942078 ) ) ;
#36083=ORIENTED_EDGE ( 'NONE', *, *, #31697, .F. ) ;
#36095=AXIS2_PLACEMENT_3D ( 'NONE', #2649, #25592, #5127 ) ;
#36100=CARTESIAN_POINT ( 'NONE',  ( 24.79193261022362549, 3.604726614523236616, 164.9789157851677146 ) ) ;
#36101=CARTESIAN_POINT ( 'NONE',  ( 14.99999999999982414, 3.464101615137652246, -1.837499999999977929 ) ) ;
#36108=CARTESIAN_POINT ( 'NONE',  ( 23.87821517812500005, -4.985214923628404016, -0.4406249993854638447 ) ) ;
#36111=CARTESIAN_POINT ( 'NONE',  ( 26.75643035624999655, 7.049594010296217766E-16, -9.815624999385457627 ) ) ;
#36120=CARTESIAN_POINT ( 'NONE',  ( 31.18414854017020232, 6.928203230275506996, 166.4053504732449085 ) ) ;
#36124=CARTESIAN_POINT ( 'NONE',  ( 18.12178482187500350, -4.985214923628407568, -1.528124999385482852 ) ) ;
#36129=EDGE_LOOP ( 'NONE', ( #27879, #21468, #7249, #15947 ) ) ;
#36133=CARTESIAN_POINT ( 'NONE',  ( 30.92186422678543778, 7.209453229046482114, 163.4074270530628894 ) ) ;
#36147=CARTESIAN_POINT ( 'NONE',  ( 18.00000000000000355, -5.196152422706632912, -2.624999999999988454 ) ) ;
#36148=CARTESIAN_POINT ( 'NONE',  ( 24.67590652769082027, -3.604726614523244610, 163.6527315933331295 ) ) ;
#36149=CARTESIAN_POINT ( 'NONE',  ( 36.74623750377789122, -3.464101615137755275, 161.1380387658727216 ) ) ;
#36154=ORIENTED_EDGE ( 'NONE', *, *, #35816, .F. ) ;
#36157=CARTESIAN_POINT ( 'NONE',  ( 24.00000000000000000, -5.196152422706629359, -3.899999999999987033 ) ) ;
#36159=CARTESIAN_POINT ( 'NONE',  ( 26.75643035624999655, 7.049594010296217766E-16, -7.228124999385493687 ) ) ;
#36171=CARTESIAN_POINT ( 'NONE',  ( 21.00000000000016342, -4.000000000000002665, 50.00000000000000000 ) ) ;
#36172=CARTESIAN_POINT ( 'NONE',  ( 24.64158895398392701, -3.604726614523240613, 163.2604799309594910 ) ) ;
#36174=CARTESIAN_POINT ( 'NONE',  ( 20.99999999999999645, -6.928203230275506996, -0.7875000000000005329 ) ) ;
#36175=CARTESIAN_POINT ( 'NONE',  ( 27.00000000000047251, -3.464101615137475942, -3.806249998770962151 ) ) ;
#36179=( BOUNDED_CURVE ( )  B_SPLINE_CURVE ( 2, ( #29071, #5771, #269, #20010, #34770, #5396, #11286 ),
 .UNSPECIFIED., .F., .F. ) 
 B_SPLINE_CURVE_WITH_KNOTS ( ( 3, 2, 2, 3 ),
 ( 0.1521739130434776044, 0.1594202898550718950, 0.1666666666666661856, 0.1739130434782605039 ),
 .UNSPECIFIED. ) 
 CURVE ( )  GEOMETRIC_REPRESENTATION_ITEM ( )  RATIONAL_B_SPLINE_CURVE ( ( 1.000000000000012212, 0.8660254037844263841, 1.000000000000000000, 0.8660254037844387076, 1.000000000000000000, 0.8660254037844453689, 0.9999999999999933387 ) ) 
 REPRESENTATION_ITEM ( '' )  );
#36184=CARTESIAN_POINT ( 'NONE',  ( 37.14004103287923186, 3.604726614523238837, 162.8445854527759309 ) ) ;
#36186=CARTESIAN_POINT ( 'NONE',  ( 18.12178482187499640, 4.985214923628404904, -5.165624999385470595 ) ) ;
#36197=CARTESIAN_POINT ( 'NONE',  ( 21.00000000000000000, 6.646953231504538984, -3.403124999385474858 ) ) ;
#36199=CARTESIAN_POINT ( 'NONE',  ( 26.99999999999999645, -3.464101615137751278, -9.656249998770976006 ) ) ;
#36203=ORIENTED_EDGE ( 'NONE', *, *, #34648, .F. ) ;
#36207=CARTESIAN_POINT ( 'NONE',  ( 24.47980610650859390, -3.604726614523244610, 161.4112935226266359 ) ) ;
#36209=VECTOR ( 'NONE', #19063, 1000.000000000000000 ) ;
#36220=( BOUNDED_CURVE ( )  B_SPLINE_CURVE ( 2, ( #14461, #22998, #11800, #8587, #26017, #23185, #34732 ),
 .UNSPECIFIED., .F., .F. ) 
 B_SPLINE_CURVE_WITH_KNOTS ( ( 3, 2, 2, 3 ),
 ( 0.1521739130434777709, 0.1594202898550720338, 0.1666666666666663243, 0.1739130434782606149 ),
 .UNSPECIFIED. ) 
 CURVE ( )  GEOMETRIC_REPRESENTATION_ITEM ( )  RATIONAL_B_SPLINE_CURVE ( ( 1.000000000000009326, 0.8660254037844296038, 1.000000000000000000, 0.8660254037844387076, 1.000000000000000000, 0.8660254037844433705, 0.9999999999999953371 ) ) 
 REPRESENTATION_ITEM ( '' )  );
#36224=EDGE_CURVE ( 'NONE', #31196, #9403, #8623, .T. ) ;
#36234=DIRECTION ( 'NONE',  ( 0.000000000000000000, 0.000000000000000000, 1.000000000000000000 ) ) ;
#36236=EDGE_CURVE ( 'NONE', #17991, #20530, #22916, .T. ) ;
#36243=CARTESIAN_POINT ( 'NONE',  ( 26.75643035624999655, 3.323476615752271712, -8.090624999385481075 ) ) ;
#36246=CARTESIAN_POINT ( 'NONE',  ( 18.12178482187499640, 4.985214923628404904, -6.965624999385466865 ) ) ;
#36247=EDGE_CURVE ( 'NONE', #26157, #7551, #2093, .T. ) ;
#36249=CARTESIAN_POINT ( 'NONE',  ( 34.40762885551985306, -5.407089921784861808, 167.4314352137346873 ) ) ;
#36252=CARTESIAN_POINT ( 'NONE',  ( 36.56321044411491528, 7.347880794884117764E-16, 159.0460299011043901 ) ) ;
#36268=EDGE_CURVE ( 'NONE', #13971, #15757, #6514, .T. ) ;
#36276=ORIENTED_EDGE ( 'NONE', *, *, #32573, .T. ) ;
#36281=CARTESIAN_POINT ( 'NONE',  ( 24.83442103481310781, 0.000000000000000000, 165.4645607004874535 ) ) ;
#36284=VERTEX_POINT ( 'NONE', #9595 ) ;
#36289=CARTESIAN_POINT ( 'NONE',  ( 26.99999999999999645, 3.464101615137755275, -5.081249998770961618 ) ) ;
#36292=CARTESIAN_POINT ( 'NONE',  ( 18.12178482187499640, 4.985214923628404904, -9.665624999385475036 ) ) ;
#36296=CARTESIAN_POINT ( 'NONE',  ( 36.80179928988602711, 3.464101615138092782, 161.7731128871306225 ) ) ;
#36299=CARTESIAN_POINT ( 'NONE',  ( 28.19883278624800127, 5.196152422706630247, 166.7041750026663181 ) ) ;
#36304=CARTESIAN_POINT ( 'NONE',  ( 23.87821517812500005, -4.985214923628404016, -1.003124999385485161 ) ) ;
#36308=ORIENTED_EDGE ( 'NONE', *, *, #12969, .F. ) ;
#36312=CARTESIAN_POINT ( 'NONE',  ( 26.99999999999999289, 0.000000000000000000, -8.000000000000000000 ) ) ;
#36313=CARTESIAN_POINT ( 'NONE',  ( 24.78703009969406779, 3.604726614523240613, 164.9228798334000601 ) ) ;
#36331=CARTESIAN_POINT ( 'NONE',  ( 23.99999999999999645, 5.196152422706631135, -1.500000000000001332 ) ) ;
#36332=CARTESIAN_POINT ( 'NONE',  ( 33.97620792891898134, -5.407089921784861808, 162.5002714581805492 ) ) ;
#36333=CARTESIAN_POINT ( 'NONE',  ( 36.66779733530500351, -3.464101615137755275, 160.2414635375901355 ) ) ;
#36339=B_SPLINE_CURVE_WITH_KNOTS ( 'NONE', 1,
 ( #24998, #13077 ),
 .UNSPECIFIED., .F., .F.,
 ( 2, 2 ),
 ( 0.000000000000000000, 1.000000000000000000 ),
 .UNSPECIFIED. ) ;
#36344=CARTESIAN_POINT ( 'NONE',  ( 18.12178482187500350, -4.985214923628407568, -5.578124999385480898 ) ) ;
#36358=CARTESIAN_POINT ( 'NONE',  ( 36.97662401522738662, -3.604726614523235284, 160.9767203938538955 ) ) ;
#36359=CARTESIAN_POINT ( 'NONE',  ( 25.21351703232559061, 3.464101615137630485, 167.0029995320877845 ) ) ;
#36361=CARTESIAN_POINT ( 'NONE',  ( 24.00000000000000000, -5.196152422706629359, -0.7500000000000006661 ) ) ;
#36371=CARTESIAN_POINT ( 'NONE',  ( 31.00520690578787253, 7.209453229046475009, 164.3600382331131868 ) ) ;
#36372=CARTESIAN_POINT ( 'NONE',  ( 18.12178482187500350, -4.985214923628407568, -5.015624999385459581 ) ) ;
#36374=CARTESIAN_POINT ( 'NONE',  ( 31.33122385594975512, 6.928203230275514990, 168.0864290250504212 ) ) ;
#36384=CARTESIAN_POINT ( 'NONE',  ( 15.24356964374999990, 0.000000000000000000, -4.640624999385472904 ) ) ;
#36388=CARTESIAN_POINT ( 'NONE',  ( 26.99999999999999645, 3.464101615137755275, -9.581249998770951848 ) ) ;
#36394=CARTESIAN_POINT ( 'NONE',  ( 24.47653776615555898, 0.000000000000000000, 161.3739362214482469 ) ) ;
#36403=FACE_OUTER_BOUND ( 'NONE', #35729, .T. ) ;
#36409=ORIENTED_EDGE ( 'NONE', *, *, #30444, .T. ) ;
#36415=CARTESIAN_POINT ( 'NONE',  ( 24.00000000000000000, -5.196152422706629359, -5.700000000000010836 ) ) ;
#36427=CARTESIAN_POINT ( 'NONE',  ( 21.00000000000000000, -6.646953231504538984, -7.340624999385477523 ) ) ;
#36430=CARTESIAN_POINT ( 'NONE',  ( 15.24356964375000167, -3.323476615752272600, -7.753124999385476279 ) ) ;
#36432=EDGE_CURVE ( 'NONE', #14950, #34407, #24188, .T. ) ;
#36433=CARTESIAN_POINT ( 'NONE',  ( 25.21845102629493951, 3.604726614523240613, 169.8540435889542550 ) ) ;
#36436=AXIS2_PLACEMENT_3D ( 'NONE', #2850, #37164, #11390 ) ;
#36438=DIRECTION ( 'NONE',  ( 1.000000000000000000, 0.000000000000000000, 0.000000000000000000 ) ) ;
#36443=CARTESIAN_POINT ( 'NONE',  ( 33.80341017455227615, -5.196152422706629359, 161.9225082118381920 ) ) ;
#36464=CARTESIAN_POINT ( 'NONE',  ( 26.97716818855048260, 0.000000000000000000, 49.47706554351410801 ) ) ;
#36468=CARTESIAN_POINT ( 'NONE',  ( 27.79398286670857132, -5.407089921784859143, 163.4740433714303265 ) ) ;
#36469=FACE_OUTER_BOUND ( 'NONE', #31507, .T. ) ;
#36472=EDGE_LOOP ( 'NONE', ( #5145, #13021, #24606 ) ) ;
#36474=EDGE_LOOP ( 'NONE', ( #19729, #18974, #36409, #6943 ) ) ;
#36476=CARTESIAN_POINT ( 'NONE',  ( 24.00000000000000000, -5.196152422706629359, -3.843749998770962240 ) ) ;
#36477=CARTESIAN_POINT ( 'NONE',  ( 26.75643035624999655, 7.049594010296217766E-16, -0.3656249993854721048 ) ) ;
#36479=CARTESIAN_POINT ( 'NONE',  ( 20.99999999999999645, 6.928203230275506996, -5.962500000000000355 ) ) ;
#36487=CARTESIAN_POINT ( 'NONE',  ( 31.08609832957909092, -6.928203230275506996, 165.2846314378917043 ) ) ;
#36489=EDGE_CURVE ( 'NONE', #35077, #28874, #36734, .T. ) ;
#36492=CARTESIAN_POINT ( 'NONE',  ( 26.75643035624999655, 3.323476615752271268, -1.790624999385477256 ) ) ;
#36496=EDGE_CURVE ( 'NONE', #24223, #14024, #33096, .T. ) ;
#36498=CARTESIAN_POINT ( 'NONE',  ( 24.88995133726761111, 3.464101615137512358, 163.3046267141977808 ) ) ;
#36501=CARTESIAN_POINT ( 'NONE',  ( 34.22460179574976991, 5.407089921784862696, 165.3394263477420054 ) ) ;
#36503=VECTOR ( 'NONE', #21875, 1000.000000000000000 ) ;
#36505=EDGE_CURVE ( 'NONE', #15426, #12608, #30671, .T. ) ;
#36508=CARTESIAN_POINT ( 'NONE',  ( 26.99999999999999645, 7.347880794884117764E-16, -2.868749998770958598 ) ) ;
#36518=CARTESIAN_POINT ( 'NONE',  ( 26.99999999999999645, -3.464101615137751278, -1.162500000000002309 ) ) ;
#36519=CARTESIAN_POINT ( 'NONE',  ( 27.73678691053042300, 5.407089921784862696, 162.8202906008076241 ) ) ;
#36520=CARTESIAN_POINT ( 'NONE',  ( 36.67106567565804198, 7.347880794884125653E-16, 160.2788208387686097 ) ) ;
#36523=EDGE_CURVE ( 'NONE', #14391, #13208, #30440, .T. ) ;
#36531=CARTESIAN_POINT ( 'NONE',  ( 18.12178482187500350, -4.985214923628407568, -9.628124999385478944 ) ) ;
#36533=AXIS2_PLACEMENT_3D ( 'NONE', #17500, #2527, #2889 ) ;
#36545=CARTESIAN_POINT ( 'NONE',  ( 26.99999999999999645, 7.347880794884117764E-16, -1.968749998770946696 ) ) ;
#36546=CARTESIAN_POINT ( 'NONE',  ( 27.75476278247212747, -5.407089921784859143, 163.0257557572890335 ) ) ;
#36552=CARTESIAN_POINT ( 'NONE',  ( 15.00000000000000000, 0.000000000000000000, -7.593749998770965348 ) ) ;
#36557=CARTESIAN_POINT ( 'NONE',  ( 34.05955060792140188, -5.407089921784855591, 163.4528826382307614 ) ) ;
#36558=CARTESIAN_POINT ( 'NONE',  ( 26.75643035624999655, -3.323476615752267715, -5.803124999385441463 ) ) ;
#36561=CARTESIAN_POINT ( 'NONE',  ( 34.30346624845981296, -5.196152422706635576, 167.6381752909151999 ) ) ;
#36567=ORIENTED_EDGE ( 'NONE', *, *, #36523, .T. ) ;
#36573=CARTESIAN_POINT ( 'NONE',  ( 23.87821517812499650, 4.985214923628404904, -2.990624999385460558 ) ) ;
#36575=ADVANCED_FACE ( 'NONE', ( #7135 ), #1988, .T. ) ;
#36577=CARTESIAN_POINT ( 'NONE',  ( 15.00000000000000000, 0.000000000000000000, -10.29374999877094510 ) ) ;
#36604=CYLINDRICAL_SURFACE ( 'NONE', #33513, 6.000000000000001776 ) ;
#36615=CARTESIAN_POINT ( 'NONE',  ( 21.00000000000000000, -6.646953231504538984, -6.890624999385480898 ) ) ;
#36617=ORIENTED_EDGE ( 'NONE', *, *, #88, .T. ) ;
#36621=CARTESIAN_POINT ( 'NONE',  ( 28.29894145125277660, -5.407089921784865361, 169.2457464034993961 ) ) ;
#36623=( BOUNDED_CURVE ( )  B_SPLINE_CURVE ( 3, ( #2658, #33949, #14175, #31784 ),
 .UNSPECIFIED., .F., .F. ) 
 B_SPLINE_CURVE_WITH_KNOTS ( ( 4, 4 ),
 ( 0.000000000000000000, 1.570796326794856812 ),
 .UNSPECIFIED. ) 
 CURVE ( )  GEOMETRIC_REPRESENTATION_ITEM ( )  RATIONAL_B_SPLINE_CURVE ( ( 1.000000000000000000, 0.8047378541243743744, 0.8047378541243743744, 1.000000000000000000 ) ) 
 REPRESENTATION_ITEM ( '' )  );
#36636=CARTESIAN_POINT ( 'NONE',  ( 14.99999999999972466, -3.464101615137598067, -0.4125000000000021982 ) ) ;
#36648=CARTESIAN_POINT ( 'NONE',  ( 37.25936693920468201, 7.347880794884125653E-16, 167.0031350508878631 ) ) ;
#36660=CARTESIAN_POINT ( 'NONE',  ( 33.87652354815133293, 5.407089921784857367, 161.3608737722381079 ) ) ;
#36665=ORIENTED_EDGE ( 'NONE', *, *, #6720, .T. ) ;
#36667=CARTESIAN_POINT ( 'NONE',  ( 26.99999999999999645, 7.347880794884117764E-16, -5.118749998770960374 ) ) ;
#36668=CARTESIAN_POINT ( 'NONE',  ( 18.12178482187499640, 4.985214923628404904, -2.015624999385456917 ) ) ;
#36671=CARTESIAN_POINT ( 'NONE',  ( 21.00000000000000355, 0.000000000000000000, 50.00000000000001421 ) ) ;
#36679=CARTESIAN_POINT ( 'NONE',  ( 30.90960795051509891, 6.928203230275506996, 163.2673371742559141 ) ) ;
#36683=CARTESIAN_POINT ( 'NONE',  ( 18.12178482187499640, 4.985214923628404904, -1.228124999385488136 ) ) ;
#36691=CARTESIAN_POINT ( 'NONE',  ( 21.00000000000016342, 4.000000000000002665, 50.00000000000000000 ) ) ;
#36692=CARTESIAN_POINT ( 'NONE',  ( 24.83278686463658502, -3.604726614523244610, 165.4458820498982163 ) ) ;
#36697=CARTESIAN_POINT ( 'NONE',  ( 15.00000000000010658, 3.464101615137812562, -2.681249998770963483 ) ) ;
#36707=ORIENTED_EDGE ( 'NONE', *, *, #32855, .T. ) ;
#36708=CARTESIAN_POINT ( 'NONE',  ( 26.99999999999999645, -3.464101615137751278, -2.512499999999989075 ) ) ;
#36710=CARTESIAN_POINT ( 'NONE',  ( 27.54068648934820729, 5.407089921784862696, 160.5788525301012157 ) ) ;
#36712=CARTESIAN_POINT ( 'NONE',  ( 30.60565229757555272, -6.928203230275514990, 159.7931081634365853 ) ) ;
#36718=ORIENTED_EDGE ( 'NONE', *, *, #2636, .F. ) ;
#36722=CARTESIAN_POINT ( 'NONE',  ( 15.24356964375000167, -3.323476615752272600, -8.315624999385494931 ) ) ;
#36725=ADVANCED_FACE ( 'NONE', ( #27396 ), #1427, .T. ) ;
#36726=CARTESIAN_POINT ( 'NONE',  ( 25.47825260081467391, 3.464101615137757051, 170.0289409263170626 ) ) ;
#36734=( BOUNDED_CURVE ( )  B_SPLINE_CURVE ( 2, ( #33277, #18889, #13371, #36479, #4274, #16599, #4830 ),
 .UNSPECIFIED., .F., .F. ) 
 B_SPLINE_CURVE_WITH_KNOTS ( ( 3, 2, 2, 3 ),
 ( 0.5652173913043473386, 0.5724637681159415736, 0.5797101449275359197, 0.5869565217391301548 ),
 .UNSPECIFIED. ) 
 CURVE ( )  GEOMETRIC_REPRESENTATION_ITEM ( )  RATIONAL_B_SPLINE_CURVE ( ( 1.000000000000008216, 0.8660254037844304920, 1.000000000000000000, 0.8660254037844387076, 1.000000000000000000, 0.8660254037844448138, 0.9999999999999938938 ) ) 
 REPRESENTATION_ITEM ( '' )  );
#36735=CARTESIAN_POINT ( 'NONE',  ( 28.07136751237244354, 5.196152422706636465, 165.2472402554827795 ) ) ;
#36736=CARTESIAN_POINT ( 'NONE',  ( 30.69144623189632526, 7.209453229046475009, 160.7737373199828426 ) ) ;
#36739=CARTESIAN_POINT ( 'NONE',  ( 30.60565229757555628, -6.928203230275514990, 159.7931081634365853 ) ) ;
#36740=CARTESIAN_POINT ( 'NONE',  ( 36.68087069682425039, 7.347880794884117764E-16, 160.3908927435282692 ) ) ;
#36746=EDGE_LOOP ( 'NONE', ( #13389, #32825, #35832, #10426 ) ) ;
#36747=CARTESIAN_POINT ( 'NONE',  ( 37.21848120135211957, 3.604726614523238837, 163.7411606810585454 ) ) ;
#36748=CARTESIAN_POINT ( 'NONE',  ( 23.87821517812500005, -4.985214923628404016, -5.390624999385473792 ) ) ;
#36752=CARTESIAN_POINT ( 'NONE',  ( 25.43903251657823006, 3.464101615137757051, 169.5806533121757695 ) ) ;
#36761=DIRECTION ( 'NONE',  ( 0.08715574274765150453, 0.000000000000000000, 0.9961946980917461003 ) ) ;
#36762=CARTESIAN_POINT ( 'NONE',  ( 21.00000000000000000, 6.646953231504538984, -2.953124999385479565 ) ) ;
#36765=CARTESIAN_POINT ( 'NONE',  ( 18.12178482187499640, 4.985214923628404904, -2.128124999385472282 ) ) ;
#36778=B_SPLINE_CURVE_WITH_KNOTS ( 'NONE', 3,
 ( #2984, #35010, #139, #3550, #17406, #11702, #6011, #12074, #20813, #17595, #29126, #23649, #32166, #14741, #17220, #12266, #9240, #32355 ),
 .UNSPECIFIED., .F., .F.,
 ( 4, 2, 2, 2, 2, 2, 2, 2, 4 ),
 ( 0.000000000000000000, 0.001127056113610278064, 0.002254112227220556128, 0.003381168340830834410, 0.004508224454441112257, 0.005635280568051390104, 0.006762336681661668819, 0.007889392795271945799, 0.009016448908882224514 ),
 .UNSPECIFIED. ) ;
#36789=CARTESIAN_POINT ( 'NONE',  ( 20.99999999999999645, 6.928203230275506996, -2.812499999999997335 ) ) ;
#36791=CARTESIAN_POINT ( 'NONE',  ( 24.00000000000000000, -5.196152422706629359, -1.593749998770960241 ) ) ;
#36792=EDGE_CURVE ( 'NONE', #13953, #805, #34524, .T. ) ;
#36795=CARTESIAN_POINT ( 'NONE',  ( 21.00000000000000000, -6.928203230275506996, -8.437499999999991118 ) ) ;
#36801=CARTESIAN_POINT ( 'NONE',  ( 26.75643035624999655, 7.049594010296217766E-16, -6.778124999385487293 ) ) ;
#36805=VECTOR ( 'NONE', #33915, 1000.000000000000000 ) ;
#36808=CARTESIAN_POINT ( 'NONE',  ( 25.14001085782205891, 3.604726614523240613, 168.9574683606716690 ) ) ;
#36810=CARTESIAN_POINT ( 'NONE',  ( 37.38356387272733627, -3.464101615137664236, 168.4227124968929559 ) ) ;
#36826=CYLINDRICAL_SURFACE ( 'NONE', #13760, 6.000000000000001776 ) ;
#36831=CARTESIAN_POINT ( 'NONE',  ( 37.10248660225891371, 7.347880794884125653E-16, 165.2099845943227479 ) ) ;
#36843=CARTESIAN_POINT ( 'NONE',  ( 33.83730346391489263, 5.407089921784857367, 160.9125861580968149 ) ) ;
#36844=CARTESIAN_POINT ( 'NONE',  ( 23.87821517812499650, 4.985214923628404904, -0.4031249993854957303 ) ) ;
#36849=CARTESIAN_POINT ( 'NONE',  ( 21.00000000000000000, -6.928203230275506996, -3.881249998770961884 ) ) ;
#36850=CARTESIAN_POINT ( 'NONE',  ( 26.75643035624999655, 3.323476615752271268, -3.028124999385441107 ) ) ;
#36852=DIRECTION ( 'NONE',  ( 1.000000000000000000, 0.000000000000000000, 0.000000000000000000 ) ) ;
#36859=CARTESIAN_POINT ( 'NONE',  ( 31.10570837169731817, 6.928203230275506996, 165.5087752449623224 ) ) ;
#36863=CARTESIAN_POINT ( 'NONE',  ( 23.87821517812499650, 4.985214923628404904, -0.8531249993854739255 ) ) ;
#36867=VERTEX_POINT ( 'NONE', #5384 ) ;
#36872=CARTESIAN_POINT ( 'NONE',  ( 27.90674060888834518, -5.407089921784865361, 164.7628702620865226 ) ) ;
#36877=CARTESIAN_POINT ( 'NONE',  ( 36.67760235647196509, -3.464101615137322288, 160.3535354423497949 ) ) ;
#36882=DIRECTION ( 'NONE',  ( 0.08715574274765150453, 0.000000000000000000, 0.9961946980917461003 ) ) ;
#36887=CARTESIAN_POINT ( 'NONE',  ( 15.00000000000000000, 3.464101615137752166, -2.737500000000003375 ) ) ;
#36888=( BOUNDED_CURVE ( )  B_SPLINE_CURVE ( 2, ( #18018, #7208, #32782, #21055, #30131, #35996, #35431 ),
 .UNSPECIFIED., .F., .F. ) 
 B_SPLINE_CURVE_WITH_KNOTS ( ( 3, 2, 2, 3 ),
 ( 0.1739130434782605039, 0.1811594202898547945, 0.1884057971014491129, 0.1956521739130434034 ),
 .UNSPECIFIED. ) 
 CURVE ( )  GEOMETRIC_REPRESENTATION_ITEM ( )  RATIONAL_B_SPLINE_CURVE ( ( 1.000000000000006661, 0.8660254037844320463, 1.000000000000000000, 0.8660254037844387076, 1.000000000000000000, 0.8660254037844402619, 0.9999999999999984457 ) ) 
 REPRESENTATION_ITEM ( '' )  );
#36889=CARTESIAN_POINT ( 'NONE',  ( 20.96843863229867821, -5.998110342775703430, -8.000000000000003553 ) ) ;
#36890=CARTESIAN_POINT ( 'NONE',  ( 24.51902619074504130, -3.604726614523244610, 161.8595811367679573 ) ) ;
#36892=CARTESIAN_POINT ( 'NONE',  ( 37.60414536301047406, -3.604726614523235284, 168.1493222201144704 ) ) ;
#36895=ORIENTED_EDGE ( 'NONE', *, *, #352, .F. ) ;
#36900=CARTESIAN_POINT ( 'NONE',  ( 15.24356964374999990, 0.000000000000000000, -10.15312499938547575 ) ) ;
#36913=CARTESIAN_POINT ( 'NONE',  ( 30.80910648460565682, 7.209453229046475009, 162.1186001624066932 ) ) ;
#36917=AXIS2_PLACEMENT_3D ( 'NONE', #19205, #33591, #36980 ) ;
#36925=ORIENTED_EDGE ( 'NONE', *, *, #7484, .T. ) ;
#36926=CARTESIAN_POINT ( 'NONE',  ( 24.60236886974748671, -3.604726614523240613, 162.8121923168181695 ) ) ;
#36927=CARTESIAN_POINT ( 'NONE',  ( 21.00000000000000000, -6.646953231504538984, -6.328124999385495997 ) ) ;
#36930=CARTESIAN_POINT ( 'NONE',  ( 25.06157068934917120, 3.604726614523240613, 168.0608931323890829 ) ) ;
#36932=CARTESIAN_POINT ( 'NONE',  ( 25.20698035151260896, 0.000000000000000000, 166.9282849285064856 ) ) ;
#36943=CARTESIAN_POINT ( 'NONE',  ( 23.87821517812500005, -4.985214923628404016, -4.940624999385468286 ) ) ;
#36946=CARTESIAN_POINT ( 'NONE',  ( 15.24356964374999990, 3.323476615752268604, -0.7406249993854975289 ) ) ;
#36951=( BOUNDED_CURVE ( )  B_SPLINE_CURVE ( 3, ( #35483, #35673, #18258, #30377 ),
 .UNSPECIFIED., .F., .F. ) 
 B_SPLINE_CURVE_WITH_KNOTS ( ( 4, 4 ),
 ( 4.712388980384648818, 6.283185307179586232 ),
 .UNSPECIFIED. ) 
 CURVE ( )  GEOMETRIC_REPRESENTATION_ITEM ( )  RATIONAL_B_SPLINE_CURVE ( ( 1.000000000000000000, 0.8047378541243555006, 0.8047378541243555006, 1.000000000000000000 ) ) 
 REPRESENTATION_ITEM ( '' )  );
#36955=EDGE_CURVE ( 'NONE', #19175, #11807, #19823, .T. ) ;
#36961=DIRECTION ( 'NONE',  ( 0.9961946980917462113, 0.000000000000000000, -0.08715574274765118534 ) ) ;
#36966=EDGE_CURVE ( 'NONE', #8971, #590, #5956, .T. ) ;
#36967=CARTESIAN_POINT ( 'NONE',  ( 26.99999999999999645, 7.347880794884117764E-16, -2.418749998770952647 ) ) ;
#36977=DIRECTION ( 'NONE',  ( 0.08715574274765150453, 0.000000000000000000, 0.9961946980917461003 ) ) ;
#36980=DIRECTION ( 'NONE',  ( 1.000000000000000000, 0.000000000000000000, -0.000000000000000000 ) ) ;
#36982=CARTESIAN_POINT ( 'NONE',  ( 18.00000000000000000, 5.196152422706630247, -8.624999999999992895 ) ) ;
#36983=EDGE_LOOP ( 'NONE', ( #2995, #16085, #18555, #25920 ) ) ;
#36987=CARTESIAN_POINT ( 'NONE',  ( 23.87821517812500005, -4.985214923628404016, -7.753124999385491378 ) ) ;
#36990=ORIENTED_EDGE ( 'NONE', *, *, #13782, .F. ) ;
#36993=CARTESIAN_POINT ( 'NONE',  ( 25.10732745429168489, -3.604726614523244610, 168.5838953488872676 ) ) ;
#36997=ADVANCED_FACE ( 'NONE', ( #29770 ), #26928, .F. ) ;
#37002=CARTESIAN_POINT ( 'NONE',  ( 28.30668801779110311, 5.196152422706636465, 167.9369659403305093 ) ) ;
#37006=VECTOR ( 'NONE', #17132, 1000.000000000000000 ) ;
#37011=ORIENTED_EDGE ( 'NONE', *, *, #26262, .F. ) ;
#37013=AXIS2_PLACEMENT_3D ( 'NONE', #19847, #25511, #8637 ) ;
#37016=CARTESIAN_POINT ( 'NONE',  ( 15.00000000000047606, 3.464101615138028389, -5.381249998770973875 ) ) ;
#37027=CARTESIAN_POINT ( 'NONE',  ( 27.74168942105997360, 5.407089921784856479, 162.8763265525752786 ) ) ;
#37032=ORIENTED_EDGE ( 'NONE', *, *, #4375, .T. ) ;
#37033=CARTESIAN_POINT ( 'NONE',  ( 26.99999999999999645, -3.464101615137751278, -5.606249998770950427 ) ) ;
#37034=CARTESIAN_POINT ( 'NONE',  ( 26.75643035624999655, 7.049594010296217766E-16, -2.165624999385467930 ) ) ;
#37036=CARTESIAN_POINT ( 'NONE',  ( 37.25936693920468201, 7.347880794884125653E-16, 167.0031350508878631 ) ) ;
#37037=CARTESIAN_POINT ( 'NONE',  ( 15.24356964374999990, 3.323476615752268604, -10.07812499938544804 ) ) ;
#37045=CARTESIAN_POINT ( 'NONE',  ( 30.94882803475154986, 6.928203230275506996, 163.7156247883972355 ) ) ;
#37050=CARTESIAN_POINT ( 'NONE',  ( 15.24356964374999990, 3.323476615752268604, -4.790624999385491023 ) ) ;
#37060=CARTESIAN_POINT ( 'NONE',  ( 37.13513852234969193, 3.604726614523243278, 162.7885495010082764 ) ) ;
#37074=CARTESIAN_POINT ( 'NONE',  ( 26.99999999999999645, 3.464101615137755275, -5.137500000000001066 ) ) ;
#37077=CARTESIAN_POINT ( 'NONE',  ( 24.47326942580252407, 3.604726614523240613, 161.3365789202697727 ) ) ;
#37079=CARTESIAN_POINT ( 'NONE',  ( 36.63184559142159458, 7.347880794884125653E-16, 159.8305332246273167 ) ) ;
#37083=ORIENTED_EDGE ( 'NONE', *, *, #5826, .T. ) ;
#37088=CARTESIAN_POINT ( 'NONE',  ( 26.75643035624999655, -3.323476615752267715, -8.165624999385475036 ) ) ;
#37091=CARTESIAN_POINT ( 'NONE',  ( 15.00000000000000000, 0.000000000000000000, -7.200000000000011724 ) ) ;
#37092=CARTESIAN_POINT ( 'NONE',  ( 24.63668644345436931, -3.604726614523244610, 163.2044439791918080 ) ) ;
#37103=CARTESIAN_POINT ( 'NONE',  ( 25.18249928241153413, 0.000000000000000000, 169.4431132759913794 ) ) ;
#37114=CARTESIAN_POINT ( 'NONE',  ( 30.86793661096032082, -7.209453229046475009, 162.7910315836186328 ) ) ;
#37115=CARTESIAN_POINT ( 'NONE',  ( 18.12178482187500350, -4.985214923628407568, -6.815624999385455851 ) ) ;
#37117=CARTESIAN_POINT ( 'NONE',  ( 25.06810737005524103, -3.604726614523244610, 168.1356077347459461 ) ) ;
#37118=CARTESIAN_POINT ( 'NONE',  ( 31.11551339264931570, -6.928203230275514990, 165.6208471472733095 ) ) ;
#37119=CARTESIAN_POINT ( 'NONE',  ( 26.99999999999999645, 7.347880794884117764E-16, -0.2250000000000029754 ) ) ;
#37132=CARTESIAN_POINT ( 'NONE',  ( 23.87821517812500005, -4.985214923628404016, -1.903124999385497063 ) ) ;
#37139=ADVANCED_FACE ( 'NONE', ( #3175 ), #5835, .T. ) ;
#37162=FACE_OUTER_BOUND ( 'NONE', #1602, .T. ) ;
#37164=DIRECTION ( 'NONE',  ( 0.000000000000000000, 0.000000000000000000, 1.000000000000000000 ) ) ;
#37167=DIRECTION ( 'NONE',  ( 0.08715574274765150453, 0.000000000000000000, 0.9961946980917461003 ) ) ;
#37169=CARTESIAN_POINT ( 'NONE',  ( 26.99999999999999645, 7.347880794884117764E-16, -8.324999999999999289 ) ) ;
#37174=CARTESIAN_POINT ( 'NONE',  ( 15.24356964374999990, 0.000000000000000000, -8.803124999385486760 ) ) ;
#37180=CARTESIAN_POINT ( 'NONE',  ( 24.91122703310946918, -3.604726614523244610, 166.3424572781808024 ) ) ;
#37186=CARTESIAN_POINT ( 'NONE',  ( 31.33857762179763995, -7.209453229046475009, 168.1704829533140355 ) ) ;
#37188=LINE ( 'NONE', #26186, #8271 ) ;
#37189=CYLINDRICAL_SURFACE ( 'NONE', #33142, 5.999999999999994671 ) ;
#37200=CARTESIAN_POINT ( 'NONE',  ( 34.24790446256528753, 5.196152422706631135, 167.0031011721061134 ) ) ;
#37214=CARTESIAN_POINT ( 'NONE',  ( 24.51739202056851852, 3.604726614523236616, 161.8409024861786918 ) ) ;
#37215=VECTOR ( 'NONE', #17884, 1000.000000000000000 ) ;
#37220=VERTEX_POINT ( 'NONE', #14561 ) ;
#37221=ORIENTED_EDGE ( 'NONE', *, *, #6337, .F. ) ;
#37222=CARTESIAN_POINT ( 'NONE',  ( 15.00000000000000000, 3.464101615137752166, -6.731249998770956644 ) ) ;
#37223=CARTESIAN_POINT ( 'NONE',  ( 18.12178482187500350, -4.985214923628407568, -2.765624999385457805 ) ) ;
#37225=DIRECTION ( 'NONE',  ( 0.000000000000000000, 0.000000000000000000, 1.000000000000000000 ) ) ;
#37231=CARTESIAN_POINT ( 'NONE',  ( 36.91292286188986793, -3.464101615137751278, 163.0432611271975532 ) ) ;
#37235=CARTESIAN_POINT ( 'NONE',  ( 26.75643035624999655, -3.323476615752267271, -4.115624999385481431 ) ) ;
#37240=CARTESIAN_POINT ( 'NONE',  ( 26.97716818855048260, 0.000000000000000000, 49.47706554351410801 ) ) ;
#37245=CARTESIAN_POINT ( 'NONE',  ( 36.97172150469783958, -3.604726614523238837, 160.9206844420862694 ) ) ;
#37259=CARTESIAN_POINT ( 'NONE',  ( 18.00000000000000355, -5.196152422706632912, -3.975000000000006306 ) ) ;
#37262=CARTESIAN_POINT ( 'NONE',  ( 30.60810355289388696, 7.209453229046482114, 159.8211261399325736 ) ) ;
#37264=CARTESIAN_POINT ( 'NONE',  ( 25.10896162446820412, 0.000000000000000000, 168.6025739994764479 ) ) ;
#37274=CARTESIAN_POINT ( 'NONE',  ( 21.00000000000000000, -6.646953231504538984, -9.140624999385492444 ) ) ;
#37279=CARTESIAN_POINT ( 'NONE',  ( 27.67142010346968561, -5.407089921784865361, 162.0731445772388213 ) ) ;
#37288=CARTESIAN_POINT ( 'NONE',  ( 25.33117728503505361, 3.464101615137705981, 168.3478623745115783 ) ) ;
#37290=CARTESIAN_POINT ( 'NONE',  ( 30.63261610554165770, -7.209453229046475009, 160.1013058987709030 ) ) ;
#37291=CARTESIAN_POINT ( 'NONE',  ( 15.00000000000000178, -3.464101615137757051, -3.506249998770959664 ) ) ;
#37300=CARTESIAN_POINT ( 'NONE',  ( 27.78090950529641745, 5.407089921784856479, 163.3246141667165716 ) ) ;
#37301=CARTESIAN_POINT ( 'NONE',  ( 15.24356964374999990, 0.000000000000000000, -7.340624999385481075 ) ) ;
#37303=CARTESIAN_POINT ( 'NONE',  ( 37.56655944895057075, 3.604726614523243278, 167.7197132565624713 ) ) ;
#37304=CARTESIAN_POINT ( 'NONE',  ( 25.12854018303972126, 0.000000000000000000, 166.0317097002238995 ) ) ;
#37305=CARTESIAN_POINT ( 'NONE',  ( 15.00000000000000000, 0.000000000000000000, -5.849999999999994316 ) ) ;
#37317=CARTESIAN_POINT ( 'NONE',  ( 23.87821517812499650, 4.985214923628404904, -1.303124999385479876 ) ) ;
#37335=VERTEX_POINT ( 'NONE', #35385 ) ;
#37336=CARTESIAN_POINT ( 'NONE',  ( 31.39740774815230751, 7.209453229046475009, 168.8429143745259751 ) ) ;
#37338=CARTESIAN_POINT ( 'NONE',  ( 15.24356964374999990, 0.000000000000000000, -0.1406249993854691294 ) ) ;
#37345=CARTESIAN_POINT ( 'NONE',  ( 25.17102860762938832, -3.464101615137868073, 166.5173546155435815 ) ) ;
#37346=EDGE_LOOP ( 'NONE', ( #18796, #16406, #26298, #30554 ) ) ;
#37351=CARTESIAN_POINT ( 'NONE',  ( 21.00000000000000000, 6.646953231504538984, -9.365624999385474325 ) ) ;
#37357=CARTESIAN_POINT ( 'NONE',  ( 34.38148213269554532, 5.407089921784862696, 167.1325768043071776 ) ) ;
#37365=CARTESIAN_POINT ( 'NONE',  ( 37.60414536301047406, -3.604726614523235284, 168.1493222201144704 ) ) ;
#37379=DIRECTION ( 'NONE',  ( 0.9961946980917462113, 0.000000000000000000, -0.08715574274765178209 ) ) ;
#37380=CARTESIAN_POINT ( 'NONE',  ( 31.22336862440664618, 6.928203230275506996, 166.8536380873862015 ) ) ;
#37381=CYLINDRICAL_SURFACE ( 'NONE', #8476, 6.000000000000001776 ) ;
#37382=( BOUNDED_CURVE ( )  B_SPLINE_CURVE ( 2, ( #3905, #30061, #4466, #27032, #26840, #36296, #35555 ),
 .UNSPECIFIED., .F., .F. ) 
 B_SPLINE_CURVE_WITH_KNOTS ( ( 3, 2, 2, 3 ),
 ( 0.6521739130434772713, 0.6594202898550713954, 0.6666666666666655194, 0.6739130434782596435 ),
 .UNSPECIFIED. ) 
 CURVE ( )  GEOMETRIC_REPRESENTATION_ITEM ( )  RATIONAL_B_SPLINE_CURVE ( ( 1.000000000000018430, 0.8660254037844202779, 1.000000000000000000, 0.8660254037844387076, 1.000000000000000000, 0.8660254037844612451, 0.9999999999999774625 ) ) 
 REPRESENTATION_ITEM ( '' )  );
#37395=CARTESIAN_POINT ( 'NONE',  ( 24.48144027668511669, 0.000000000000000000, 161.4299721732159014 ) ) ;
#37396=CARTESIAN_POINT ( 'NONE',  ( 18.12178482187499640, 4.985214923628404904, -1.228124999385488136 ) ) ;
#37400=ORIENTED_EDGE ( 'NONE', *, *, #8012, .T. ) ;
#37402=CARTESIAN_POINT ( 'NONE',  ( 18.00000000000000000, 5.196152422706630247, -7.218749998770951137 ) ) ;
#37403=CARTESIAN_POINT ( 'NONE',  ( 26.75643035624999655, 3.323476615752271268, -1.678124999385453897 ) ) ;
#37412=CARTESIAN_POINT ( 'NONE',  ( 24.78536444607796341, 0.000000000000000000, 162.1091930777120069 ) ) ;
#37416=CARTESIAN_POINT ( 'NONE',  ( 26.75643035624999655, -3.323476615752267271, -5.015624999385472904 ) ) ;
#37426=CARTESIAN_POINT ( 'NONE',  ( 27.63220001923324176, -5.407089921784865361, 161.6248569630975283 ) ) ;
#37436=CARTESIAN_POINT ( 'NONE',  ( 31.06648828746087787, 6.928203230275506996, 165.0604876308210578 ) ) ;
#37440=CARTESIAN_POINT ( 'NONE',  ( 15.00000000000000000, 3.464101615137752166, -4.987500000000014921 ) ) ;
#37442=CARTESIAN_POINT ( 'NONE',  ( 36.97498984505087805, 7.646167579472024665E-16, 160.9580417432647153 ) ) ;
#37444=CARTESIAN_POINT ( 'NONE',  ( 29.54925771143595981, 5.908847357411728396, 159.6727445521698883 ) ) ;
#37450=CARTESIAN_POINT ( 'NONE',  ( 27.96678062107526941, -5.196152422706638241, 164.0518066177726553 ) ) ;
#37454=DIRECTION ( 'NONE',  ( 0.08715574274765143514, 0.000000000000000000, 0.9961946980917462113 ) ) ;
#37458=CARTESIAN_POINT ( 'NONE',  ( 33.81932759197320593, -5.407089921784861808, 160.7071210016154055 ) ) ;
#37469=CARTESIAN_POINT ( 'NONE',  ( 28.28586808984062628, 5.407089921784862696, 169.0963171987856128 ) ) ;
#37471=CARTESIAN_POINT ( 'NONE',  ( 21.00000000000000000, -6.928203230275506996, -2.981249998770937992 ) ) ;
#37479=ORIENTED_EDGE ( 'NONE', *, *, #9772, .F. ) ;
#37480=CARTESIAN_POINT ( 'NONE',  ( 27.63710252976279591, -5.407089921784859143, 161.6808929148651828 ) ) ;
#37481=CARTESIAN_POINT ( 'NONE',  ( 21.00000000000000000, -6.646953231504538984, -6.778124999385457983 ) ) ;
#37483=CARTESIAN_POINT ( 'NONE',  ( 31.23562490067698150, 7.209453229046482114, 166.9937279661931768 ) ) ;
#37484=CARTESIAN_POINT ( 'NONE',  ( 34.08121910445329661, 5.196152422706637353, 165.0978788107812818 ) ) ;
#37485=CARTESIAN_POINT ( 'NONE',  ( 15.00000000000000000, 0.000000000000000000, 0.000000000000000000 ) ) ;
#37490=VERTEX_POINT ( 'NONE', #7694 ) ;
#37496=CARTESIAN_POINT ( 'NONE',  ( 26.75643035624999655, 3.323476615752271712, -2.690624999385500260 ) ) ;
#37522=COLOUR_RGB('Light Blue',0.38,0.62,0.78);
#37523=FILL_AREA_STYLE_COLOUR('',#37522);
#37524=FILL_AREA_STYLE('',(#37523));
#37525=SURFACE_STYLE_FILL_AREA(#37524);
#37526=SURFACE_SIDE_STYLE('',(#37525));
#37527=SURFACE_STYLE_USAGE(.BOTH.,#37526);
#37528=PRESENTATION_STYLE_ASSIGNMENT((#37527));
ENDSEC;
END-ISO-10303-21;
